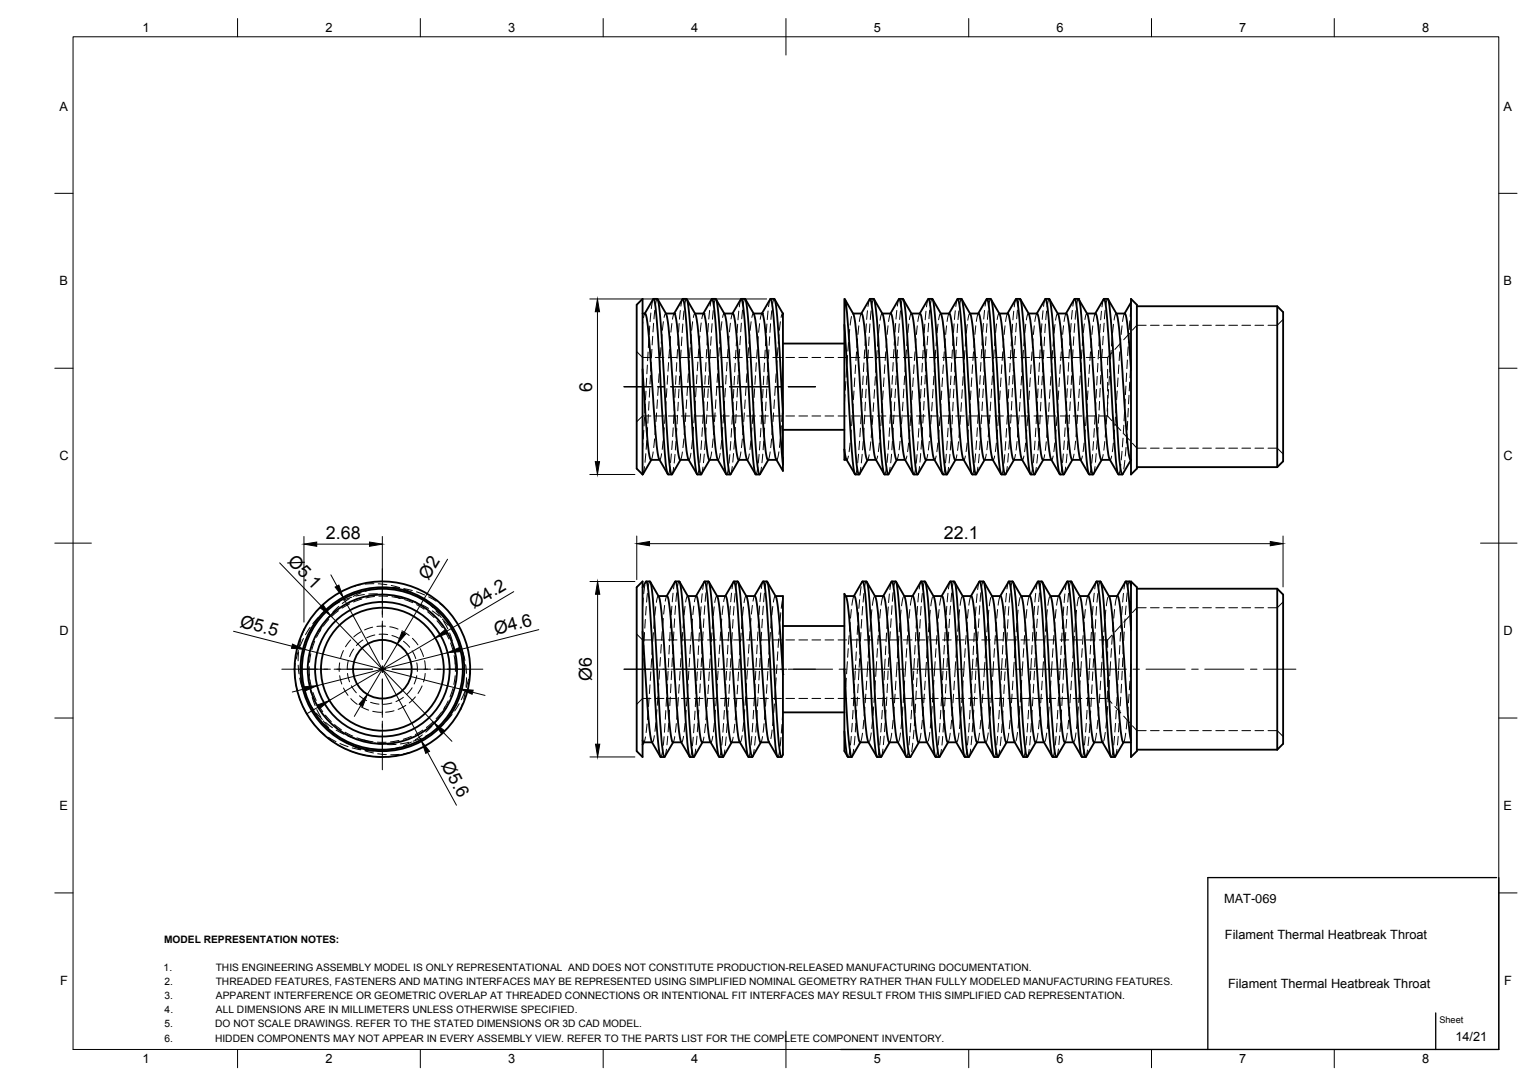
ISO-10303-21;
HEADER;
/* Generated by software containing ST-Developer
 * from STEP Tools, Inc. (www.steptools.com) 
 */

FILE_DESCRIPTION(
/* description */ ('CAx-IF Rec.Pracs.---Representation and Presentation of Product Manufa
cturing Information (PMI)---4.0---2014-10-13'),
/* implementation_level */ '2;1');

FILE_NAME(
/* name */ 'Filament Thermal Heatbreak Throat.step',
/* time_stamp */ '2026-10-24T15:08:39-07:00',
/* author */ (''),
/* organization */ (''),
/* preprocessor_version */ 'ST-DEVELOPER v20.2',
/* originating_system */ 'Autodesk Translation Framework v15.17.0.0',
/* authorisation */ '');

FILE_SCHEMA (('AP242_MANAGED_MODEL_BASED_3D_ENGINEERING_MIM_LF { 1 0 10303 442 2 1 4 }'));
ENDSEC;

DATA;
#10=MECHANICAL_DESIGN_GEOMETRIC_PRESENTATION_REPRESENTATION('',(#831),#50081);
#106=B_SPLINE_SURFACE_WITH_KNOTS('',3,3,((#39360,#39361,#39362,#39363,#39364,
#39365,#39366,#39367,#39368,#39369,#39370,#39371,#39372,#39373,#39374,#39375,
#39376,#39377,#39378,#39379,#39380,#39381,#39382,#39383,#39384,#39385,#39386,
#39387,#39388,#39389,#39390,#39391,#39392,#39393,#39394,#39395,#39396,#39397,
#39398,#39399,#39400,#39401,#39402,#39403,#39404,#39405,#39406,#39407,#39408,
#39409,#39410,#39411,#39412,#39413,#39414,#39415,#39416,#39417,#39418,#39419,
#39420,#39421,#39422,#39423,#39424,#39425,#39426),(#39427,#39428,#39429,
#39430,#39431,#39432,#39433,#39434,#39435,#39436,#39437,#39438,#39439,#39440,
#39441,#39442,#39443,#39444,#39445,#39446,#39447,#39448,#39449,#39450,#39451,
#39452,#39453,#39454,#39455,#39456,#39457,#39458,#39459,#39460,#39461,#39462,
#39463,#39464,#39465,#39466,#39467,#39468,#39469,#39470,#39471,#39472,#39473,
#39474,#39475,#39476,#39477,#39478,#39479,#39480,#39481,#39482,#39483,#39484,
#39485,#39486,#39487,#39488,#39489,#39490,#39491,#39492,#39493),(#39494,
#39495,#39496,#39497,#39498,#39499,#39500,#39501,#39502,#39503,#39504,#39505,
#39506,#39507,#39508,#39509,#39510,#39511,#39512,#39513,#39514,#39515,#39516,
#39517,#39518,#39519,#39520,#39521,#39522,#39523,#39524,#39525,#39526,#39527,
#39528,#39529,#39530,#39531,#39532,#39533,#39534,#39535,#39536,#39537,#39538,
#39539,#39540,#39541,#39542,#39543,#39544,#39545,#39546,#39547,#39548,#39549,
#39550,#39551,#39552,#39553,#39554,#39555,#39556,#39557,#39558,#39559,#39560),
(#39561,#39562,#39563,#39564,#39565,#39566,#39567,#39568,#39569,#39570,
#39571,#39572,#39573,#39574,#39575,#39576,#39577,#39578,#39579,#39580,#39581,
#39582,#39583,#39584,#39585,#39586,#39587,#39588,#39589,#39590,#39591,#39592,
#39593,#39594,#39595,#39596,#39597,#39598,#39599,#39600,#39601,#39602,#39603,
#39604,#39605,#39606,#39607,#39608,#39609,#39610,#39611,#39612,#39613,#39614,
#39615,#39616,#39617,#39618,#39619,#39620,#39621,#39622,#39623,#39624,#39625,
#39626,#39627)),.UNSPECIFIED.,.F.,.F.,.F.,(4,4),(4,1,1,1,1,1,1,1,1,1,1,
1,1,1,1,1,1,1,1,1,1,1,1,1,1,1,1,1,1,1,1,1,1,1,1,1,1,1,1,1,1,1,1,1,1,1,1,
1,1,1,1,1,1,1,1,1,1,1,1,1,1,1,1,1,4),(-0.000386239467008404,0.0586069165862638),
(7.06837814145609,8.05903683580502,9.04949020103305,10.0399435662611,11.0303969314891,
12.0208502967171,13.0113036619452,14.0017570271732,14.9922103924013,15.9826637576293,
16.9731171228573,17.9635704880854,18.9540238533134,19.9444772185414,20.9349305837695,
21.9253839489975,22.9158373142255,23.9062906794536,24.8967440446816,25.8871974099096,
26.8776507751377,27.8681041403657,28.8585575055937,29.8490108708218,30.8394642360498,
31.8299176012778,32.8203709665059,33.8108243317339,34.8012776969619,35.79173106219,
36.782184427418,37.772637792646,38.7630911578741,39.7535445231021,40.7439978883301,
41.7344512535582,42.7249046187862,43.7153579840142,44.7058113492423,45.6962647144703,
46.6867180796983,47.6771714449264,48.6676248101544,49.6580781753824,50.6485315406105,
51.6389849058385,52.6294382710665,53.6198916362946,54.6103450015226,55.6007983667506,
56.5912517319787,57.5817050972067,58.5721584624347,59.5626118276628,60.5530651928908,
61.5435185581188,62.5339719233469,63.5244252885749,64.5148786538029,65.505332019031,
66.495785384259,67.486238749487,68.4766921147151,69.4671454799431,70.4577594577278),
 .UNSPECIFIED.);
#107=B_SPLINE_SURFACE_WITH_KNOTS('',3,3,((#39674,#39675,#39676,#39677,#39678,
#39679,#39680,#39681,#39682,#39683,#39684,#39685,#39686,#39687,#39688,#39689,
#39690,#39691,#39692,#39693,#39694,#39695,#39696,#39697,#39698,#39699,#39700,
#39701,#39702,#39703,#39704,#39705,#39706,#39707,#39708,#39709,#39710,#39711,
#39712,#39713,#39714,#39715,#39716,#39717,#39718,#39719,#39720,#39721,#39722,
#39723,#39724,#39725,#39726,#39727,#39728,#39729,#39730,#39731,#39732,#39733,
#39734,#39735,#39736,#39737,#39738,#39739,#39740),(#39741,#39742,#39743,
#39744,#39745,#39746,#39747,#39748,#39749,#39750,#39751,#39752,#39753,#39754,
#39755,#39756,#39757,#39758,#39759,#39760,#39761,#39762,#39763,#39764,#39765,
#39766,#39767,#39768,#39769,#39770,#39771,#39772,#39773,#39774,#39775,#39776,
#39777,#39778,#39779,#39780,#39781,#39782,#39783,#39784,#39785,#39786,#39787,
#39788,#39789,#39790,#39791,#39792,#39793,#39794,#39795,#39796,#39797,#39798,
#39799,#39800,#39801,#39802,#39803,#39804,#39805,#39806,#39807),(#39808,
#39809,#39810,#39811,#39812,#39813,#39814,#39815,#39816,#39817,#39818,#39819,
#39820,#39821,#39822,#39823,#39824,#39825,#39826,#39827,#39828,#39829,#39830,
#39831,#39832,#39833,#39834,#39835,#39836,#39837,#39838,#39839,#39840,#39841,
#39842,#39843,#39844,#39845,#39846,#39847,#39848,#39849,#39850,#39851,#39852,
#39853,#39854,#39855,#39856,#39857,#39858,#39859,#39860,#39861,#39862,#39863,
#39864,#39865,#39866,#39867,#39868,#39869,#39870,#39871,#39872,#39873,#39874),
(#39875,#39876,#39877,#39878,#39879,#39880,#39881,#39882,#39883,#39884,
#39885,#39886,#39887,#39888,#39889,#39890,#39891,#39892,#39893,#39894,#39895,
#39896,#39897,#39898,#39899,#39900,#39901,#39902,#39903,#39904,#39905,#39906,
#39907,#39908,#39909,#39910,#39911,#39912,#39913,#39914,#39915,#39916,#39917,
#39918,#39919,#39920,#39921,#39922,#39923,#39924,#39925,#39926,#39927,#39928,
#39929,#39930,#39931,#39932,#39933,#39934,#39935,#39936,#39937,#39938,#39939,
#39940,#39941)),.UNSPECIFIED.,.F.,.F.,.F.,(4,4),(4,1,1,1,1,1,1,1,1,1,1,
1,1,1,1,1,1,1,1,1,1,1,1,1,1,1,1,1,1,1,1,1,1,1,1,1,1,1,1,1,1,1,1,1,1,1,1,
1,1,1,1,1,1,1,1,1,1,1,1,1,1,1,1,1,4),(-0.00577350269189626,0.0581188424251775),
(10.7523816656495,11.7430246153529,12.733477980581,13.723931345809,14.714384711037,
15.7048380762651,16.6952914414931,17.6857448067211,18.6761981719492,19.6666515371772,
20.6571049024052,21.6475582676333,22.6380116328613,23.6284649980893,24.6189183633174,
25.6093717285454,26.5998250937734,27.5902784590015,28.5807318242295,29.5711851894575,
30.5616385546856,31.5520919199136,32.5425452851416,33.5329986503697,34.5234520155977,
35.5139053808257,36.5043587460538,37.4948121112818,38.4852654765099,39.4757188417379,
40.4661722069659,41.4566255721939,42.447078937422,43.43753230265,44.4279856678781,
45.4184390331061,46.4088923983341,47.3993457635622,48.3897991287902,49.3802524940182,
50.3707058592463,51.3611592244743,52.3516125897023,53.3420659549304,54.3325193201584,
55.3229726853864,56.3134260506145,57.3038794158425,58.2943327810705,59.2847861462986,
60.2752395115266,61.2656928767546,62.2561462419827,63.2465996072107,64.2370529724387,
65.2275063376668,66.2179597028948,67.2084130681228,68.1988664333509,69.1893197985789,
70.1797731638069,71.170226529035,72.160679894263,73.151133259491,74.1417901888294),
 .UNSPECIFIED.);
#108=B_SPLINE_SURFACE_WITH_KNOTS('',3,3,((#40005,#40006,#40007,#40008,#40009,
#40010,#40011,#40012,#40013,#40014,#40015,#40016,#40017,#40018,#40019,#40020,
#40021,#40022,#40023,#40024,#40025,#40026,#40027,#40028,#40029,#40030,#40031,
#40032,#40033,#40034,#40035,#40036,#40037,#40038,#40039),(#40040,#40041,
#40042,#40043,#40044,#40045,#40046,#40047,#40048,#40049,#40050,#40051,#40052,
#40053,#40054,#40055,#40056,#40057,#40058,#40059,#40060,#40061,#40062,#40063,
#40064,#40065,#40066,#40067,#40068,#40069,#40070,#40071,#40072,#40073,#40074),
(#40075,#40076,#40077,#40078,#40079,#40080,#40081,#40082,#40083,#40084,
#40085,#40086,#40087,#40088,#40089,#40090,#40091,#40092,#40093,#40094,#40095,
#40096,#40097,#40098,#40099,#40100,#40101,#40102,#40103,#40104,#40105,#40106,
#40107,#40108,#40109),(#40110,#40111,#40112,#40113,#40114,#40115,#40116,
#40117,#40118,#40119,#40120,#40121,#40122,#40123,#40124,#40125,#40126,#40127,
#40128,#40129,#40130,#40131,#40132,#40133,#40134,#40135,#40136,#40137,#40138,
#40139,#40140,#40141,#40142,#40143,#40144)),.UNSPECIFIED.,.F.,.F.,.F.,(4,
4),(4,1,1,1,1,1,1,1,1,1,1,1,1,1,1,1,1,1,1,1,1,1,1,1,1,1,1,1,1,1,1,1,4),
(-0.000393287427394601,0.0585773552985969),(7.06836282084679,8.0677424967863,
9.06690152299556,10.0660605492048,11.0652195754141,12.0643786016233,13.0635376278326,
14.0626966540418,15.0618556802511,16.0610147064604,17.0601737326696,18.0593327588789,
19.0584917850881,20.0576508112974,21.0568098375066,22.0559688637159,23.0551278899252,
24.0542869161344,25.0534459423437,26.0526049685529,27.0517639947622,28.0509230209714,
29.0500820471807,30.04924107339,31.0484000995992,32.0475591258085,33.0467181520177,
34.045877178227,35.0450362044363,36.0441952306455,37.0433542568548,38.042513283064,
39.0418309313306),.UNSPECIFIED.);
#109=B_SPLINE_SURFACE_WITH_KNOTS('',3,3,((#40284,#40285,#40286,#40287,#40288,
#40289,#40290,#40291,#40292,#40293,#40294,#40295,#40296,#40297,#40298,#40299,
#40300,#40301,#40302,#40303,#40304,#40305,#40306,#40307,#40308,#40309,#40310,
#40311,#40312,#40313,#40314,#40315,#40316,#40317,#40318),(#40319,#40320,
#40321,#40322,#40323,#40324,#40325,#40326,#40327,#40328,#40329,#40330,#40331,
#40332,#40333,#40334,#40335,#40336,#40337,#40338,#40339,#40340,#40341,#40342,
#40343,#40344,#40345,#40346,#40347,#40348,#40349,#40350,#40351,#40352,#40353),
(#40354,#40355,#40356,#40357,#40358,#40359,#40360,#40361,#40362,#40363,
#40364,#40365,#40366,#40367,#40368,#40369,#40370,#40371,#40372,#40373,#40374,
#40375,#40376,#40377,#40378,#40379,#40380,#40381,#40382,#40383,#40384,#40385,
#40386,#40387,#40388),(#40389,#40390,#40391,#40392,#40393,#40394,#40395,
#40396,#40397,#40398,#40399,#40400,#40401,#40402,#40403,#40404,#40405,#40406,
#40407,#40408,#40409,#40410,#40411,#40412,#40413,#40414,#40415,#40416,#40417,
#40418,#40419,#40420,#40421,#40422,#40423)),.UNSPECIFIED.,.F.,.F.,.F.,(4,
4),(4,1,1,1,1,1,1,1,1,1,1,1,1,1,1,1,1,1,1,1,1,1,1,1,1,1,1,1,1,1,1,1,4),
(-0.000893816201826896,0.0581534486591829),(10.7523808111136,11.7517302763342,
12.7508893025435,13.7500483287527,14.749207354962,15.7483663811713,16.7475254073805,
17.7466844335898,18.745843459799,19.7450024860083,20.7441615122175,21.7433205384268,
22.742479564636,23.7416385908453,24.7407976170546,25.7399566432638,26.7391156694731,
27.7382746956823,28.7374337218916,29.7365927481009,30.7357517743101,31.7349108005194,
32.7340698267286,33.7332288529379,34.7323878791471,35.7315469053564,36.7307059315657,
37.7298649577749,38.7290239839842,39.7281830101934,40.7273420364027,41.7265010626119,
42.7258669660187),.UNSPECIFIED.);
#386=B_SPLINE_CURVE_WITH_KNOTS('',3,(#34790,#34791,#34792,#34793,#34794,
#34795,#34796,#34797,#34798,#34799,#34800,#34801,#34802,#34803,#34804,#34805,
#34806,#34807,#34808,#34809,#34810,#34811,#34812,#34813,#34814,#34815,#34816,
#34817,#34818,#34819,#34820,#34821,#34822,#34823,#34824,#34825,#34826,#34827,
#34828,#34829,#34830,#34831,#34832,#34833,#34834,#34835,#34836,#34837,#34838),
 .UNSPECIFIED.,.F.,.F.,(4,3,3,3,3,3,3,3,3,3,3,3,3,3,3,3,4),(0.,0.0927605595561279,
0.125,0.216051601199591,0.25,0.341388358155206,0.375,0.46637118185636,0.5,
0.591371181856193,0.625,0.716388358155103,0.75,0.841051601199441,0.875,
0.967760559556323,1.),.UNSPECIFIED.);
#387=B_SPLINE_CURVE_WITH_KNOTS('',3,(#34840,#34841,#34842,#34843,#34844,
#34845,#34846,#34847,#34848,#34849,#34850,#34851,#34852,#34853,#34854,#34855,
#34856,#34857,#34858,#34859,#34860,#34861,#34862,#34863,#34864,#34865,#34866,
#34867,#34868,#34869,#34870,#34871,#34872,#34873,#34874,#34875,#34876,#34877,
#34878,#34879,#34880,#34881,#34882,#34883,#34884,#34885,#34886,#34887,#34888,
#34889,#34890,#34891,#34892,#34893,#34894),.UNSPECIFIED.,.F.,.F.,(4,3,3,
3,3,3,3,3,3,3,3,3,3,3,3,3,3,3,4),(1.15710129956961E-6,0.0927580101727587,
0.125,0.215560207328814,0.25,0.343554436628594,0.375,0.4375,0.46875,0.5,
0.53125,0.5625,0.625,0.6875,0.75,0.835314126539692,0.875,0.952649745898871,
0.999999206802969),.UNSPECIFIED.);
#388=B_SPLINE_CURVE_WITH_KNOTS('',3,(#34896,#34897,#34898,#34899,#34900,
#34901,#34902,#34903,#34904,#34905,#34906,#34907,#34908,#34909,#34910,#34911,
#34912,#34913,#34914,#34915,#34916,#34917,#34918,#34919,#34920,#34921,#34922,
#34923,#34924,#34925,#34926,#34927,#34928,#34929,#34930,#34931,#34932,#34933,
#34934,#34935,#34936,#34937,#34938,#34939,#34940,#34941,#34942,#34943,#34944),
 .UNSPECIFIED.,.F.,.F.,(4,3,3,3,3,3,3,3,3,3,3,3,3,3,3,3,4),(0.,0.0927652271086669,
0.125,0.216056340442133,0.25,0.341393095875492,0.375,0.466375911195523,
0.5,0.59137591119598,0.625,0.716393095875431,0.75,0.841056340442169,0.875,
0.967765227108083,1.),.UNSPECIFIED.);
#389=B_SPLINE_CURVE_WITH_KNOTS('',3,(#34946,#34947,#34948,#34949,#34950,
#34951,#34952,#34953,#34954,#34955,#34956,#34957,#34958,#34959,#34960,#34961,
#34962,#34963,#34964,#34965,#34966,#34967,#34968,#34969,#34970,#34971,#34972,
#34973,#34974,#34975,#34976,#34977,#34978,#34979,#34980,#34981,#34982,#34983,
#34984,#34985,#34986,#34987,#34988,#34989,#34990,#34991,#34992,#34993,#34994),
 .UNSPECIFIED.,.F.,.F.,(4,3,3,3,3,3,3,3,3,3,3,3,3,3,3,3,4),(0.,0.0927588912582948,
0.125,0.216049907277145,0.25,0.34138666477614,0.375,0.466369491473306,0.5,
0.591369491472985,0.625,0.716386664776259,0.75,0.841049907277114,0.875,
0.967758891258586,1.),.UNSPECIFIED.);
#390=B_SPLINE_CURVE_WITH_KNOTS('',3,(#34996,#34997,#34998,#34999,#35000,
#35001,#35002,#35003,#35004,#35005,#35006,#35007,#35008,#35009,#35010,#35011,
#35012,#35013,#35014,#35015,#35016,#35017,#35018,#35019,#35020,#35021,#35022,
#35023,#35024,#35025,#35026,#35027,#35028,#35029,#35030,#35031,#35032,#35033,
#35034,#35035,#35036,#35037,#35038,#35039,#35040,#35041,#35042,#35043,#35044,
#35045,#35046,#35047,#35048,#35049,#35050,#35051,#35052,#35053,#35054,#35055,
#35056,#35057,#35058,#35059,#35060,#35061,#35062,#35063,#35064,#35065,#35066,
#35067,#35068,#35069,#35070,#35071),.UNSPECIFIED.,.F.,.F.,(4,3,3,3,3,3,
3,3,3,3,3,3,3,3,3,3,3,3,3,3,3,3,3,3,3,4),(1.15508471750028E-6,0.092144029884165,
0.125,0.216529255746127,0.25,0.3125,0.375,0.40625,0.4375,0.46875,0.484375,
0.4921875,0.5,0.5078125,0.515625,0.53125,0.5625,0.59375,0.625,0.6875,0.75,
0.8125,0.875,0.9375,0.995454104613646,0.999999596646375),.UNSPECIFIED.);
#391=B_SPLINE_CURVE_WITH_KNOTS('',3,(#35073,#35074,#35075,#35076,#35077,
#35078,#35079,#35080,#35081,#35082,#35083,#35084,#35085,#35086,#35087,#35088,
#35089,#35090,#35091,#35092,#35093,#35094,#35095,#35096,#35097,#35098,#35099,
#35100,#35101,#35102,#35103,#35104,#35105,#35106,#35107,#35108,#35109,#35110,
#35111,#35112,#35113,#35114,#35115,#35116,#35117,#35118,#35119,#35120,#35121),
 .UNSPECIFIED.,.F.,.F.,(4,3,3,3,3,3,3,3,3,3,3,3,3,3,3,3,4),(0.,0.0927687029302607,
0.125,0.216059869646637,0.25,0.341396623944995,0.375,0.466379433025891,
0.5,0.59137943302596,0.625,0.71639662394496,0.75,0.841059869646648,0.875,
0.967768702930745,1.),.UNSPECIFIED.);
#392=B_SPLINE_CURVE_WITH_KNOTS('',3,(#35123,#35124,#35125,#35126,#35127,
#35128,#35129,#35130,#35131,#35132,#35133,#35134,#35135,#35136,#35137,#35138,
#35139,#35140,#35141,#35142,#35143,#35144,#35145,#35146,#35147,#35148,#35149,
#35150,#35151,#35152,#35153,#35154,#35155,#35156,#35157,#35158,#35159,#35160,
#35161,#35162,#35163,#35164,#35165,#35166,#35167,#35168,#35169,#35170,#35171),
 .UNSPECIFIED.,.F.,.F.,(4,3,3,3,3,3,3,3,3,3,3,3,3,3,3,3,4),(0.,0.0927568833925016,
0.125,0.216047868569561,0.25,0.34138462672263,0.375,0.46636745702548,0.5,
0.59136745702557,0.625,0.716384626722753,0.75,0.841047868569713,0.875,0.967756883392973,
1.),.UNSPECIFIED.);
#393=B_SPLINE_CURVE_WITH_KNOTS('',3,(#35173,#35174,#35175,#35176,#35177,
#35178,#35179,#35180,#35181,#35182,#35183,#35184,#35185,#35186,#35187,#35188,
#35189,#35190,#35191,#35192,#35193,#35194,#35195,#35196,#35197,#35198,#35199,
#35200,#35201,#35202,#35203,#35204,#35205,#35206,#35207,#35208,#35209,#35210,
#35211,#35212,#35213,#35214,#35215,#35216,#35217,#35218,#35219,#35220,#35221),
 .UNSPECIFIED.,.F.,.F.,(4,3,3,3,3,3,3,3,3,3,3,3,3,3,3,3,4),(1.00511200959296E-6,
0.0927437682042961,0.125,0.216035219771111,0.25,0.341376986124011,0.375,
0.466313829040159,0.5,0.591406458509517,0.625,0.716377484365712,0.75,0.841045743313971,
0.875,0.967756443545387,0.99999978647056),.UNSPECIFIED.);
#394=B_SPLINE_CURVE_WITH_KNOTS('',3,(#35223,#35224,#35225,#35226,#35227,
#35228,#35229,#35230,#35231,#35232,#35233,#35234,#35235,#35236,#35237,#35238,
#35239,#35240,#35241,#35242,#35243,#35244,#35245,#35246,#35247,#35248,#35249,
#35250,#35251,#35252,#35253,#35254,#35255,#35256,#35257,#35258,#35259,#35260,
#35261,#35262,#35263,#35264,#35265,#35266,#35267,#35268,#35269,#35270,#35271),
 .UNSPECIFIED.,.F.,.F.,(4,3,3,3,3,3,3,3,3,3,3,3,3,3,3,3,4),(0.,0.0927720508247614,
0.125,0.216063268956037,0.25,0.341400022160318,0.375,0.466382825231913,
0.5,0.591382825232266,0.625,0.716400022160194,0.75,0.841063268956108,0.875,
0.967772050824302,1.),.UNSPECIFIED.);
#395=B_SPLINE_CURVE_WITH_KNOTS('',3,(#35277,#35278,#35279,#35280,#35281,
#35282,#35283,#35284,#35285,#35286,#35287,#35288,#35289,#35290,#35291,#35292,
#35293,#35294,#35295,#35296,#35297,#35298,#35299,#35300,#35301),
 .UNSPECIFIED.,.F.,.F.,(4,3,3,3,3,3,3,3,4),(0.,0.125,0.25,0.375,0.5,0.625,
0.75,0.875,0.999999474719706),.UNSPECIFIED.);
#396=B_SPLINE_CURVE_WITH_KNOTS('',3,(#35303,#35304,#35305,#35306,#35307,
#35308,#35309,#35310,#35311,#35312,#35313,#35314,#35315,#35316,#35317,#35318,
#35319,#35320,#35321,#35322,#35323,#35324,#35325,#35326,#35327,#35328,#35329,
#35330,#35331,#35332,#35333,#35334,#35335,#35336,#35337,#35338,#35339,#35340,
#35341,#35342,#35343,#35344,#35345,#35346,#35347,#35348,#35349,#35350,#35351),
 .UNSPECIFIED.,.F.,.F.,(4,3,3,3,3,3,3,3,3,3,3,3,3,3,3,3,4),(0.,0.092751628903762,
0.125,0.216042533365587,0.25,0.341379293228406,0.375,0.466362132969287,
0.5,0.591362132969264,0.625,0.716379293228501,0.75,0.841042533365549,0.875,
0.967751628903877,1.),.UNSPECIFIED.);
#397=B_SPLINE_CURVE_WITH_KNOTS('',3,(#35353,#35354,#35355,#35356,#35357,
#35358,#35359,#35360,#35361,#35362,#35363,#35364,#35365,#35366,#35367,#35368,
#35369,#35370,#35371,#35372,#35373,#35374,#35375,#35376,#35377,#35378,#35379,
#35380,#35381,#35382,#35383,#35384,#35385,#35386,#35387,#35388,#35389,#35390,
#35391,#35392,#35393,#35394,#35395,#35396,#35397,#35398,#35399,#35400,#35401),
 .UNSPECIFIED.,.F.,.F.,(4,3,3,3,3,3,3,3,3,3,3,3,3,3,3,3,4),(0.,0.0927733010189759,
0.125,0.216064538349619,0.25,0.341401291145062,0.375,0.4663840919732,0.5,
0.591384091973165,0.625,0.716401291144964,0.75,0.841064538349631,0.875,
0.967773301019603,1.),.UNSPECIFIED.);
#398=B_SPLINE_CURVE_WITH_KNOTS('',3,(#35403,#35404,#35405,#35406,#35407,
#35408,#35409,#35410,#35411,#35412,#35413,#35414,#35415,#35416,#35417,#35418,
#35419,#35420,#35421,#35422,#35423,#35424,#35425,#35426,#35427,#35428,#35429,
#35430,#35431,#35432,#35433,#35434,#35435,#35436,#35437,#35438,#35439,#35440,
#35441,#35442,#35443,#35444,#35445,#35446,#35447,#35448,#35449,#35450,#35451,
#35452,#35453,#35454),.UNSPECIFIED.,.F.,.F.,(4,2,2,2,2,2,2,2,2,2,2,2,2,
2,2,2,2,2,2,2,2,2,2,2,2,4),(0.,0.0553130156040213,0.0625,0.125,0.1875,0.25,
0.3125,0.375,0.40625,0.4375,0.46875,0.484375,0.4921875,0.5,0.5078125,0.515625,
0.53125,0.5625,0.59375,0.625,0.6875,0.75,0.841517211022419,0.875,0.967130863494855,
0.999999278904145),.UNSPECIFIED.);
#399=B_SPLINE_CURVE_WITH_KNOTS('',3,(#35456,#35457,#35458,#35459,#35460,
#35461,#35462,#35463,#35464,#35465,#35466,#35467,#35468,#35469,#35470,#35471,
#35472,#35473,#35474,#35475,#35476,#35477,#35478,#35479,#35480,#35481,#35482,
#35483,#35484,#35485,#35486,#35487,#35488,#35489,#35490,#35491,#35492,#35493,
#35494,#35495,#35496,#35497,#35498,#35499,#35500,#35501,#35502,#35503,#35504),
 .UNSPECIFIED.,.F.,.F.,(4,3,3,3,3,3,3,3,3,3,3,3,3,3,3,3,4),(0.,0.092754553141066,
0.125,0.21604550252371,0.25,0.341382261435592,0.375,0.466365095923449,0.5,
0.591365095923193,0.625,0.716382261435363,0.75,0.841045502523726,0.875,
0.96775455314112,1.),.UNSPECIFIED.);
#400=B_SPLINE_CURVE_WITH_KNOTS('',3,(#35506,#35507,#35508,#35509,#35510,
#35511,#35512,#35513,#35514,#35515,#35516,#35517,#35518,#35519,#35520,#35521,
#35522,#35523,#35524,#35525,#35526,#35527,#35528,#35529,#35530,#35531,#35532,
#35533,#35534,#35535,#35536,#35537,#35538,#35539,#35540,#35541,#35542,#35543,
#35544,#35545,#35546,#35547,#35548,#35549,#35550,#35551,#35552,#35553,#35554),
 .UNSPECIFIED.,.F.,.F.,(4,3,3,3,3,3,3,3,3,3,3,3,3,3,3,3,4),(0.,0.0927714769858617,
0.125,0.216062686304942,0.25,0.341399439696681,0.375,0.466382243798817,
0.5,0.591382243798365,0.625,0.716399439696732,0.75,0.841062686305149,0.875,
0.967771476985755,1.),.UNSPECIFIED.);
#401=B_SPLINE_CURVE_WITH_KNOTS('',3,(#35556,#35557,#35558,#35559,#35560,
#35561,#35562,#35563,#35564,#35565,#35566,#35567,#35568,#35569,#35570,#35571,
#35572,#35573,#35574,#35575,#35576,#35577,#35578,#35579,#35580,#35581,#35582,
#35583,#35584,#35585,#35586,#35587,#35588,#35589,#35590,#35591,#35592,#35593,
#35594,#35595,#35596,#35597,#35598,#35599,#35600,#35601,#35602,#35603,#35604,
#35605,#35606,#35607,#35608,#35609,#35610,#35611,#35612,#35613,#35614,#35615,
#35616,#35617,#35618,#35619,#35620,#35621,#35622,#35623,#35624,#35625,#35626,
#35627,#35628,#35629,#35630,#35631,#35632,#35633,#35634,#35635,#35636,#35637,
#35638,#35639,#35640,#35641,#35642,#35643),.UNSPECIFIED.,.F.,.F.,(4,3,3,
3,3,3,3,3,3,3,3,3,3,3,3,3,3,3,3,3,3,3,3,3,3,3,3,3,3,4),(1.05714741198223E-7,
0.0471016803099375,0.0625,0.114776485281687,0.125,0.183175405287037,0.1875,
0.25,0.3125,0.375,0.40625,0.4375,0.453125,0.46875,0.484375,0.4921875,0.5,
0.5078125,0.515625,0.53125,0.546875,0.5625,0.59375,0.625,0.6875,0.75,0.8125,
0.875,0.968959747574043,0.999999002444466),.UNSPECIFIED.);
#402=B_SPLINE_CURVE_WITH_KNOTS('',3,(#35645,#35646,#35647,#35648,#35649,
#35650,#35651,#35652,#35653,#35654,#35655,#35656,#35657,#35658,#35659,#35660,
#35661,#35662,#35663,#35664,#35665,#35666,#35667,#35668,#35669,#35670,#35671,
#35672,#35673,#35674,#35675,#35676,#35677,#35678,#35679,#35680,#35681,#35682,
#35683,#35684,#35685,#35686,#35687,#35688,#35689,#35690,#35691,#35692,#35693),
 .UNSPECIFIED.,.F.,.F.,(4,3,3,3,3,3,3,3,3,3,3,3,3,3,3,3,4),(0.,0.0927568305050716,
0.125,0.216047814869766,0.25,0.341384573040307,0.375,0.466367403437729,
0.5,0.591367403437667,0.625,0.716384573040161,0.75,0.841047814869804,0.875,
0.967756830505404,1.),.UNSPECIFIED.);
#403=B_SPLINE_CURVE_WITH_KNOTS('',3,(#35695,#35696,#35697,#35698,#35699,
#35700,#35701,#35702,#35703,#35704,#35705,#35706,#35707,#35708,#35709,#35710,
#35711,#35712,#35713,#35714,#35715,#35716,#35717,#35718,#35719,#35720,#35721,
#35722,#35723,#35724,#35725,#35726,#35727,#35728,#35729,#35730,#35731,#35732,
#35733,#35734,#35735,#35736,#35737,#35738,#35739,#35740,#35741,#35742,#35743),
 .UNSPECIFIED.,.F.,.F.,(4,3,3,3,3,3,3,3,3,3,3,3,3,3,3,3,4),(0.,0.0927687785918848,
0.125,0.21605994647008,0.25,0.341396700743647,0.375,0.466379509688856,0.5,
0.591379509688596,0.625,0.716396700743673,0.75,0.841059946470065,0.875,
0.967768778592018,1.),.UNSPECIFIED.);
#404=B_SPLINE_CURVE_WITH_KNOTS('',3,(#35745,#35746,#35747,#35748,#35749,
#35750,#35751,#35752,#35753,#35754,#35755,#35756,#35757,#35758,#35759,#35760,
#35761,#35762,#35763,#35764,#35765,#35766,#35767,#35768,#35769,#35770,#35771,
#35772,#35773,#35774,#35775,#35776,#35777,#35778),.UNSPECIFIED.,.F.,.F.,
(4,2,2,2,2,2,2,2,2,2,2,2,2,2,2,2,4),(6.2904793357381E-7,0.092754167897614,
0.125,0.216044766897767,0.25,0.341379705506234,0.375,0.466367644770845,
0.5,0.591380776467673,0.625,0.716346028360352,0.75,0.841038184239321,0.875,
0.967744550610455,0.999998988396429),.UNSPECIFIED.);
#405=B_SPLINE_CURVE_WITH_KNOTS('',3,(#35780,#35781,#35782,#35783),
 .UNSPECIFIED.,.F.,.F.,(4,4),(0.,0.999999235891784),.UNSPECIFIED.);
#406=B_SPLINE_CURVE_WITH_KNOTS('',3,(#35786,#35787,#35788,#35789,#35790,
#35791,#35792,#35793,#35794,#35795,#35796,#35797,#35798,#35799,#35800,#35801,
#35802,#35803,#35804,#35805,#35806,#35807,#35808,#35809,#35810,#35811,#35812,
#35813,#35814,#35815,#35816,#35817,#35818,#35819,#35820,#35821,#35822,#35823,
#35824,#35825,#35826,#35827,#35828,#35829,#35830,#35831,#35832,#35833,#35834),
 .UNSPECIFIED.,.F.,.F.,(4,3,3,3,3,3,3,3,3,3,3,3,3,3,3,3,4),(5.35367963709457E-13,
0.11846007821872,0.125,0.242079186084241,0.25,0.367390321915038,0.375,0.492346917375386,
0.5,0.617346917375406,0.625,0.742390321915024,0.75,0.86707918608421,0.875,
0.993460078218313,1.),.UNSPECIFIED.);
#407=B_SPLINE_CURVE_WITH_KNOTS('',3,(#35838,#35839,#35840,#35841,#35842,
#35843,#35844,#35845,#35846,#35847,#35848,#35849,#35850,#35851,#35852,#35853,
#35854,#35855,#35856,#35857,#35858,#35859,#35860,#35861,#35862,#35863,#35864,
#35865,#35866,#35867,#35868,#35869,#35870,#35871,#35872,#35873,#35874,#35875,
#35876,#35877,#35878,#35879,#35880,#35881,#35882,#35883,#35884,#35885,#35886),
 .UNSPECIFIED.,.F.,.F.,(4,3,3,3,3,3,3,3,3,3,3,3,3,3,3,3,4),(0.500496609805673,
0.50390625,0.5078125,0.515625,0.53125,0.546875,0.5625,0.591671105840508,
0.59375,0.625,0.6875,0.749287235495431,0.75,0.8125,0.875,0.907000590990823,
0.999998995230263),.UNSPECIFIED.);
#408=B_SPLINE_CURVE_WITH_KNOTS('',3,(#35888,#35889,#35890,#35891,#35892,
#35893,#35894,#35895,#35896,#35897,#35898,#35899,#35900,#35901,#35902,#35903,
#35904,#35905,#35906,#35907,#35908,#35909,#35910,#35911,#35912,#35913,#35914,
#35915,#35916,#35917,#35918,#35919,#35920,#35921,#35922,#35923,#35924,#35925,
#35926,#35927,#35928,#35929,#35930,#35931,#35932,#35933,#35934,#35935,#35936,
#35937,#35938,#35939,#35940,#35941,#35942,#35943,#35944,#35945,#35946,#35947,
#35948,#35949,#35950,#35951,#35952,#35953,#35954,#35955,#35956,#35957,#35958,
#35959,#35960,#35961,#35962,#35963,#35964,#35965,#35966,#35967,#35968,#35969,
#35970,#35971,#35972,#35973,#35974,#35975,#35976,#35977,#35978,#35979,#35980,
#35981,#35982,#35983,#35984,#35985,#35986,#35987,#35988,#35989,#35990,#35991,
#35992,#35993,#35994,#35995,#35996,#35997,#35998,#35999,#36000,#36001,#36002,
#36003,#36004,#36005,#36006,#36007,#36008,#36009,#36010,#36011,#36012,#36013,
#36014,#36015,#36016,#36017,#36018,#36019,#36020,#36021,#36022,#36023,#36024,
#36025,#36026,#36027,#36028,#36029,#36030,#36031,#36032,#36033,#36034,#36035,
#36036,#36037,#36038,#36039,#36040,#36041,#36042,#36043,#36044,#36045,#36046,
#36047,#36048,#36049,#36050,#36051,#36052,#36053,#36054,#36055,#36056,#36057,
#36058,#36059,#36060,#36061,#36062,#36063,#36064,#36065,#36066,#36067,#36068,
#36069,#36070,#36071,#36072,#36073,#36074,#36075,#36076,#36077,#36078,#36079,
#36080,#36081,#36082,#36083,#36084,#36085,#36086,#36087,#36088,#36089,#36090,
#36091,#36092,#36093,#36094,#36095,#36096,#36097,#36098,#36099,#36100,#36101,
#36102,#36103,#36104,#36105,#36106,#36107,#36108,#36109,#36110,#36111,#36112,
#36113,#36114,#36115,#36116,#36117,#36118,#36119,#36120,#36121,#36122,#36123,
#36124,#36125,#36126,#36127,#36128,#36129,#36130,#36131,#36132,#36133,#36134,
#36135,#36136,#36137,#36138,#36139,#36140,#36141,#36142,#36143,#36144,#36145,
#36146,#36147,#36148,#36149,#36150,#36151,#36152,#36153,#36154,#36155,#36156,
#36157,#36158,#36159,#36160,#36161,#36162,#36163,#36164,#36165,#36166,#36167,
#36168,#36169,#36170,#36171,#36172,#36173,#36174,#36175,#36176,#36177,#36178,
#36179,#36180,#36181,#36182,#36183,#36184,#36185,#36186,#36187,#36188,#36189,
#36190,#36191,#36192,#36193,#36194,#36195,#36196,#36197,#36198,#36199,#36200,
#36201,#36202,#36203,#36204,#36205,#36206,#36207,#36208,#36209,#36210,#36211,
#36212,#36213,#36214,#36215,#36216,#36217,#36218,#36219,#36220,#36221,#36222,
#36223,#36224,#36225,#36226,#36227,#36228,#36229,#36230,#36231,#36232,#36233,
#36234,#36235,#36236,#36237,#36238,#36239,#36240,#36241,#36242,#36243,#36244,
#36245,#36246,#36247,#36248,#36249,#36250,#36251,#36252,#36253,#36254,#36255,
#36256,#36257,#36258,#36259,#36260,#36261,#36262,#36263,#36264,#36265,#36266,
#36267,#36268,#36269,#36270,#36271,#36272,#36273,#36274,#36275,#36276,#36277,
#36278,#36279,#36280,#36281,#36282,#36283,#36284,#36285,#36286,#36287,#36288,
#36289,#36290,#36291,#36292,#36293,#36294,#36295,#36296,#36297,#36298,#36299,
#36300,#36301,#36302,#36303,#36304,#36305,#36306,#36307,#36308,#36309,#36310,
#36311,#36312,#36313,#36314,#36315,#36316,#36317,#36318,#36319,#36320,#36321,
#36322,#36323,#36324,#36325,#36326,#36327,#36328,#36329,#36330,#36331,#36332,
#36333,#36334,#36335,#36336,#36337,#36338,#36339,#36340,#36341,#36342,#36343,
#36344,#36345,#36346,#36347,#36348,#36349,#36350,#36351,#36352,#36353,#36354,
#36355,#36356,#36357,#36358,#36359,#36360,#36361,#36362,#36363,#36364,#36365,
#36366,#36367,#36368,#36369,#36370,#36371,#36372,#36373,#36374,#36375,#36376,
#36377,#36378,#36379,#36380,#36381,#36382,#36383,#36384,#36385,#36386,#36387,
#36388,#36389,#36390,#36391,#36392,#36393,#36394,#36395,#36396,#36397,#36398,
#36399,#36400,#36401,#36402,#36403,#36404,#36405,#36406,#36407,#36408,#36409,
#36410,#36411,#36412,#36413,#36414,#36415,#36416,#36417,#36418,#36419,#36420,
#36421,#36422,#36423,#36424,#36425,#36426,#36427,#36428,#36429,#36430,#36431,
#36432,#36433,#36434,#36435,#36436,#36437,#36438,#36439,#36440,#36441,#36442,
#36443,#36444,#36445,#36446,#36447,#36448,#36449,#36450,#36451,#36452,#36453,
#36454,#36455,#36456,#36457,#36458,#36459,#36460,#36461,#36462,#36463,#36464,
#36465,#36466,#36467,#36468,#36469,#36470,#36471,#36472,#36473,#36474,#36475,
#36476,#36477,#36478,#36479,#36480,#36481,#36482,#36483,#36484,#36485,#36486,
#36487,#36488,#36489,#36490,#36491,#36492,#36493,#36494,#36495,#36496,#36497,
#36498,#36499,#36500,#36501,#36502,#36503,#36504,#36505,#36506,#36507,#36508,
#36509,#36510,#36511,#36512,#36513,#36514,#36515,#36516,#36517,#36518,#36519,
#36520,#36521,#36522,#36523,#36524,#36525,#36526,#36527,#36528,#36529,#36530,
#36531,#36532,#36533,#36534,#36535,#36536,#36537,#36538,#36539,#36540,#36541,
#36542,#36543,#36544,#36545,#36546,#36547,#36548,#36549,#36550,#36551,#36552,
#36553,#36554,#36555,#36556,#36557,#36558,#36559,#36560,#36561,#36562,#36563,
#36564,#36565,#36566,#36567,#36568,#36569,#36570,#36571,#36572,#36573,#36574,
#36575,#36576,#36577,#36578,#36579,#36580,#36581,#36582,#36583,#36584,#36585,
#36586,#36587,#36588,#36589,#36590,#36591,#36592,#36593,#36594,#36595,#36596,
#36597,#36598,#36599,#36600,#36601,#36602,#36603,#36604,#36605,#36606,#36607,
#36608,#36609,#36610,#36611,#36612,#36613,#36614,#36615,#36616,#36617,#36618,
#36619,#36620,#36621,#36622,#36623,#36624,#36625,#36626,#36627,#36628,#36629,
#36630,#36631,#36632,#36633,#36634,#36635,#36636,#36637,#36638,#36639,#36640,
#36641,#36642,#36643,#36644,#36645,#36646,#36647,#36648,#36649,#36650,#36651,
#36652,#36653,#36654,#36655,#36656,#36657,#36658,#36659,#36660,#36661,#36662,
#36663,#36664,#36665,#36666,#36667,#36668,#36669,#36670,#36671,#36672,#36673,
#36674,#36675,#36676,#36677,#36678,#36679,#36680,#36681,#36682,#36683,#36684,
#36685,#36686,#36687,#36688,#36689,#36690,#36691,#36692,#36693,#36694,#36695,
#36696,#36697,#36698,#36699,#36700,#36701,#36702,#36703,#36704,#36705,#36706,
#36707,#36708,#36709,#36710,#36711,#36712,#36713,#36714,#36715,#36716,#36717,
#36718,#36719,#36720,#36721,#36722,#36723,#36724,#36725,#36726,#36727,#36728,
#36729,#36730,#36731,#36732,#36733,#36734,#36735,#36736,#36737,#36738,#36739,
#36740,#36741,#36742,#36743,#36744,#36745,#36746,#36747,#36748,#36749,#36750,
#36751,#36752,#36753,#36754,#36755,#36756,#36757,#36758,#36759,#36760,#36761,
#36762,#36763,#36764,#36765,#36766,#36767,#36768,#36769,#36770,#36771,#36772,
#36773,#36774,#36775,#36776,#36777,#36778,#36779,#36780,#36781,#36782,#36783,
#36784,#36785,#36786,#36787,#36788,#36789,#36790,#36791,#36792,#36793,#36794,
#36795,#36796,#36797,#36798,#36799,#36800,#36801,#36802,#36803,#36804,#36805,
#36806,#36807,#36808,#36809,#36810,#36811,#36812,#36813,#36814,#36815,#36816,
#36817,#36818,#36819,#36820,#36821,#36822,#36823,#36824,#36825,#36826,#36827,
#36828,#36829,#36830,#36831,#36832,#36833),.UNSPECIFIED.,.F.,.F.,(4,2,2,
2,2,2,2,2,2,2,2,2,2,2,2,2,2,2,2,2,2,2,2,2,2,2,2,2,2,2,2,2,2,2,2,2,2,2,2,
2,2,2,2,2,2,2,2,2,2,2,2,2,2,2,2,2,2,2,2,2,2,2,2,2,2,2,2,2,2,2,2,2,2,2,2,
2,2,2,2,2,2,2,2,2,2,2,2,2,2,2,2,2,2,2,2,2,2,2,2,2,2,2,2,2,2,2,2,2,2,2,2,
2,2,2,2,2,2,2,2,2,2,2,2,2,2,2,2,2,2,2,2,2,2,2,2,2,2,2,2,2,2,2,2,2,2,2,2,
2,2,2,2,2,2,2,2,2,2,2,2,2,2,2,2,2,2,2,2,2,2,2,2,2,2,2,2,2,2,2,2,2,2,2,2,
2,2,2,2,2,2,2,2,2,2,2,2,2,2,2,2,2,2,2,2,2,2,2,2,2,2,2,2,2,2,2,2,2,2,2,2,
2,2,2,2,2,2,2,2,2,2,2,2,2,2,2,2,2,2,2,2,2,2,2,2,2,2,2,2,2,2,2,2,2,2,2,2,
2,2,2,2,2,2,2,2,2,2,2,2,2,2,2,2,2,2,2,2,2,2,2,2,2,2,2,2,2,2,2,2,2,2,2,2,
2,2,2,2,2,2,2,2,2,2,2,2,2,2,2,2,2,2,2,2,2,2,2,2,2,2,2,2,2,2,2,2,2,2,2,2,
2,2,2,2,2,2,2,2,2,2,2,2,2,2,2,2,2,2,2,2,2,2,2,2,2,2,2,2,2,2,2,2,2,2,2,2,
2,2,2,2,2,2,2,2,2,2,2,2,2,2,2,2,2,2,2,2,2,2,2,2,2,2,2,2,2,2,2,2,2,2,2,2,
2,2,2,2,2,2,2,2,2,2,2,2,2,2,2,2,2,2,2,2,2,2,2,2,2,2,2,2,2,2,2,2,2,2,2,2,
2,2,2,2,2,2,2,2,2,2,2,2,2,2,2,2,2,2,2,2,2,2,2,2,2,2,2,2,2,2,2,2,2,2,2,2,
2,4),(0.000313237606796583,0.0732396125606311,0.107388601669689,0.116229997177897,
0.120739200951735,0.12448068829046,0.12932232799047,0.140221656971463,0.197481902428677,
0.242183482957304,0.258897773384315,0.267128547630496,0.273754482371197,
0.281405825657101,0.294762578788611,0.359832446620594,0.392697716411196,
0.410524918994634,0.416397219067249,0.420282279646255,0.423842780221686,
0.43003701160593,0.449122813102218,0.499312016373005,0.532450329898909,
0.554251024099348,0.563329965988381,0.570055283822999,0.577253748747926,
0.588794905730077,0.63783386640416,0.68555064429509,0.700318391868383,0.71074492774884,
0.715554302770943,0.719289105967843,0.723890692170196,0.733204015963814,
0.775297264573541,0.813397616482522,0.836829411115005,0.854004311242021,
0.862319189947006,0.868890720456341,0.876460021720684,0.889436588905798,
0.958064649980759,0.988901173792772,1.00605964200919,1.01185486548237,1.01572483607133,
1.01981038743091,1.02662506481103,1.05294308186016,1.11603960015384,1.13681639290964,
1.15255038391308,1.16059722623153,1.16657003890367,1.17412248481406,1.18702187013861,
1.26634207907997,1.29860430761864,1.30722407958094,1.31168903283532,1.31543564929409,
1.32033674769295,1.3315838632717,1.38851310549199,1.43301151510683,1.44974680322203,
1.45798167437105,1.46460815319793,1.47225708342722,1.48560161688953,1.5508096408345,
1.58359577756807,1.60139783967576,1.60726747808697,1.61115213976924,1.61471343822002,
1.62091124413417,1.64002901256489,1.69019703923327,1.72332762695399,1.74512535184184,
1.75420411351427,1.76092964789903,1.76812867093258,1.77967145331808,1.82873709616104,
1.87643479990973,1.89120007939844,1.90162546861717,1.906434770132,1.9101697274484,
1.91477176451421,1.92408679796526,1.96636127139429,2.00482306070261,2.02795782992859,
2.0449757045374,2.05326230394008,2.05989243997341,2.06750403665759,2.08067525344837,
2.14761187164537,2.17939332316874,2.19686781230856,2.20270002240954,2.20657731262491,
2.21014682013202,2.21638708153345,2.23591442338624,2.28577745846129,2.33125256327586,
2.3448634669727,2.35249097721753,2.35911945320565,2.36738364623431,2.38048505743541,
2.45126394470639,2.491824698676,2.4990749260843,2.50325459238726,2.50703244418594,
2.51165892580978,2.5230138751059,2.57957652125262,2.62385667981512,2.640608277974,
2.64884637960265,2.65547334481351,2.66312050416494,2.67645581165643,2.74177291493049,
2.77449742393239,2.7922799505251,2.79814754898393,2.80203192776873,2.80559387940277,
2.81179453066218,2.83093749953759,2.88108952277184,2.91421444333614,2.93601008099111,
2.94508878799329,2.95181455092315,2.95901406896798,2.97055820458558,3.01964431923071,
3.06732837603487,3.08209198747141,3.09251664138888,3.09732594073853,3.10106105597637,
3.1056634855733,3.11497990222459,3.15743985639091,3.21906433038732,3.23596923937728,
3.24423525632709,3.25080307478489,3.25840680359813,3.2715414761115,3.33881303289814,
3.37040526765403,3.38781716509415,3.39364215558881,3.39751804612596,3.40108919541907,
3.40733786232631,3.426948013979,3.48278666763428,3.51842522126189,3.53429071536459,
3.54236291286626,3.5483383589686,3.55587295299742,3.56868876036549,3.64839732381433,
3.68047143337749,3.68906884053197,3.6935294641211,3.69727691731241,3.70218474989,
3.71347069177186,3.77036733262433,3.81484680103362,3.83158489220578,3.83982060803806,
3.84644753088318,3.85409671343685,3.86744100221539,3.93266508916591,3.96544623029879,
3.98324714544429,3.98911689971542,3.99300175767898,3.99656333766215,4.0027618249125,
4.02188353105887,4.07205271143324,4.10518460928008,4.12698337883407,4.13606266588215,
4.14278861918699,4.14998811824146,4.16153172542411,4.21060248968077,4.25830151837033,
4.2730674850971,4.28349340724766,4.28830299066872,4.29203818429792,4.29664053409124,
4.30595626291475,4.34934748303688,4.39619782041856,4.41434929080584,4.42857812647288,
4.43633085160234,4.4429505060573,4.45105416420926,4.46359846997177,4.52012220950349,
4.55871685980115,4.57197906541737,4.58161223716024,4.58627531352348,4.5896388918647,
4.59418922081277,4.6032378874983,4.65583263761798,4.69656653463468,4.72135568666745,
4.730856601774,4.73758480567342,4.74462888557875,4.75541960666407,4.79288568239407,
4.82885445160377,4.87344626915557,4.88080474789728,4.88500753632564,4.88881892169032,
4.89429083248362,4.90891007740531,4.93287264334698,5.01162740766663,5.02465998817305,
5.03224150521685,5.03881164645255,5.04710891455437,5.06418654928975,5.08743200694948,
5.12585309495423,5.16790924677788,5.17722081086339,5.18182206712108,5.18555689260041,
5.19036670092958,5.20079548702653,5.21556888747791,5.26331057623244,5.31236987823311,
5.32391216753674,5.33111087790344,5.33783609047363,5.34691438697375,5.36871160436141,
5.40183944885928,5.45201633410622,5.47107788044713,5.47726931209096,5.48082925358337,
5.48471473812841,5.49058942437643,5.50843711943276,5.54136693322142,5.60638140494845,
5.6197470670641,5.62740026155646,5.63402591022171,5.64225388314361,5.65895372302928,
5.70370953468402,5.76105341546906,5.77079415343036,5.77555639304346,5.7793664111699,
5.78347665201096,5.79040604229506,5.82198915488222,5.8857049079595,5.91128857237193,
5.9211610784852,5.92733794405061,5.93417624848413,5.94391888997028,5.97061846915713,
6.01703809091761,6.06096967345059,6.0702767349235,6.07487690866175,6.07861148482227,
6.08342177761782,6.09385448693531,6.10863590921031,6.15643602560443,6.20541939886094,
6.21695774531404,6.22415527180339,6.23088023313038,6.23995951770358,6.261766258068,
6.29491770242867,6.34515755983286,6.36412883642266,6.37031032870974,6.3738681807214,
6.37775507522321,6.38363788156199,6.40156027295113,6.43472527589361,6.49934039243712,
6.51273957205739,6.52039961020333,6.52702412278388,6.53524154289608,6.55188625378585,
6.5967321111915,6.65408992772509,6.66381299538236,6.66857090801069,6.67237964758556,
6.67649143080277,6.68342886648739,6.71518648574016,6.77978011830595,6.80455227971896,
6.81430962319356,6.82108212878374,6.82805754263332,6.83851346682056,6.87195972478911,
6.95215361079866,6.96269806089745,6.96752838705944,6.97126383418314,6.97584690258443,
6.98506573626334,7.02263603588288,7.09433868882286,7.10799292718832,7.11570737876551,
7.12232755374372,7.13047392861467,7.14673772581042,7.20925409112281,7.25175036210626,
7.26106350359465,7.26566474748929,7.26939912698676,7.27420780311051,7.28463214639486,
7.29939754904456,7.34709095519899,7.39619443290078,7.40773763475398,7.4149359919494,
7.42166025661953,7.43073631439035,7.4525229928785,7.48562823741736,7.53575129037795,
7.55487486475011,7.56107238851728,7.56463323392608,7.56851706622811,7.57438498142335,
7.59217665456648,7.62493481732375,7.69022330462129,7.70356180776332,7.71120861885677,
7.71783400362131,7.72606848306152,7.74280685165591,7.78714839928332,7.84382330403291,
7.85529557183305,7.86023376188207,7.8639833645544,7.86842058678017,7.87690577738169,
7.88810374115488,7.91676560401724,7.98957914746058,8.00215087631491,8.00956315584407,
8.01622251652062,8.02482648592442,8.04365816094504,8.07033861727407,8.10460906787267,
8.14806363667771,8.15537705237786,8.15956945765984,8.16338350099015,8.16887609108397,
8.18365337250209,8.20801392577201,8.28573096649293,8.29897840424588,8.30660499365386,
8.31323133193775,8.32149111057444,8.33837102002009,8.38106655106261,8.4352194528517,
8.44928421307062,8.45482389939674,8.45860817415939,8.46276801406585,8.46993053964016,
8.50739522920647,8.56970187884935,8.59163513100119,8.60096217952688,8.60772586212575,
8.61483428769196,8.62594833814482,8.66832213642274,8.68365072489435,8.74111159240067,
8.7496274961707,8.75412329755277,8.75786472642003,8.76280357698595,8.77397110823675,
8.79020879126153,8.84939545791893,8.88566667308928,8.89658894894715,8.90365793660862,
8.91044347639736,8.91989866627855,8.94436484759657,8.98422036065577,9.03835238060195,
9.04708268240285,9.05162363084941,9.05532514558369,9.06018348337513,9.07088942244905,
9.08620626270874,9.13783286586151,9.18237623172095,9.19373048934184,9.20088857749546,
9.20762799411705,9.21680752646988,9.23930234293591,9.27409640251205,9.32864526177467,
9.34224801874259,9.34771243020849,9.35152134447465,9.35572449427036,9.36308997113074,
9.41097147200668,9.44274043488676),.UNSPECIFIED.);
#409=B_SPLINE_CURVE_WITH_KNOTS('',3,(#36835,#36836,#36837,#36838,#36839,
#36840,#36841,#36842,#36843,#36844,#36845,#36846,#36847,#36848,#36849,#36850,
#36851,#36852,#36853,#36854,#36855,#36856,#36857,#36858,#36859,#36860,#36861,
#36862,#36863,#36864,#36865,#36866,#36867,#36868,#36869,#36870,#36871,#36872,
#36873,#36874,#36875,#36876,#36877,#36878,#36879,#36880,#36881,#36882,#36883,
#36884,#36885,#36886,#36887,#36888,#36889,#36890,#36891,#36892,#36893,#36894,
#36895,#36896,#36897,#36898,#36899,#36900,#36901,#36902,#36903,#36904,#36905,
#36906,#36907,#36908,#36909,#36910,#36911,#36912,#36913,#36914,#36915,#36916,
#36917,#36918,#36919,#36920,#36921,#36922,#36923,#36924,#36925,#36926,#36927,
#36928,#36929,#36930,#36931,#36932,#36933,#36934,#36935,#36936,#36937,#36938,
#36939,#36940,#36941,#36942,#36943,#36944,#36945,#36946,#36947,#36948,#36949,
#36950,#36951,#36952,#36953,#36954,#36955,#36956,#36957,#36958,#36959,#36960,
#36961,#36962,#36963,#36964,#36965,#36966,#36967,#36968,#36969,#36970,#36971,
#36972,#36973,#36974,#36975,#36976,#36977,#36978,#36979,#36980,#36981,#36982,
#36983,#36984,#36985,#36986,#36987,#36988,#36989,#36990,#36991,#36992,#36993,
#36994,#36995,#36996,#36997,#36998,#36999,#37000,#37001,#37002,#37003,#37004,
#37005,#37006,#37007,#37008,#37009,#37010,#37011,#37012,#37013,#37014,#37015,
#37016,#37017,#37018,#37019,#37020,#37021,#37022,#37023,#37024,#37025,#37026,
#37027,#37028,#37029,#37030,#37031,#37032,#37033,#37034,#37035,#37036,#37037,
#37038,#37039,#37040,#37041,#37042,#37043,#37044,#37045,#37046,#37047,#37048,
#37049,#37050,#37051,#37052,#37053,#37054,#37055,#37056,#37057,#37058,#37059,
#37060,#37061,#37062,#37063,#37064,#37065,#37066,#37067,#37068,#37069,#37070,
#37071,#37072,#37073,#37074,#37075,#37076,#37077,#37078,#37079,#37080,#37081,
#37082,#37083,#37084,#37085,#37086,#37087,#37088,#37089,#37090,#37091,#37092,
#37093,#37094,#37095,#37096,#37097,#37098,#37099,#37100,#37101,#37102,#37103,
#37104,#37105,#37106,#37107,#37108,#37109,#37110,#37111,#37112,#37113,#37114,
#37115,#37116,#37117,#37118,#37119,#37120,#37121,#37122,#37123,#37124,#37125,
#37126,#37127,#37128,#37129,#37130,#37131,#37132,#37133,#37134,#37135,#37136,
#37137,#37138,#37139,#37140,#37141,#37142,#37143,#37144,#37145,#37146,#37147,
#37148,#37149,#37150,#37151,#37152,#37153,#37154,#37155,#37156,#37157,#37158,
#37159,#37160,#37161,#37162,#37163,#37164,#37165,#37166,#37167,#37168,#37169,
#37170,#37171,#37172,#37173,#37174,#37175,#37176,#37177,#37178,#37179,#37180,
#37181,#37182,#37183,#37184,#37185,#37186,#37187,#37188,#37189,#37190,#37191,
#37192,#37193,#37194,#37195,#37196,#37197,#37198,#37199,#37200,#37201,#37202,
#37203,#37204,#37205,#37206,#37207,#37208,#37209,#37210,#37211,#37212,#37213,
#37214,#37215,#37216,#37217,#37218,#37219,#37220,#37221,#37222,#37223,#37224),
 .UNSPECIFIED.,.F.,.F.,(4,2,2,2,2,2,2,2,2,2,2,2,2,2,2,2,2,2,2,2,2,2,2,2,
2,2,2,2,2,2,2,2,2,2,2,2,2,2,2,2,2,2,2,2,2,2,2,2,2,2,2,2,2,2,2,2,2,2,2,2,
2,2,2,2,2,2,2,2,2,2,2,2,2,2,2,2,2,2,2,2,2,2,2,2,2,2,2,2,2,2,2,2,2,2,2,2,
2,2,2,2,2,2,2,2,2,2,2,2,2,2,2,2,2,2,2,2,2,2,2,2,2,2,2,2,2,2,2,2,2,2,2,2,
2,2,2,2,2,2,2,2,2,2,2,2,2,2,2,2,2,2,2,2,2,2,2,2,2,2,2,2,2,2,2,2,2,2,2,2,
2,2,2,2,2,2,2,2,2,2,2,2,2,2,2,2,2,2,2,2,2,2,2,2,2,2,4),(9.99999999526152E-7,
0.02541508705979,0.0403509785521346,0.0478988957842898,0.0541473169418411,
0.0607715627350446,0.0689794030361682,0.0850231306095784,0.140555435079713,
0.173585934480102,0.188350097916006,0.198774669984789,0.203583572743684,
0.20731820680062,0.211919827642413,0.221233979609255,0.264646346264958,
0.311470042953097,0.329614886335042,0.343839280917871,0.35159037156107,
0.35820904340011,0.366312017366255,0.378856297343035,0.435269542521666,
0.473931972186144,0.49349270960845,0.499550744538113,0.503473421030138,
0.506997351234623,0.512999204789748,0.53040898313939,0.581879644126399,
0.623712128187474,0.640123710024594,0.648298060722711,0.654920127170653,
0.662613387749988,0.67616713643093,0.738608872800642,0.773101424473421,
0.791440449153294,0.797369422545081,0.80126564039814,0.804814062124252,
0.810945956436549,0.829461537871561,0.886330892904588,0.921781420161633,
0.937943429823994,0.946071029843745,0.952690622809616,0.960421006174729,
0.97414880871105,1.03185979384175,1.06958924070581,1.08268946443784,1.09223470828921,
1.09688056522918,1.10024265388201,1.1048070309001,1.11393025772448,1.1799559966417,
1.21189033405176,1.2331676438347,1.24216632496867,1.24887863916426,1.25610686702012,
1.26779453972329,1.31837403481817,1.35636457635536,1.38506419660503,1.39183807772474,
1.39591435594572,1.39974303726536,1.40552566248542,1.42124676978749,1.47406019861245,
1.50820862862716,1.53043596827541,1.5395775531375,1.54631192021341,1.55348559060862,
1.56491065125921,1.60926620515102,1.66090596941392,1.67622375644931,1.68693143540261,
1.69179065888691,1.69549305560627,1.70003539947624,1.70876887097193,1.76293424303464,
1.80280979026846,1.82728429692332,1.83674210724431,1.84352928172483,1.84976015883669,
1.8599462518553,1.88823141575172,1.94179659623945,1.97943655892693,1.98669149214734,
1.99087159173205,1.99469084996073,2.00021440726323,2.01522176968697,2.04016382138305,
2.1164765391538,2.13002112034464,2.13771127091191,2.14433177541148,2.15250559103361,
2.16892119780121,2.21093710449602,2.26274000132455,2.27967966095738,2.28562176463385,
2.28913403699085,2.29306869599499,2.29918716107689,2.31935976452665,2.36028657690867,
2.41367472917936,2.42626028226952,2.43437464521228,2.44099296215536,2.44873263999628,
2.46290364477065,2.48095745045831,2.52734101885416,2.57129836700053,2.58060409495587,
2.58520405916938,2.58893983523734,2.59375359411506,2.6041978076728,2.6190006463112,
2.66695430111742,2.71567951130462,2.72720795203295,2.73440477612739,2.7411329213571,
2.75022265791473,2.77208905832678,2.80537678018994,2.85596265538789,2.87447221987865,
2.88060315926801,2.88415128178029,2.88804330123993,2.89396506363409,2.91227355281239,
2.94667645633749,3.00935373112116,3.02289418062897,3.03057962783057,3.03719446225264,
3.04535893359252,3.06174596062229,3.10327548774194,3.15420939777526,3.17226518965298,
3.17834083402444,3.18187622467,3.18577996015993,3.19175249373992,3.21050493335888,
3.24635311542894,3.30691938175137,3.32057951640045,3.3282967358863,3.33491892847784,
3.34306739813751,3.35933488529976,3.42197603469795,3.46418131911456,3.47353803357934,
3.47815099013026,3.48189654725739,3.48672299886183,3.49718158689922,3.51200355480281,
3.56010114755446,3.60825547711487,3.6197700369559,3.62697430206707,3.63372116635705,
3.64285552699046,3.66494112643857,3.69871103664215,3.76234943713865,3.77115339485521,
3.77402045671866,3.77647229296193),.UNSPECIFIED.);
#410=B_SPLINE_CURVE_WITH_KNOTS('',3,(#37226,#37227,#37228,#37229,#37230,
#37231,#37232,#37233,#37234,#37235,#37236,#37237,#37238,#37239,#37240,#37241,
#37242,#37243,#37244,#37245,#37246,#37247,#37248,#37249,#37250,#37251,#37252,
#37253,#37254,#37255,#37256,#37257,#37258,#37259,#37260,#37261,#37262,#37263,
#37264,#37265,#37266,#37267,#37268,#37269,#37270,#37271,#37272,#37273,#37274,
#37275,#37276,#37277,#37278,#37279,#37280,#37281,#37282,#37283,#37284,#37285,
#37286,#37287,#37288,#37289,#37290,#37291,#37292,#37293,#37294,#37295,#37296,
#37297,#37298,#37299,#37300,#37301,#37302,#37303,#37304,#37305,#37306,#37307,
#37308,#37309,#37310,#37311,#37312,#37313,#37314,#37315,#37316,#37317,#37318,
#37319,#37320,#37321,#37322,#37323,#37324,#37325,#37326,#37327),
 .UNSPECIFIED.,.F.,.F.,(4,2,2,2,2,2,2,2,2,2,2,2,2,2,2,2,2,2,2,2,2,2,2,2,
2,2,2,2,2,2,2,2,2,2,2,2,2,2,2,2,2,2,2,2,2,2,2,2,2,2,4),(0.000274590634593237,
0.0025082762786118,0.00535069727310344,0.0116844857126863,0.0342991856608529,
0.0843016193333742,0.115297757508164,0.136139369508367,0.145022650646858,
0.151667283405926,0.158837468056138,0.170458820756428,0.221014938736121,
0.267413615605875,0.281958972332198,0.292254398082525,0.297016468905675,
0.300730962418017,0.305324808844561,0.314619905230995,0.357647295962238,
0.419422814912621,0.436370390294811,0.444655812784192,0.451299173082329,
0.458941834237123,0.472211170200764,0.516280100710487,0.546464638149321,
0.58483144266112,0.59212456635804,0.596333234407501,0.600256784222936,0.605985302348148,
0.621931521037642,0.649320403068425,0.720955334511645,0.733274317749864,
0.740699761065403,0.747479592700835,0.756403816803348,0.776727475649347,
0.804043104311228,0.856916121248536,0.88117922472343,0.887847382211191,
0.891895834338558,0.895605417154939,0.899318875233909,0.904616105327427,
0.944316620293279),.UNSPECIFIED.);
#411=B_SPLINE_CURVE_WITH_KNOTS('',3,(#37331,#37332,#37333,#37334,#37335,
#37336,#37337),.UNSPECIFIED.,.F.,.F.,(4,1,1,1,4),(0.,0.25,0.5,0.75,1.),
 .UNSPECIFIED.);
#412=B_SPLINE_CURVE_WITH_KNOTS('',3,(#37339,#37340,#37341,#37342,#37343,
#37344,#37345,#37346,#37347,#37348,#37349,#37350,#37351,#37352,#37353,#37354,
#37355,#37356,#37357,#37358,#37359,#37360,#37361,#37362,#37363,#37364,#37365,
#37366,#37367,#37368,#37369,#37370,#37371,#37372,#37373,#37374,#37375,#37376,
#37377,#37378,#37379,#37380,#37381,#37382,#37383,#37384,#37385,#37386,#37387,
#37388,#37389,#37390,#37391,#37392,#37393,#37394,#37395,#37396,#37397,#37398,
#37399,#37400,#37401,#37402,#37403,#37404,#37405,#37406,#37407,#37408,#37409,
#37410,#37411,#37412,#37413,#37414,#37415,#37416,#37417,#37418,#37419,#37420,
#37421,#37422,#37423,#37424,#37425,#37426,#37427,#37428,#37429),
 .UNSPECIFIED.,.F.,.F.,(4,3,3,3,3,3,3,3,3,3,3,3,3,3,3,3,3,3,3,3,3,3,3,3,
3,3,3,3,3,3,4),(1.01781475985858E-6,0.0978279187980743,0.125,0.1875,0.25,
0.255532112875372,0.3125,0.375,0.40625,0.413169433494558,0.4375,0.46875,
0.484375,0.4921875,0.5,0.5078125,0.515625,0.53125,0.5625,0.59375,0.625,
0.627666778982696,0.6875,0.75,0.800182159962401,0.8125,0.875,0.924421520907667,
0.9375,0.992828832419945,0.999999605898017),.UNSPECIFIED.);
#413=B_SPLINE_CURVE_WITH_KNOTS('',3,(#37431,#37432,#37433,#37434,#37435,
#37436,#37437,#37438,#37439,#37440,#37441,#37442,#37443,#37444,#37445,#37446,
#37447,#37448,#37449,#37450,#37451,#37452,#37453,#37454,#37455,#37456,#37457,
#37458,#37459,#37460,#37461,#37462,#37463,#37464,#37465,#37466,#37467,#37468,
#37469,#37470,#37471,#37472,#37473,#37474,#37475,#37476,#37477,#37478,#37479),
 .UNSPECIFIED.,.F.,.F.,(4,3,3,3,3,3,3,3,3,3,3,3,3,3,3,3,4),(0.,0.0886352608471135,
0.125,0.212002569513292,0.25,0.33732431895677,0.375,0.462307893887243,0.5,
0.587307893887231,0.625,0.712324318956778,0.75,0.837002569513291,0.875,
0.963635260847104,1.),.UNSPECIFIED.);
#414=B_SPLINE_CURVE_WITH_KNOTS('',3,(#37481,#37482,#37483,#37484,#37485,
#37486,#37487,#37488,#37489,#37490,#37491,#37492,#37493,#37494,#37495,#37496,
#37497,#37498,#37499,#37500,#37501,#37502,#37503,#37504,#37505,#37506,#37507,
#37508,#37509,#37510,#37511,#37512,#37513,#37514,#37515,#37516,#37517,#37518,
#37519,#37520,#37521,#37522,#37523,#37524,#37525,#37526,#37527,#37528,#37529),
 .UNSPECIFIED.,.F.,.F.,(4,3,3,3,3,3,3,3,3,3,3,3,3,3,3,3,4),(0.,0.0886238521664878,
0.125,0.211990985604023,0.25,0.337312738768364,0.375,0.462296334182994,
0.5,0.587296334182989,0.625,0.71231273876836,0.75,0.836990985604029,0.875,
0.96362385216648,1.),.UNSPECIFIED.);
#415=B_SPLINE_CURVE_WITH_KNOTS('',3,(#37531,#37532,#37533,#37534,#37535,
#37536,#37537,#37538,#37539,#37540,#37541,#37542,#37543,#37544,#37545,#37546,
#37547,#37548,#37549,#37550,#37551,#37552,#37553,#37554,#37555,#37556,#37557,
#37558,#37559,#37560,#37561,#37562,#37563,#37564,#37565,#37566,#37567,#37568,
#37569,#37570,#37571,#37572,#37573,#37574,#37575,#37576,#37577,#37578,#37579),
 .UNSPECIFIED.,.F.,.F.,(4,3,3,3,3,3,3,3,3,3,3,3,3,3,3,3,4),(1.00099247898549E-6,
0.0886113417660512,0.125,0.211978963112827,0.25,0.337305507603416,0.375,
0.462245106775286,0.5,0.587333725456046,0.625,0.712305984259491,0.75,0.836989030990787,
0.875,0.963623492160247,0.999999791341556),.UNSPECIFIED.);
#416=B_SPLINE_CURVE_WITH_KNOTS('',3,(#37581,#37582,#37583,#37584,#37585,
#37586,#37587,#37588,#37589,#37590,#37591,#37592,#37593,#37594,#37595,#37596,
#37597,#37598,#37599,#37600,#37601,#37602,#37603,#37604,#37605,#37606,#37607,
#37608,#37609,#37610,#37611,#37612,#37613,#37614,#37615,#37616,#37617,#37618,
#37619,#37620,#37621,#37622,#37623,#37624,#37625,#37626,#37627,#37628,#37629),
 .UNSPECIFIED.,.F.,.F.,(4,3,3,3,3,3,3,3,3,3,3,3,3,3,3,3,4),(0.,0.0886378390083851,
0.125,0.212005187268809,0.25,0.337326935869751,0.375,0.462310506172766,
0.5,0.587310506172741,0.625,0.712326935869763,0.75,0.837005187268801,0.875,
0.963637839008402,1.),.UNSPECIFIED.);
#417=B_SPLINE_CURVE_WITH_KNOTS('',3,(#37631,#37632,#37633,#37634,#37635,
#37636,#37637,#37638,#37639,#37640,#37641,#37642,#37643,#37644,#37645,#37646,
#37647,#37648,#37649,#37650,#37651,#37652,#37653,#37654,#37655,#37656,#37657,
#37658,#37659,#37660,#37661,#37662,#37663,#37664,#37665,#37666,#37667,#37668,
#37669,#37670,#37671,#37672,#37673,#37674,#37675,#37676,#37677,#37678,#37679),
 .UNSPECIFIED.,.F.,.F.,(4,3,3,3,3,3,3,3,3,3,3,3,3,3,3,3,4),(0.,0.0886216790948839,
0.125,0.211988779152122,0.25,0.337310533023806,0.375,0.462294132341469,
0.5,0.58729413234147,0.625,0.712310533023803,0.75,0.836988779152123,0.875,
0.963621679094858,1.),.UNSPECIFIED.);
#418=B_SPLINE_CURVE_WITH_KNOTS('',3,(#37681,#37682,#37683,#37684,#37685,
#37686,#37687,#37688,#37689,#37690,#37691,#37692,#37693,#37694,#37695,#37696,
#37697,#37698,#37699,#37700,#37701,#37702,#37703,#37704,#37705,#37706,#37707,
#37708,#37709,#37710,#37711,#37712,#37713,#37714,#37715,#37716,#37717,#37718,
#37719,#37720,#37721,#37722,#37723,#37724,#37725,#37726,#37727,#37728,#37729),
 .UNSPECIFIED.,.F.,.F.,(4,3,3,3,3,3,3,3,3,3,3,3,3,3,3,3,4),(7.23012916031714E-7,
0.0886177045235499,0.125,0.211984073096313,0.25,0.337305828475216,0.375,
0.462289436118893,0.5,0.5872894361189,0.625,0.712305828475213,0.75,0.836984073096328,
0.875,0.963617044238319,1.),.UNSPECIFIED.);
#419=B_SPLINE_CURVE_WITH_KNOTS('',3,(#37731,#37732,#37733,#37734,#37735,
#37736,#37737,#37738,#37739,#37740,#37741,#37742,#37743,#37744,#37745,#37746,
#37747,#37748,#37749,#37750,#37751,#37752,#37753,#37754,#37755,#37756,#37757,
#37758,#37759,#37760,#37761,#37762,#37763,#37764,#37765,#37766,#37767,#37768,
#37769,#37770,#37771,#37772,#37773,#37774,#37775,#37776,#37777,#37778,#37779),
 .UNSPECIFIED.,.F.,.F.,(4,3,3,3,3,3,3,3,3,3,3,3,3,3,3,3,4),(0.,0.0886395817675682,
0.125,0.212006956791507,0.25,0.337328704822608,0.375,0.462312271997881,
0.5,0.587312271997905,0.625,0.712328704822597,0.75,0.837006956791513,0.875,
0.963639581767539,1.),.UNSPECIFIED.);
#420=B_SPLINE_CURVE_WITH_KNOTS('',3,(#37781,#37782,#37783,#37784,#37785,
#37786,#37787,#37788,#37789,#37790,#37791,#37792,#37793,#37794,#37795,#37796,
#37797,#37798,#37799,#37800,#37801,#37802,#37803,#37804,#37805,#37806,#37807,
#37808,#37809,#37810,#37811,#37812,#37813,#37814,#37815,#37816,#37817,#37818,
#37819,#37820,#37821,#37822,#37823,#37824,#37825,#37826,#37827,#37828,#37829),
 .UNSPECIFIED.,.F.,.F.,(4,3,3,3,3,3,3,3,3,3,3,3,3,3,3,3,4),(0.,0.0886188875000415,
0.125,0.211985944674266,0.25,0.337307699454002,0.375,0.462291303786219,
0.5,0.587291303786234,0.625,0.712307699453993,0.75,0.836985944674267,0.875,
0.963618887500054,1.),.UNSPECIFIED.);
#421=B_SPLINE_CURVE_WITH_KNOTS('',3,(#37831,#37832,#37833,#37834,#37835,
#37836,#37837,#37838,#37839,#37840,#37841,#37842,#37843,#37844,#37845,#37846,
#37847,#37848,#37849,#37850,#37851,#37852),.UNSPECIFIED.,.F.,.F.,(4,3,3,
3,3,3,3,4),(8.83577889380245E-7,0.195536634947496,0.25,0.5,0.566780896033298,
0.75,0.937584669068563,1.),.UNSPECIFIED.);
#422=B_SPLINE_CURVE_WITH_KNOTS('',3,(#37856,#37857,#37858,#37859,#37860,
#37861,#37862,#37863,#37864,#37865,#37866,#37867,#37868,#37869,#37870,#37871,
#37872,#37873,#37874,#37875,#37876,#37877,#37878,#37879,#37880,#37881,#37882,
#37883,#37884,#37885,#37886,#37887,#37888,#37889,#37890,#37891,#37892,#37893,
#37894,#37895,#37896,#37897,#37898,#37899,#37900,#37901,#37902,#37903,#37904,
#37905,#37906,#37907,#37908,#37909,#37910,#37911,#37912,#37913,#37914,#37915,
#37916,#37917,#37918,#37919,#37920,#37921,#37922,#37923,#37924,#37925,#37926,
#37927,#37928,#37929,#37930,#37931,#37932,#37933,#37934,#37935,#37936,#37937,
#37938,#37939,#37940,#37941,#37942,#37943,#37944,#37945,#37946,#37947,#37948,
#37949,#37950,#37951,#37952,#37953,#37954,#37955,#37956,#37957,#37958,#37959,
#37960,#37961,#37962,#37963,#37964,#37965,#37966,#37967,#37968,#37969,#37970,
#37971,#37972,#37973,#37974,#37975,#37976,#37977,#37978,#37979,#37980,#37981,
#37982,#37983,#37984,#37985,#37986,#37987,#37988,#37989,#37990,#37991,#37992,
#37993,#37994,#37995,#37996,#37997,#37998,#37999,#38000,#38001,#38002,#38003,
#38004,#38005,#38006,#38007,#38008,#38009,#38010,#38011,#38012,#38013,#38014,
#38015,#38016,#38017,#38018,#38019,#38020,#38021,#38022,#38023,#38024,#38025,
#38026,#38027,#38028,#38029,#38030,#38031,#38032,#38033,#38034,#38035,#38036,
#38037,#38038,#38039,#38040,#38041,#38042,#38043,#38044,#38045,#38046,#38047,
#38048,#38049,#38050,#38051,#38052,#38053,#38054,#38055,#38056,#38057,#38058,
#38059,#38060,#38061,#38062,#38063,#38064,#38065,#38066,#38067,#38068,#38069,
#38070,#38071,#38072,#38073,#38074,#38075,#38076,#38077,#38078,#38079,#38080,
#38081,#38082,#38083,#38084,#38085,#38086,#38087,#38088,#38089,#38090,#38091,
#38092,#38093,#38094,#38095,#38096,#38097,#38098,#38099,#38100,#38101,#38102,
#38103,#38104,#38105,#38106,#38107,#38108,#38109,#38110,#38111,#38112,#38113,
#38114,#38115,#38116,#38117,#38118,#38119,#38120,#38121,#38122,#38123,#38124,
#38125,#38126,#38127,#38128,#38129,#38130,#38131,#38132,#38133,#38134,#38135,
#38136,#38137,#38138,#38139,#38140,#38141,#38142,#38143,#38144,#38145,#38146,
#38147,#38148,#38149,#38150,#38151,#38152,#38153,#38154,#38155,#38156,#38157,
#38158,#38159,#38160,#38161,#38162,#38163,#38164,#38165,#38166,#38167,#38168,
#38169,#38170,#38171,#38172,#38173,#38174,#38175,#38176,#38177,#38178,#38179,
#38180,#38181,#38182,#38183,#38184,#38185,#38186,#38187,#38188,#38189,#38190,
#38191,#38192,#38193,#38194,#38195,#38196,#38197),.UNSPECIFIED.,.F.,.F.,
(4,2,2,2,2,2,2,2,2,2,2,2,2,2,2,2,2,2,2,2,2,2,2,2,2,2,2,2,2,2,2,2,2,2,2,
2,2,2,2,2,2,2,2,2,2,2,2,2,2,2,2,2,2,2,2,2,2,2,2,2,2,2,2,2,2,2,2,2,2,2,2,
2,2,2,2,2,2,2,2,2,2,2,2,2,2,2,2,2,2,2,2,2,2,2,2,2,2,2,2,2,2,2,2,2,2,2,2,
2,2,2,2,2,2,2,2,2,2,2,2,2,2,2,2,2,2,2,2,2,2,2,2,2,2,2,2,2,2,2,2,2,2,2,2,
2,2,2,2,2,2,2,2,2,2,2,2,2,2,2,2,2,2,2,2,2,2,2,2,2,2,2,4),(1.00000000230168E-6,
0.00270686683477302,0.00578013839413656,0.0146631673706884,0.0546195079158328,
0.0956849417342354,0.118927518992973,0.128775936846263,0.136252617995142,
0.144478190542676,0.15828221299073,0.235046296377132,0.268196766064285,
0.286394477892574,0.292358443255677,0.296284179023899,0.300167040939504,
0.306427742313422,0.327922114008251,0.382123323164708,0.422311158381288,
0.434910252745757,0.44208371144609,0.448366899237495,0.456249172852546,
0.468792601527292,0.518955441473817,0.565719787146273,0.587278799532253,
0.593306598296846,0.597114659355356,0.600569798001007,0.606200418528769,
0.620832369761187,0.681981858298264,0.727563855778881,0.738978699544188,
0.74623072370966,0.753102243049817,0.762541754626802,0.784632816535728,
0.854402797787406,0.872707911890411,0.884903098454377,0.890096691313338,
0.893939824049587,0.898434112826663,0.906811756910079,0.965737406041129,
1.01356858983867,1.02932012397361,1.03739325442462,1.04339391787124,1.05099379254819,
1.06400661622428,1.14359015573781,1.16749357497808,1.18210231392832,1.18757632047122,
1.19138593847589,1.19556216209836,1.20286773363048,1.2466503732369,1.28143691110029,
1.30769572225958,1.32629495305924,1.3348254503737,1.34143774786581,1.34880564804806,
1.36131579902078,1.43480064613803,1.46340841333038,1.47457962120612,1.48303969140981,
1.4874513914218,1.49119059442889,1.49611282537706,1.50747844961977,1.56433476114742,
1.5999989598884,1.6228690473338,1.63211938844692,1.63888586197319,1.64605080500312,
1.65737090731572,1.69875233824027,1.71627196787867,1.77144690675703,1.78010852447289,
1.78464710306606,1.78836201207362,1.79326289410475,1.80418399198311,1.81992038509624,
1.87477223330872,1.91547880593922,1.92675713612992,1.93390293673173,1.9406553847883,
1.94989187936498,1.97274951265969,2.00840714107598,2.06528199524312,2.07552357683295,
2.08093377673006,2.08473347450726,2.08895721789922,2.09642566664508,2.10589791876019,
2.1277654222735,2.19494631184431,2.21746004485472,2.2268522049097,2.23355637160797,
2.24062130216056,2.25153928621326,2.29086867062449,2.32564080626157,2.36938832195415,
2.37670926188997,2.38090107982992,2.3847139624554,2.3901998970205,2.40492153443202,
2.42913968770142,2.50724404223848,2.52041822514432,2.52803163635923,2.53466351050005,
2.54295266287335,2.55997873443911,2.58312787154005,2.6215354819646,2.66369352930304,
2.67300467983656,2.67760717712282,2.68134300104556,2.68615471963433,2.69659405653731,
2.7113881985145,2.75927686564514,2.80813803034489,2.81967068926964,2.82686675018931,
2.83359174147683,2.84267322490722,2.86449650877761,2.89768572387087,2.94801408370866,
2.9668763350307,2.97304553205218,2.97660063326439,2.98048876321959,2.98638034958086,
3.00438735807661,3.03782125689201,3.10198182120185,3.11542156423178,3.1230894359458,
3.12971193330523,3.13791546624242,3.15449005265703,3.19892062263756,3.25528526333678,
3.26680140627161,3.27145400415412,3.27523692698049,3.2794004830943,3.28657865243074,
3.32452173193262,3.39737921865892),.UNSPECIFIED.);
#423=B_SPLINE_CURVE_WITH_KNOTS('',3,(#38198,#38199,#38200,#38201),
 .UNSPECIFIED.,.F.,.F.,(4,4),(0.5,0.500496609805673),.UNSPECIFIED.);
#424=B_SPLINE_CURVE_WITH_KNOTS('',3,(#38203,#38204,#38205,#38206,#38207,
#38208),.UNSPECIFIED.,.F.,.F.,(4,2,4),(-0.00141044735461021,-0.000756989983528312,
-0.000100211350264882),.UNSPECIFIED.);
#425=B_SPLINE_CURVE_WITH_KNOTS('',3,(#38212,#38213,#38214,#38215,#38216,
#38217,#38218,#38219,#38220,#38221,#38222,#38223,#38224,#38225,#38226,#38227,
#38228,#38229,#38230,#38231,#38232,#38233,#38234,#38235,#38236,#38237,#38238,
#38239,#38240,#38241,#38242,#38243,#38244,#38245,#38246,#38247,#38248,#38249,
#38250,#38251,#38252,#38253,#38254,#38255,#38256,#38257,#38258,#38259,#38260),
 .UNSPECIFIED.,.F.,.F.,(4,3,3,3,3,3,3,3,3,3,3,3,3,3,3,3,4),(0.,0.0927679075208042,
0.125,0.216059062020963,0.25,0.341395816579201,0.375,0.466378627087965,
0.5,0.591378627088015,0.625,0.716395816579185,0.75,0.841059062020798,0.875,
0.967767907520689,1.),.UNSPECIFIED.);
#426=B_SPLINE_CURVE_WITH_KNOTS('',3,(#38262,#38263,#38264,#38265,#38266,
#38267,#38268,#38269,#38270,#38271,#38272,#38273,#38274,#38275,#38276,#38277,
#38278,#38279,#38280,#38281,#38282,#38283,#38284,#38285,#38286,#38287,#38288,
#38289,#38290,#38291,#38292,#38293,#38294,#38295,#38296,#38297,#38298,#38299,
#38300,#38301,#38302,#38303,#38304,#38305,#38306,#38307,#38308,#38309,#38310,
#38311,#38312,#38313,#38314,#38315,#38316,#38317,#38318,#38319,#38320,#38321,
#38322,#38323,#38324,#38325,#38326,#38327,#38328,#38329,#38330,#38331,#38332,
#38333,#38334,#38335,#38336,#38337,#38338,#38339,#38340,#38341,#38342,#38343,
#38344,#38345,#38346,#38347,#38348,#38349,#38350,#38351,#38352,#38353,#38354,
#38355,#38356,#38357,#38358,#38359,#38360,#38361,#38362,#38363,#38364,#38365,
#38366,#38367,#38368,#38369,#38370),.UNSPECIFIED.,.F.,.F.,(4,3,3,3,3,3,
3,3,3,3,3,3,3,3,3,3,3,3,3,3,3,3,3,3,3,3,3,3,3,3,3,3,3,3,3,3,4),(1.46787644835882E-7,
0.0459840424349436,0.0625,0.0640257524258921,0.117713071409535,0.125,0.167674721829891,
0.1875,0.25,0.3125,0.324179685500434,0.375,0.40625,0.4375,0.46875,0.484375,
0.5,0.515625,0.53125,0.5625,0.625,0.634598942174335,0.65625,0.6875,0.71875,
0.734375,0.742632729388345,0.750148009590237,0.757120179138782,0.769674509629174,
0.78125,0.8125,0.84375,0.875,0.926573451013963,0.9375,0.999999590615941),
 .UNSPECIFIED.);
#427=B_SPLINE_CURVE_WITH_KNOTS('',3,(#38372,#38373,#38374,#38375,#38376,
#38377,#38378,#38379,#38380,#38381,#38382,#38383,#38384,#38385,#38386,#38387,
#38388,#38389,#38390,#38391,#38392,#38393,#38394,#38395,#38396,#38397,#38398,
#38399,#38400,#38401,#38402,#38403,#38404,#38405,#38406,#38407,#38408,#38409,
#38410,#38411,#38412,#38413,#38414,#38415,#38416,#38417,#38418,#38419,#38420),
 .UNSPECIFIED.,.F.,.F.,(4,3,3,3,3,3,3,3,3,3,3,3,3,3,3,3,4),(0.,0.0927529117207158,
0.125,0.216043835888795,0.25,0.341380595334184,0.375,0.466363432770545,
0.5,0.591363432771095,0.625,0.716380595334513,0.75,0.841043835888631,0.875,
0.967752911720961,1.),.UNSPECIFIED.);
#428=B_SPLINE_CURVE_WITH_KNOTS('',3,(#38422,#38423,#38424,#38425,#38426,
#38427,#38428,#38429,#38430,#38431,#38432,#38433,#38434,#38435,#38436,#38437,
#38438,#38439,#38440,#38441,#38442,#38443,#38444,#38445,#38446,#38447,#38448,
#38449,#38450,#38451,#38452,#38453,#38454,#38455),.UNSPECIFIED.,.F.,.F.,
(4,2,2,2,2,2,2,2,2,2,2,2,2,2,2,2,4),(0.,0.0927729654601161,0.125,0.216064197637713,
0.25,0.341400950542809,0.375,0.466383751973243,0.5,0.591383751973228,0.625,
0.716400950542821,0.75,0.841064197637697,0.875,0.967772965460199,1.),
 .UNSPECIFIED.);
#429=B_SPLINE_CURVE_WITH_KNOTS('',3,(#38461,#38462,#38463,#38464,#38465,
#38466,#38467,#38468,#38469,#38470,#38471,#38472,#38473,#38474,#38475,#38476,
#38477,#38478,#38479,#38480,#38481,#38482,#38483,#38484,#38485),
 .UNSPECIFIED.,.F.,.F.,(4,3,3,3,3,3,3,3,4),(0.,0.125,0.25,0.375,0.5,0.625,
0.75,0.875,1.),.UNSPECIFIED.);
#430=B_SPLINE_CURVE_WITH_KNOTS('',3,(#38487,#38488,#38489,#38490,#38491,
#38492,#38493,#38494,#38495,#38496,#38497,#38498,#38499,#38500,#38501,#38502,
#38503,#38504,#38505,#38506,#38507,#38508,#38509,#38510,#38511,#38512,#38513,
#38514,#38515,#38516,#38517,#38518,#38519,#38520,#38521,#38522,#38523,#38524,
#38525,#38526,#38527,#38528,#38529,#38530,#38531,#38532,#38533,#38534,#38535),
 .UNSPECIFIED.,.F.,.F.,(4,3,3,3,3,3,3,3,3,3,3,3,3,3,3,3,4),(1.61418366015071E-7,
0.0927499019073366,0.125,0.216040617119944,0.25,0.341377377596209,0.375,
0.466360220727834,0.5,0.591360220727629,0.625,0.716377377596198,0.75,0.841040617119855,
0.875,0.967749741650065,1.),.UNSPECIFIED.);
#431=B_SPLINE_CURVE_WITH_KNOTS('',3,(#38537,#38538,#38539,#38540,#38541,
#38542,#38543,#38544,#38545,#38546,#38547,#38548,#38549,#38550,#38551,#38552,
#38553,#38554,#38555,#38556,#38557,#38558,#38559,#38560,#38561,#38562,#38563,
#38564,#38565,#38566,#38567,#38568,#38569,#38570,#38571,#38572,#38573,#38574,
#38575,#38576,#38577,#38578,#38579,#38580,#38581,#38582,#38583,#38584,#38585),
 .UNSPECIFIED.,.F.,.F.,(4,3,3,3,3,3,3,3,3,3,3,3,3,3,3,3,4),(0.,0.092769801779297,
0.125,0.216060985371345,0.25,0.341397739310444,0.375,0.466380546419268,
0.5,0.591380546419013,0.625,0.716397739310629,0.75,0.841060985371185,0.875,
0.967769801779509,1.),.UNSPECIFIED.);
#432=B_SPLINE_CURVE_WITH_KNOTS('',3,(#38587,#38588,#38589,#38590,#38591,
#38592,#38593,#38594,#38595,#38596,#38597,#38598,#38599,#38600,#38601,#38602,
#38603,#38604,#38605,#38606,#38607,#38608,#38609,#38610,#38611,#38612,#38613,
#38614,#38615,#38616,#38617,#38618,#38619,#38620,#38621,#38622,#38623,#38624,
#38625,#38626,#38627,#38628,#38629,#38630,#38631,#38632,#38633,#38634,#38635),
 .UNSPECIFIED.,.F.,.F.,(4,3,3,3,3,3,3,3,3,3,3,3,3,3,3,3,4),(0.,0.092760818757206,
0.125,0.216051864381934,0.25,0.341388621253046,0.375,0.466371444488478,
0.5,0.59137144448888,0.625,0.716388621253012,0.75,0.841051864382076,0.875,
0.967760818757123,1.),.UNSPECIFIED.);
#433=B_SPLINE_CURVE_WITH_KNOTS('',3,(#38637,#38638,#38639,#38640,#38641,
#38642,#38643,#38644,#38645,#38646,#38647,#38648,#38649,#38650,#38651,#38652,
#38653,#38654,#38655,#38656,#38657,#38658,#38659,#38660,#38661,#38662,#38663,
#38664,#38665,#38666,#38667,#38668,#38669,#38670,#38671,#38672,#38673,#38674,
#38675,#38676,#38677,#38678,#38679,#38680,#38681,#38682,#38683,#38684,#38685),
 .UNSPECIFIED.,.F.,.F.,(4,3,3,3,3,3,3,3,3,3,3,3,3,3,3,3,4),(1.25095121062788E-6,
0.0928811417084261,0.125,0.215904919700791,0.25,0.340703649733594,0.375,
0.472752790800904,0.5,0.58379655566272,0.625,0.717023923539693,0.75,0.841676781252664,
0.875,0.969038482526097,0.999998918721821),.UNSPECIFIED.);
#434=B_SPLINE_CURVE_WITH_KNOTS('',3,(#38687,#38688,#38689,#38690),
 .UNSPECIFIED.,.F.,.F.,(4,4),(0.,0.999999406830264),.UNSPECIFIED.);
#435=B_SPLINE_CURVE_WITH_KNOTS('',3,(#38693,#38694,#38695,#38696,#38697,
#38698,#38699,#38700,#38701,#38702,#38703,#38704,#38705,#38706,#38707,#38708,
#38709,#38710,#38711,#38712,#38713,#38714,#38715,#38716,#38717,#38718,#38719,
#38720,#38721,#38722,#38723,#38724,#38725,#38726,#38727,#38728,#38729,#38730,
#38731,#38732,#38733,#38734,#38735,#38736,#38737,#38738,#38739,#38740,#38741),
 .UNSPECIFIED.,.F.,.F.,(4,3,3,3,3,3,3,3,3,3,3,3,3,3,3,3,4),(5.35569051418317E-13,
0.118460071640814,0.125,0.24207917943708,0.25,0.367390315276668,0.375,0.492346910740242,
0.5,0.617346910740273,0.625,0.742390315276672,0.75,0.867079179437042,0.875,
0.993460071640304,1.),.UNSPECIFIED.);
#436=B_SPLINE_CURVE_WITH_KNOTS('',3,(#38745,#38746,#38747,#38748,#38749,
#38750,#38751,#38752,#38753,#38754,#38755,#38756,#38757,#38758,#38759,#38760,
#38761,#38762,#38763,#38764,#38765,#38766,#38767,#38768,#38769,#38770,#38771,
#38772,#38773,#38774,#38775,#38776,#38777,#38778,#38779,#38780,#38781,#38782,
#38783,#38784,#38785,#38786,#38787,#38788,#38789,#38790,#38791,#38792,#38793),
 .UNSPECIFIED.,.F.,.F.,(4,3,3,3,3,3,3,3,3,3,3,3,3,3,3,3,4),(0.,0.0886362384441663,
0.125,0.212003562124013,0.25,0.337325311248101,0.375,0.462308884423835,
0.5,0.587308884423828,0.625,0.712325311248107,0.75,0.837003562124003,0.875,
0.963636238444181,1.),.UNSPECIFIED.);
#437=B_SPLINE_CURVE_WITH_KNOTS('',3,(#38795,#38796,#38797,#38798,#38799,
#38800,#38801,#38802,#38803,#38804,#38805,#38806,#38807,#38808,#38809,#38810,
#38811,#38812,#38813,#38814,#38815,#38816,#38817,#38818,#38819,#38820,#38821,
#38822,#38823,#38824,#38825,#38826,#38827,#38828,#38829,#38830,#38831,#38832,
#38833,#38834,#38835,#38836,#38837,#38838,#38839,#38840,#38841,#38842,#38843),
 .UNSPECIFIED.,.F.,.F.,(4,3,3,3,3,3,3,3,3,3,3,3,3,3,3,3,4),(0.,0.0886170904948371,
0.125,0.211984120063404,0.25,0.337305875427266,0.375,0.462289482987845,
0.5,0.58728948298785,0.625,0.712305875427259,0.75,0.836984120063407,0.875,
0.963617076466439,0.999999838308052),.UNSPECIFIED.);
#438=B_SPLINE_CURVE_WITH_KNOTS('',3,(#38845,#38846,#38847,#38848,#38849,
#38850,#38851,#38852,#38853,#38854,#38855,#38856,#38857,#38858,#38859,#38860,
#38861,#38862,#38863,#38864,#38865,#38866,#38867,#38868,#38869),
 .UNSPECIFIED.,.F.,.F.,(4,3,3,3,3,3,3,3,4),(0.,0.209718158421766,0.25,0.456937946730344,
0.5,0.70693794673032,0.75,0.959718158421781,1.),.UNSPECIFIED.);
#439=B_SPLINE_CURVE_WITH_KNOTS('',3,(#38873,#38874,#38875,#38876,#38877,
#38878,#38879,#38880,#38881,#38882),.UNSPECIFIED.,.F.,.F.,(4,2,2,2,4),(1.2249654638409E-12,
0.291982900699211,0.5,0.791982900697973,1.),.UNSPECIFIED.);
#440=B_SPLINE_CURVE_WITH_KNOTS('',3,(#38884,#38885,#38886,#38887,#38888,
#38889,#38890,#38891,#38892,#38893,#38894,#38895,#38896,#38897,#38898,#38899,
#38900,#38901,#38902,#38903,#38904,#38905,#38906,#38907,#38908,#38909,#38910,
#38911,#38912,#38913,#38914,#38915,#38916,#38917,#38918,#38919,#38920,#38921,
#38922,#38923,#38924,#38925,#38926,#38927,#38928,#38929,#38930,#38931,#38932),
 .UNSPECIFIED.,.F.,.F.,(4,3,3,3,3,3,3,3,3,3,3,3,3,3,3,3,4),(0.,0.0886392611603209,
0.125,0.212006631260798,0.25,0.337328379396744,0.375,0.462311947147395,
0.5,0.587311947147404,0.625,0.712328379396739,0.75,0.837006631260799,0.875,
0.963639261160282,1.),.UNSPECIFIED.);
#441=B_SPLINE_CURVE_WITH_KNOTS('',3,(#38934,#38935,#38936,#38937,#38938,
#38939,#38940,#38941,#38942,#38943,#38944,#38945,#38946,#38947,#38948,#38949,
#38950,#38951,#38952,#38953,#38954,#38955,#38956,#38957,#38958,#38959,#38960,
#38961,#38962,#38963,#38964,#38965,#38966,#38967,#38968,#38969,#38970,#38971,
#38972,#38973,#38974,#38975,#38976,#38977,#38978,#38979,#38980,#38981,#38982),
 .UNSPECIFIED.,.F.,.F.,(4,3,3,3,3,3,3,3,3,3,3,3,3,3,3,3,4),(0.,0.0886201162472742,
0.125,0.211987192297148,0.25,0.337308946677277,0.375,0.462292548802212,
0.5,0.587292548802218,0.625,0.712308946677277,0.75,0.836987192297145,0.875,
0.963620116247306,1.),.UNSPECIFIED.);
#442=B_SPLINE_CURVE_WITH_KNOTS('',3,(#38984,#38985,#38986,#38987,#38988,
#38989,#38990,#38991,#38992,#38993,#38994,#38995,#38996,#38997,#38998,#38999,
#39000,#39001,#39002,#39003,#39004,#39005,#39006,#39007,#39008,#39009,#39010,
#39011,#39012,#39013,#39014,#39015,#39016,#39017,#39018,#39019,#39020,#39021,
#39022,#39023,#39024,#39025,#39026,#39027,#39028,#39029,#39030,#39031,#39032),
 .UNSPECIFIED.,.F.,.F.,(4,3,3,3,3,3,3,3,3,3,3,3,3,3,3,3,4),(5.05515188767001E-7,
0.0886110104715978,0.125,0.211979068662331,0.25,0.337305561024299,0.375,
0.462245638602086,0.5,0.587333292602463,0.625,0.712306032467428,0.75,0.836989026938191,
0.875,0.963623466963222,0.99999974561912),.UNSPECIFIED.);
#443=B_SPLINE_CURVE_WITH_KNOTS('',3,(#39034,#39035,#39036,#39037,#39038,
#39039,#39040,#39041,#39042,#39043,#39044,#39045,#39046,#39047,#39048,#39049,
#39050,#39051,#39052,#39053,#39054,#39055,#39056,#39057,#39058,#39059,#39060,
#39061,#39062,#39063,#39064,#39065,#39066,#39067,#39068,#39069,#39070,#39071,
#39072,#39073,#39074,#39075,#39076,#39077,#39078,#39079,#39080,#39081,#39082),
 .UNSPECIFIED.,.F.,.F.,(4,3,3,3,3,3,3,3,3,3,3,3,3,3,3,3,4),(0.,0.0886344285884905,
0.125,0.212001724472824,0.25,0.337323474188171,0.375,0.462307050612556,
0.5,0.587307050612541,0.625,0.712323474188171,0.75,0.837001724472838,0.875,
0.963634428588436,1.),.UNSPECIFIED.);
#444=B_SPLINE_CURVE_WITH_KNOTS('',3,(#39084,#39085,#39086,#39087,#39088,
#39089,#39090,#39091,#39092,#39093,#39094,#39095,#39096,#39097,#39098,#39099,
#39100,#39101,#39102,#39103,#39104,#39105,#39106,#39107,#39108),
 .UNSPECIFIED.,.F.,.F.,(4,3,3,3,3,3,3,3,4),(0.,0.177329485747707,0.25,0.424060419200447,
0.5,0.674060419200489,0.75,0.927329485747577,1.),.UNSPECIFIED.);
#445=B_SPLINE_CURVE_WITH_KNOTS('',3,(#39112,#39113,#39114,#39115,#39116,
#39117,#39118),.UNSPECIFIED.,.F.,.F.,(4,1,1,1,4),(0.,0.25,0.5,0.75,1.),
 .UNSPECIFIED.);
#446=B_SPLINE_CURVE_WITH_KNOTS('',3,(#39120,#39121,#39122,#39123,#39124,
#39125,#39126,#39127,#39128,#39129,#39130,#39131,#39132,#39133,#39134,#39135,
#39136,#39137,#39138,#39139,#39140,#39141,#39142,#39143,#39144,#39145,#39146,
#39147,#39148,#39149,#39150,#39151,#39152,#39153,#39154,#39155,#39156,#39157,
#39158,#39159,#39160,#39161,#39162,#39163,#39164,#39165,#39166,#39167,#39168,
#39169,#39170,#39171,#39172,#39173,#39174,#39175,#39176,#39177,#39178,#39179,
#39180,#39181,#39182,#39183,#39184,#39185,#39186),.UNSPECIFIED.,.F.,.F.,
(4,3,3,3,3,3,3,3,3,3,3,3,3,3,3,3,3,3,3,3,3,3,4),(1.06075131901111E-6,0.0884946396841923,
0.102026634743488,0.125,0.212110420183879,0.25,0.261096997261559,0.337989428361259,
0.375,0.420019583798184,0.457713536375547,0.5,0.580296494461757,0.599118987891557,
0.625,0.711607136294009,0.740646741453979,0.75,0.836347955298163,0.875,
0.898862893862905,0.962328567718677,0.999998772366922),.UNSPECIFIED.);
#447=B_SPLINE_CURVE_WITH_KNOTS('',3,(#39187,#39188,#39189,#39190,#39191,
#39192,#39193,#39194,#39195,#39196,#39197,#39198,#39199,#39200,#39201,#39202,
#39203,#39204,#39205,#39206,#39207,#39208,#39209,#39210,#39211,#39212,#39213,
#39214,#39215,#39216,#39217,#39218,#39219,#39220,#39221,#39222,#39223,#39224,
#39225,#39226,#39227,#39228,#39229,#39230,#39231,#39232,#39233,#39234,#39235),
 .UNSPECIFIED.,.F.,.F.,(4,3,3,3,3,3,3,3,3,3,3,3,3,3,3,3,4),(0.,0.0886276628941314,
0.125,0.211994854865046,0.25,0.337316606787889,0.375,0.462300195359125,
0.5,0.587300195359111,0.625,0.712316606787894,0.75,0.836994854865049,0.875,
0.963627662894127,1.),.UNSPECIFIED.);
#448=B_SPLINE_CURVE_WITH_KNOTS('',3,(#39276,#39277,#39278,#39279,#39280,
#39281,#39282,#39283,#39284,#39285,#39286,#39287,#39288,#39289,#39290,#39291,
#39292,#39293,#39294,#39295,#39296,#39297,#39298,#39299,#39300,#39301,#39302,
#39303,#39304,#39305,#39306,#39307,#39308,#39309,#39310,#39311,#39312,#39313,
#39314,#39315),.UNSPECIFIED.,.F.,.F.,(4,3,3,3,3,3,3,3,3,3,3,3,3,4),(-0.499777858153212,
-0.47181324986483,-0.404411035114472,-0.399568579211665,-0.370348404118398,
-0.312287096243119,-0.306423970531928,-0.263103928856152,-0.205372645614112,
-0.199340068239674,-0.11676936673232,-0.101385295104661,-0.096217945588105,
0.),.UNSPECIFIED.);
#449=B_SPLINE_CURVE_WITH_KNOTS('',3,(#39316,#39317,#39318,#39319,#39320,
#39321,#39322,#39323,#39324,#39325,#39326,#39327,#39328,#39329,#39330,#39331,
#39332,#39333,#39334,#39335,#39336,#39337,#39338,#39339,#39340,#39341,#39342,
#39343,#39344,#39345,#39346,#39347,#39348,#39349,#39350,#39351,#39352,#39353,
#39354,#39355,#39356,#39357,#39358),.UNSPECIFIED.,.F.,.F.,(4,3,3,3,3,3,
3,3,3,3,3,3,3,3,4),(-0.503648702838967,-0.430770877953045,-0.423912464156221,
-0.414886975050139,-0.331929750071717,-0.32764763640537,-0.286137866472306,
-0.230749364089863,-0.225605706863336,-0.22120879272055,-0.117677069982424,
-0.111686767538004,-0.0817616813229237,-0.0223522743546254,0.),
 .UNSPECIFIED.);
#450=B_SPLINE_CURVE_WITH_KNOTS('',3,(#39628,#39629,#39630,#39631,#39632,
#39633),.UNSPECIFIED.,.F.,.F.,(4,2,4),(7.69181997283135E-5,0.00104275533486278,
0.00201241795641651),.UNSPECIFIED.);
#451=B_SPLINE_CURVE_WITH_KNOTS('',3,(#39634,#39635,#39636,#39637,#39638,
#39639,#39640,#39641,#39642,#39643,#39644,#39645,#39646,#39647,#39648,#39649,
#39650,#39651,#39652,#39653,#39654,#39655,#39656,#39657,#39658,#39659,#39660,
#39661,#39662,#39663,#39664,#39665,#39666,#39667,#39668,#39669,#39670,#39671,
#39672,#39673),.UNSPECIFIED.,.F.,.F.,(4,3,3,3,3,3,3,3,3,3,3,3,3,4),(0.,
0.0959833697741033,0.101972206699614,0.195587298215562,0.206341771970019,
0.216827129531729,0.271561541990413,0.3003318498953,0.306853038549853,0.312555564896745,
0.399722509461884,0.404649475313381,0.493811083623272,0.501724005229504),
 .UNSPECIFIED.);
#452=B_SPLINE_CURVE_WITH_KNOTS('',3,(#39942,#39943,#39944,#39945,#39946,
#39947,#39948,#39949,#39950,#39951,#39952,#39953,#39954,#39955,#39956,#39957,
#39958,#39959,#39960,#39961,#39962,#39963,#39964,#39965,#39966,#39967,#39968,
#39969,#39970,#39971,#39972,#39973,#39974,#39975,#39976,#39977,#39978,#39979,
#39980,#39981,#39982,#39983,#39984,#39985,#39986,#39987,#39988,#39989,#39990,
#39991,#39992,#39993,#39994,#39995,#39996,#39997,#39998,#39999),
 .UNSPECIFIED.,.F.,.F.,(4,3,3,3,3,3,3,3,3,3,3,3,3,3,3,3,3,3,3,4),(0.000189315453215585,
0.0299594922632419,0.108460134023621,0.114084312282721,0.118341445248336,
0.223026221099152,0.228346490943163,0.239675938105935,0.322886901748949,
0.329558994731095,0.33493041280197,0.389982815414618,0.404828322990172,
0.413165778692639,0.418170476314411,0.422544813989412,0.449072712381233,
0.476360707610091,0.50168871402095,0.503648702838949),.UNSPECIFIED.);
#453=B_SPLINE_CURVE_WITH_KNOTS('',3,(#40145,#40146,#40147,#40148,#40149,
#40150,#40151,#40152,#40153,#40154,#40155,#40156,#40157,#40158,#40159,#40160,
#40161,#40162,#40163,#40164,#40165,#40166,#40167,#40168,#40169,#40170,#40171,
#40172,#40173,#40174,#40175,#40176,#40177,#40178,#40179,#40180,#40181,#40182,
#40183,#40184,#40185,#40186,#40187,#40188,#40189,#40190),.UNSPECIFIED.,
 .F.,.F.,(4,3,3,3,3,3,3,3,3,3,3,3,3,3,3,4),(9.88255891804216E-5,0.0299029135328962,
0.117771907894534,0.147638843125062,0.220655384964364,0.224985986036839,
0.229406390499783,0.237239648816644,0.328742913474894,0.334897242635998,
0.404790741220614,0.413084719440826,0.418385494722407,0.42240987867637,
0.501611305817306,0.503648702838969),.UNSPECIFIED.);
#454=B_SPLINE_CURVE_WITH_KNOTS('',3,(#40191,#40192,#40193,#40194,#40195,
#40196,#40197,#40198,#40199,#40200,#40201,#40202,#40203,#40204,#40205,#40206,
#40207,#40208,#40209,#40210,#40211,#40212,#40213,#40214,#40215,#40216,#40217,
#40218,#40219,#40220,#40221,#40222,#40223,#40224,#40225,#40226,#40227,#40228,
#40229,#40230,#40231,#40232,#40233),.UNSPECIFIED.,.F.,.F.,(4,3,3,3,3,3,
3,3,3,3,3,3,3,3,4),(-0.503648702838958,-0.429930161153392,-0.422397062002223,
-0.416091587548294,-0.333112845076983,-0.328793934021496,-0.300414695296256,
-0.288538996878268,-0.233218025246608,-0.227649042762086,-0.222314267218344,
-0.11882824439468,-0.11430518334793,-0.0249444678531058,0.),
 .UNSPECIFIED.);
#455=B_SPLINE_CURVE_WITH_KNOTS('',3,(#40237,#40238,#40239,#40240,#40241,
#40242,#40243,#40244,#40245,#40246,#40247,#40248,#40249,#40250,#40251,#40252,
#40253,#40254,#40255,#40256,#40257,#40258,#40259,#40260,#40261,#40262,#40263,
#40264,#40265,#40266,#40267,#40268,#40269,#40270,#40271,#40272,#40273,#40274,
#40275,#40276,#40277,#40278,#40279,#40280,#40281,#40282),.UNSPECIFIED.,
 .F.,.F.,(4,3,3,3,3,3,3,3,3,3,3,3,3,3,3,4),(-0.500212455550078,-0.471794247742062,
-0.409627241063031,-0.404584739756394,-0.39961108596175,-0.322820829274765,
-0.311856171421863,-0.26553693014911,-0.207517702253279,-0.202680435589951,
-0.198239983473561,-0.107350009536642,-0.100409420181077,-0.0696937723003933,
-0.0181002222704456,0.),.UNSPECIFIED.);
#456=B_SPLINE_CURVE_WITH_KNOTS('',3,(#40424,#40425,#40426,#40427,#40428,
#40429,#40430,#40431,#40432,#40433,#40434,#40435,#40436,#40437,#40438,#40439,
#40440,#40441,#40442,#40443,#40444,#40445,#40446,#40447,#40448,#40449,#40450,
#40451,#40452,#40453,#40454,#40455,#40456,#40457,#40458,#40459,#40460,#40461,
#40462,#40463),.UNSPECIFIED.,.F.,.F.,(4,3,3,3,3,3,3,3,3,3,3,3,3,4),(0.,
0.0979252393519714,0.101981016086327,0.186131114719788,0.194303776652966,
0.201330780004315,0.205068643612296,0.214441627415338,0.396886032890214,
0.402513654010981,0.407314608904017,0.437254927315218,0.49643612517153,
0.501724005229503),.UNSPECIFIED.);
#639=CONICAL_SURFACE('',#10635,0.0011,0.785398163397448);
#640=CONICAL_SURFACE('',#10642,0.0022,0.785398163397448);
#641=CONICAL_SURFACE('',#10649,0.00155,0.832981266674431);
#642=CONICAL_SURFACE('',#10650,0.00265,0.785398163397448);
#643=CONICAL_SURFACE('',#10657,0.0029,0.785398163397448);
#644=CONICAL_SURFACE('',#10665,0.0029,0.785398163397449);
#748=FACE_BOUND('',#1977,.T.);
#749=FACE_BOUND('',#1980,.T.);
#750=FACE_BOUND('',#1990,.T.);
#751=FACE_BOUND('',#1995,.T.);
#752=FACE_BOUND('',#1998,.T.);
#791=SHAPE_REPRESENTATION_RELATIONSHIP('SRR','None',#50159,#811);
#811=ADVANCED_BREP_SHAPE_REPRESENTATION('',(#851),#50072);
#831=STYLED_ITEM('',(#50261),#851);
#851=MANIFOLD_SOLID_BREP('Body1',#9876);
#999=PLANE('',#10640);
#1000=PLANE('',#10645);
#1001=PLANE('',#10654);
#1002=PLANE('',#10659);
#1003=PLANE('',#10660);
#1004=PLANE('',#10663);
#1005=PLANE('',#10666);
#1391=FACE_OUTER_BOUND('',#1970,.T.);
#1392=FACE_OUTER_BOUND('',#1971,.T.);
#1393=FACE_OUTER_BOUND('',#1972,.T.);
#1394=FACE_OUTER_BOUND('',#1973,.T.);
#1395=FACE_OUTER_BOUND('',#1974,.T.);
#1396=FACE_OUTER_BOUND('',#1975,.T.);
#1397=FACE_OUTER_BOUND('',#1976,.T.);
#1398=FACE_OUTER_BOUND('',#1978,.T.);
#1399=FACE_OUTER_BOUND('',#1979,.T.);
#1400=FACE_OUTER_BOUND('',#1981,.T.);
#1401=FACE_OUTER_BOUND('',#1982,.T.);
#1402=FACE_OUTER_BOUND('',#1983,.T.);
#1403=FACE_OUTER_BOUND('',#1984,.T.);
#1404=FACE_OUTER_BOUND('',#1985,.T.);
#1405=FACE_OUTER_BOUND('',#1986,.T.);
#1406=FACE_OUTER_BOUND('',#1987,.T.);
#1407=FACE_OUTER_BOUND('',#1988,.T.);
#1408=FACE_OUTER_BOUND('',#1989,.T.);
#1409=FACE_OUTER_BOUND('',#1991,.T.);
#1410=FACE_OUTER_BOUND('',#1992,.T.);
#1411=FACE_OUTER_BOUND('',#1993,.T.);
#1412=FACE_OUTER_BOUND('',#1994,.T.);
#1413=FACE_OUTER_BOUND('',#1996,.T.);
#1414=FACE_OUTER_BOUND('',#1997,.T.);
#1415=FACE_OUTER_BOUND('',#1999,.T.);
#1970=EDGE_LOOP('',(#7758,#7759,#7760,#7761,#7762,#7763,#7764,#7765,#7766,
#7767,#7768,#7769,#7770,#7771,#7772,#7773,#7774,#7775,#7776,#7777,#7778,
#7779,#7780,#7781));
#1971=EDGE_LOOP('',(#7782,#7783,#7784,#7785,#7786,#7787,#7788,#7789,#7790,
#7791,#7792,#7793,#7794,#7795,#7796,#7797,#7798,#7799,#7800,#7801,#7802));
#1972=EDGE_LOOP('',(#7803,#7804,#7805,#7806,#7807,#7808,#7809,#7810,#7811,
#7812,#7813,#7814,#7815,#7816));
#1973=EDGE_LOOP('',(#7817,#7818,#7819,#7820,#7821,#7822,#7823,#7824,#7825,
#7826,#7827,#7828,#7829,#7830));
#1974=EDGE_LOOP('',(#7831,#7832,#7833,#7834));
#1975=EDGE_LOOP('',(#7835,#7836,#7837,#7838));
#1976=EDGE_LOOP('',(#7839));
#1977=EDGE_LOOP('',(#7840));
#1978=EDGE_LOOP('',(#7841,#7842,#7843,#7844));
#1979=EDGE_LOOP('',(#7845));
#1980=EDGE_LOOP('',(#7846));
#1981=EDGE_LOOP('',(#7847,#7848,#7849,#7850));
#1982=EDGE_LOOP('',(#7851,#7852,#7853,#7854));
#1983=EDGE_LOOP('',(#7855,#7856,#7857,#7858));
#1984=EDGE_LOOP('',(#7859,#7860,#7861,#7862));
#1985=EDGE_LOOP('',(#7863,#7864,#7865,#7866,#7867));
#1986=EDGE_LOOP('',(#7868,#7869,#7870,#7871,#7872,#7873,#7874,#7875,#7876,
#7877,#7878,#7879,#7880,#7881,#7882,#7883,#7884,#7885,#7886,#7887,#7888,
#7889,#7890,#7891,#7892));
#1987=EDGE_LOOP('',(#7893,#7894,#7895,#7896,#7897,#7898,#7899,#7900,#7901,
#7902,#7903,#7904,#7905,#7906,#7907,#7908,#7909,#7910,#7911));
#1988=EDGE_LOOP('',(#7912,#7913,#7914,#7915,#7916,#7917,#7918));
#1989=EDGE_LOOP('',(#7919));
#1990=EDGE_LOOP('',(#7920));
#1991=EDGE_LOOP('',(#7921,#7922,#7923,#7924,#7925,#7926,#7927,#7928,#7929,
#7930,#7931,#7932,#7933,#7934));
#1992=EDGE_LOOP('',(#7935,#7936,#7937,#7938,#7939));
#1993=EDGE_LOOP('',(#7940,#7941,#7942,#7943,#7944,#7945,#7946,#7947,#7948,
#7949,#7950,#7951,#7952,#7953));
#1994=EDGE_LOOP('',(#7954,#7955,#7956,#7957));
#1995=EDGE_LOOP('',(#7958));
#1996=EDGE_LOOP('',(#7959,#7960,#7961,#7962,#7963,#7964));
#1997=EDGE_LOOP('',(#7965,#7966,#7967,#7968));
#1998=EDGE_LOOP('',(#7969));
#1999=EDGE_LOOP('',(#7970,#7971,#7972,#7973));
#2523=LINE('',#39240,#3101);
#2524=LINE('',#39245,#3102);
#2525=LINE('',#39253,#3103);
#2526=LINE('',#39260,#3104);
#2527=LINE('',#39263,#3105);
#2528=LINE('',#39267,#3106);
#2529=LINE('',#39270,#3107);
#2530=LINE('',#40002,#3108);
#2531=LINE('',#40468,#3109);
#2532=LINE('',#40473,#3110);
#3101=VECTOR('',#12377,0.0011);
#3102=VECTOR('',#12384,0.001);
#3103=VECTOR('',#12393,0.0022);
#3104=VECTOR('',#12402,0.0021);
#3105=VECTOR('',#12407,0.00155);
#3106=VECTOR('',#12412,0.00265);
#3107=VECTOR('',#12415,0.00275);
#3108=VECTOR('',#12426,0.0029);
#3109=VECTOR('',#12443,0.0029);
#3110=VECTOR('',#12450,0.001475);
#3601=CIRCLE('',#10622,0.00251045773724889);
#3602=CIRCLE('',#10623,0.00250000000001);
#3603=CIRCLE('',#10624,0.00250000000001);
#3604=CIRCLE('',#10626,0.00300000000001);
#3605=CIRCLE('',#10627,0.00300000000001);
#3606=CIRCLE('',#10629,0.00251044841467262);
#3607=CIRCLE('',#10630,0.00250000000001);
#3608=CIRCLE('',#10631,0.00250000000001);
#3609=CIRCLE('',#10633,0.00300000000001);
#3610=CIRCLE('',#10634,0.00300000000001);
#3611=CIRCLE('',#10636,0.00100000000001);
#3612=CIRCLE('',#10637,0.00120000000001);
#3613=CIRCLE('',#10639,0.00100000000001);
#3614=CIRCLE('',#10641,0.00280000000001);
#3615=CIRCLE('',#10643,0.00210000000001);
#3616=CIRCLE('',#10644,0.00230000000001);
#3617=CIRCLE('',#10646,0.00255000000001);
#3618=CIRCLE('',#10648,0.00210000000001);
#3619=CIRCLE('',#10651,0.00275000000001);
#3620=CIRCLE('',#10653,0.00275000000001);
#3621=CIRCLE('',#10655,0.00300000000001);
#3622=CIRCLE('',#10656,0.00300000000001);
#3623=CIRCLE('',#10658,0.00280000000001);
#3624=CIRCLE('',#10661,0.00300000000001);
#3625=CIRCLE('',#10662,0.00300000000001);
#3626=CIRCLE('',#10664,0.00147500000001);
#3627=CIRCLE('',#10667,0.00147500000001);
#4295=VERTEX_POINT('',#34788);
#4296=VERTEX_POINT('',#34789);
#4297=VERTEX_POINT('',#34839);
#4298=VERTEX_POINT('',#34895);
#4299=VERTEX_POINT('',#34945);
#4300=VERTEX_POINT('',#34995);
#4301=VERTEX_POINT('',#35072);
#4302=VERTEX_POINT('',#35122);
#4303=VERTEX_POINT('',#35172);
#4304=VERTEX_POINT('',#35222);
#4305=VERTEX_POINT('',#35272);
#4306=VERTEX_POINT('',#35274);
#4307=VERTEX_POINT('',#35276);
#4308=VERTEX_POINT('',#35302);
#4309=VERTEX_POINT('',#35352);
#4310=VERTEX_POINT('',#35402);
#4311=VERTEX_POINT('',#35455);
#4312=VERTEX_POINT('',#35505);
#4313=VERTEX_POINT('',#35555);
#4314=VERTEX_POINT('',#35644);
#4315=VERTEX_POINT('',#35694);
#4316=VERTEX_POINT('',#35744);
#4317=VERTEX_POINT('',#35779);
#4318=VERTEX_POINT('',#35784);
#4319=VERTEX_POINT('',#35836);
#4320=VERTEX_POINT('',#35837);
#4321=VERTEX_POINT('',#35887);
#4322=VERTEX_POINT('',#36834);
#4323=VERTEX_POINT('',#37225);
#4324=VERTEX_POINT('',#37328);
#4325=VERTEX_POINT('',#37330);
#4326=VERTEX_POINT('',#37338);
#4327=VERTEX_POINT('',#37430);
#4328=VERTEX_POINT('',#37480);
#4329=VERTEX_POINT('',#37530);
#4330=VERTEX_POINT('',#37580);
#4331=VERTEX_POINT('',#37630);
#4332=VERTEX_POINT('',#37680);
#4333=VERTEX_POINT('',#37730);
#4334=VERTEX_POINT('',#37780);
#4335=VERTEX_POINT('',#37830);
#4336=VERTEX_POINT('',#37853);
#4337=VERTEX_POINT('',#37855);
#4338=VERTEX_POINT('',#38202);
#4339=VERTEX_POINT('',#38210);
#4340=VERTEX_POINT('',#38211);
#4341=VERTEX_POINT('',#38261);
#4342=VERTEX_POINT('',#38371);
#4343=VERTEX_POINT('',#38421);
#4344=VERTEX_POINT('',#38456);
#4345=VERTEX_POINT('',#38458);
#4346=VERTEX_POINT('',#38460);
#4347=VERTEX_POINT('',#38486);
#4348=VERTEX_POINT('',#38536);
#4349=VERTEX_POINT('',#38586);
#4350=VERTEX_POINT('',#38636);
#4351=VERTEX_POINT('',#38686);
#4352=VERTEX_POINT('',#38691);
#4353=VERTEX_POINT('',#38743);
#4354=VERTEX_POINT('',#38744);
#4355=VERTEX_POINT('',#38794);
#4356=VERTEX_POINT('',#38844);
#4357=VERTEX_POINT('',#38870);
#4358=VERTEX_POINT('',#38872);
#4359=VERTEX_POINT('',#38883);
#4360=VERTEX_POINT('',#38933);
#4361=VERTEX_POINT('',#38983);
#4362=VERTEX_POINT('',#39033);
#4363=VERTEX_POINT('',#39083);
#4364=VERTEX_POINT('',#39109);
#4365=VERTEX_POINT('',#39111);
#4366=VERTEX_POINT('',#39119);
#4367=VERTEX_POINT('',#39237);
#4368=VERTEX_POINT('',#39239);
#4369=VERTEX_POINT('',#39243);
#4370=VERTEX_POINT('',#39247);
#4371=VERTEX_POINT('',#39250);
#4372=VERTEX_POINT('',#39252);
#4373=VERTEX_POINT('',#39256);
#4374=VERTEX_POINT('',#39259);
#4375=VERTEX_POINT('',#39265);
#4376=VERTEX_POINT('',#39269);
#4377=VERTEX_POINT('',#39273);
#4378=VERTEX_POINT('',#39274);
#4379=VERTEX_POINT('',#40001);
#4380=VERTEX_POINT('',#40235);
#4381=VERTEX_POINT('',#40465);
#4382=VERTEX_POINT('',#40470);
#5532=EDGE_CURVE('',#4295,#4296,#386,.T.);
#5533=EDGE_CURVE('',#4296,#4297,#387,.T.);
#5534=EDGE_CURVE('',#4297,#4298,#388,.T.);
#5535=EDGE_CURVE('',#4298,#4299,#389,.T.);
#5536=EDGE_CURVE('',#4299,#4300,#390,.T.);
#5537=EDGE_CURVE('',#4300,#4301,#391,.T.);
#5538=EDGE_CURVE('',#4301,#4302,#392,.T.);
#5539=EDGE_CURVE('',#4302,#4303,#393,.T.);
#5540=EDGE_CURVE('',#4303,#4304,#394,.T.);
#5541=EDGE_CURVE('',#4304,#4305,#3601,.T.);
#5542=EDGE_CURVE('',#4306,#4305,#3602,.T.);
#5543=EDGE_CURVE('',#4307,#4306,#395,.F.);
#5544=EDGE_CURVE('',#4308,#4307,#396,.F.);
#5545=EDGE_CURVE('',#4309,#4308,#397,.F.);
#5546=EDGE_CURVE('',#4310,#4309,#398,.F.);
#5547=EDGE_CURVE('',#4311,#4310,#399,.F.);
#5548=EDGE_CURVE('',#4312,#4311,#400,.F.);
#5549=EDGE_CURVE('',#4313,#4312,#401,.F.);
#5550=EDGE_CURVE('',#4314,#4313,#402,.F.);
#5551=EDGE_CURVE('',#4315,#4314,#403,.F.);
#5552=EDGE_CURVE('',#4316,#4315,#404,.F.);
#5553=EDGE_CURVE('',#4317,#4316,#405,.F.);
#5554=EDGE_CURVE('',#4318,#4317,#3603,.T.);
#5555=EDGE_CURVE('',#4318,#4295,#406,.T.);
#5556=EDGE_CURVE('',#4319,#4320,#407,.T.);
#5557=EDGE_CURVE('',#4320,#4321,#408,.T.);
#5558=EDGE_CURVE('',#4321,#4322,#409,.T.);
#5559=EDGE_CURVE('',#4322,#4323,#410,.T.);
#5560=EDGE_CURVE('',#4323,#4324,#3604,.T.);
#5561=EDGE_CURVE('',#4324,#4325,#411,.T.);
#5562=EDGE_CURVE('',#4325,#4326,#412,.T.);
#5563=EDGE_CURVE('',#4326,#4327,#413,.T.);
#5564=EDGE_CURVE('',#4327,#4328,#414,.T.);
#5565=EDGE_CURVE('',#4328,#4329,#415,.T.);
#5566=EDGE_CURVE('',#4329,#4330,#416,.T.);
#5567=EDGE_CURVE('',#4330,#4331,#417,.T.);
#5568=EDGE_CURVE('',#4331,#4332,#418,.T.);
#5569=EDGE_CURVE('',#4332,#4333,#419,.T.);
#5570=EDGE_CURVE('',#4333,#4334,#420,.T.);
#5571=EDGE_CURVE('',#4334,#4335,#421,.T.);
#5572=EDGE_CURVE('',#4336,#4335,#3605,.T.);
#5573=EDGE_CURVE('',#4336,#4337,#422,.T.);
#5574=EDGE_CURVE('',#4337,#4319,#423,.T.);
#5575=EDGE_CURVE('',#4319,#4338,#424,.T.);
#5576=EDGE_CURVE('',#4339,#4340,#425,.T.);
#5577=EDGE_CURVE('',#4340,#4341,#426,.T.);
#5578=EDGE_CURVE('',#4341,#4342,#427,.T.);
#5579=EDGE_CURVE('',#4342,#4343,#428,.T.);
#5580=EDGE_CURVE('',#4343,#4344,#3606,.T.);
#5581=EDGE_CURVE('',#4345,#4344,#3607,.T.);
#5582=EDGE_CURVE('',#4346,#4345,#429,.F.);
#5583=EDGE_CURVE('',#4347,#4346,#430,.F.);
#5584=EDGE_CURVE('',#4348,#4347,#431,.F.);
#5585=EDGE_CURVE('',#4349,#4348,#432,.F.);
#5586=EDGE_CURVE('',#4350,#4349,#433,.F.);
#5587=EDGE_CURVE('',#4351,#4350,#434,.F.);
#5588=EDGE_CURVE('',#4352,#4351,#3608,.T.);
#5589=EDGE_CURVE('',#4352,#4339,#435,.T.);
#5590=EDGE_CURVE('',#4353,#4354,#436,.T.);
#5591=EDGE_CURVE('',#4354,#4355,#437,.T.);
#5592=EDGE_CURVE('',#4355,#4356,#438,.T.);
#5593=EDGE_CURVE('',#4357,#4356,#3609,.T.);
#5594=EDGE_CURVE('',#4357,#4358,#439,.T.);
#5595=EDGE_CURVE('',#4358,#4359,#440,.T.);
#5596=EDGE_CURVE('',#4359,#4360,#441,.T.);
#5597=EDGE_CURVE('',#4360,#4361,#442,.T.);
#5598=EDGE_CURVE('',#4361,#4362,#443,.T.);
#5599=EDGE_CURVE('',#4362,#4363,#444,.T.);
#5600=EDGE_CURVE('',#4364,#4363,#3610,.T.);
#5601=EDGE_CURVE('',#4364,#4365,#445,.T.);
#5602=EDGE_CURVE('',#4365,#4366,#446,.T.);
#5603=EDGE_CURVE('',#4366,#4353,#447,.T.);
#5604=EDGE_CURVE('',#4367,#4367,#3611,.T.);
#5605=EDGE_CURVE('',#4367,#4368,#2523,.T.);
#5606=EDGE_CURVE('',#4368,#4368,#3612,.T.);
#5607=EDGE_CURVE('',#4369,#4369,#3613,.T.);
#5608=EDGE_CURVE('',#4369,#4367,#2524,.T.);
#5609=EDGE_CURVE('',#4370,#4370,#3614,.T.);
#5610=EDGE_CURVE('',#4371,#4371,#3615,.T.);
#5611=EDGE_CURVE('',#4371,#4372,#2525,.T.);
#5612=EDGE_CURVE('',#4372,#4372,#3616,.T.);
#5613=EDGE_CURVE('',#4373,#4373,#3617,.T.);
#5614=EDGE_CURVE('',#4371,#4374,#2526,.T.);
#5615=EDGE_CURVE('',#4374,#4374,#3618,.T.);
#5616=EDGE_CURVE('',#4369,#4374,#2527,.T.);
#5617=EDGE_CURVE('',#4375,#4375,#3619,.T.);
#5618=EDGE_CURVE('',#4375,#4373,#2528,.T.);
#5619=EDGE_CURVE('',#4375,#4376,#2529,.T.);
#5620=EDGE_CURVE('',#4376,#4376,#3620,.T.);
#5621=EDGE_CURVE('',#4377,#4378,#3621,.T.);
#5622=EDGE_CURVE('',#4377,#4306,#448,.T.);
#5623=EDGE_CURVE('',#4305,#4336,#449,.T.);
#5624=EDGE_CURVE('',#4378,#4336,#3622,.T.);
#5625=EDGE_CURVE('',#4335,#4377,#450,.T.);
#5626=EDGE_CURVE('',#4317,#4324,#451,.T.);
#5627=EDGE_CURVE('',#4323,#4318,#452,.T.);
#5628=EDGE_CURVE('',#4378,#4379,#2530,.T.);
#5629=EDGE_CURVE('',#4379,#4379,#3623,.T.);
#5630=EDGE_CURVE('',#4356,#4345,#453,.T.);
#5631=EDGE_CURVE('',#4351,#4364,#454,.T.);
#5632=EDGE_CURVE('',#4363,#4380,#3624,.T.);
#5633=EDGE_CURVE('',#4363,#4352,#455,.T.);
#5634=EDGE_CURVE('',#4380,#4364,#3625,.T.);
#5635=EDGE_CURVE('',#4344,#4357,#456,.T.);
#5636=EDGE_CURVE('',#4381,#4381,#3626,.T.);
#5637=EDGE_CURVE('',#4380,#4370,#2531,.T.);
#5638=EDGE_CURVE('',#4382,#4382,#3627,.T.);
#5639=EDGE_CURVE('',#4382,#4381,#2532,.T.);
#7758=ORIENTED_EDGE('',*,*,#5532,.T.);
#7759=ORIENTED_EDGE('',*,*,#5533,.T.);
#7760=ORIENTED_EDGE('',*,*,#5534,.T.);
#7761=ORIENTED_EDGE('',*,*,#5535,.T.);
#7762=ORIENTED_EDGE('',*,*,#5536,.T.);
#7763=ORIENTED_EDGE('',*,*,#5537,.T.);
#7764=ORIENTED_EDGE('',*,*,#5538,.T.);
#7765=ORIENTED_EDGE('',*,*,#5539,.T.);
#7766=ORIENTED_EDGE('',*,*,#5540,.T.);
#7767=ORIENTED_EDGE('',*,*,#5541,.T.);
#7768=ORIENTED_EDGE('',*,*,#5542,.F.);
#7769=ORIENTED_EDGE('',*,*,#5543,.F.);
#7770=ORIENTED_EDGE('',*,*,#5544,.F.);
#7771=ORIENTED_EDGE('',*,*,#5545,.F.);
#7772=ORIENTED_EDGE('',*,*,#5546,.F.);
#7773=ORIENTED_EDGE('',*,*,#5547,.F.);
#7774=ORIENTED_EDGE('',*,*,#5548,.F.);
#7775=ORIENTED_EDGE('',*,*,#5549,.F.);
#7776=ORIENTED_EDGE('',*,*,#5550,.F.);
#7777=ORIENTED_EDGE('',*,*,#5551,.F.);
#7778=ORIENTED_EDGE('',*,*,#5552,.F.);
#7779=ORIENTED_EDGE('',*,*,#5553,.F.);
#7780=ORIENTED_EDGE('',*,*,#5554,.F.);
#7781=ORIENTED_EDGE('',*,*,#5555,.T.);
#7782=ORIENTED_EDGE('',*,*,#5556,.T.);
#7783=ORIENTED_EDGE('',*,*,#5557,.T.);
#7784=ORIENTED_EDGE('',*,*,#5558,.T.);
#7785=ORIENTED_EDGE('',*,*,#5559,.T.);
#7786=ORIENTED_EDGE('',*,*,#5560,.T.);
#7787=ORIENTED_EDGE('',*,*,#5561,.T.);
#7788=ORIENTED_EDGE('',*,*,#5562,.T.);
#7789=ORIENTED_EDGE('',*,*,#5563,.T.);
#7790=ORIENTED_EDGE('',*,*,#5564,.T.);
#7791=ORIENTED_EDGE('',*,*,#5565,.T.);
#7792=ORIENTED_EDGE('',*,*,#5566,.T.);
#7793=ORIENTED_EDGE('',*,*,#5567,.T.);
#7794=ORIENTED_EDGE('',*,*,#5568,.T.);
#7795=ORIENTED_EDGE('',*,*,#5569,.T.);
#7796=ORIENTED_EDGE('',*,*,#5570,.T.);
#7797=ORIENTED_EDGE('',*,*,#5571,.T.);
#7798=ORIENTED_EDGE('',*,*,#5572,.F.);
#7799=ORIENTED_EDGE('',*,*,#5573,.T.);
#7800=ORIENTED_EDGE('',*,*,#5574,.T.);
#7801=ORIENTED_EDGE('',*,*,#5575,.T.);
#7802=ORIENTED_EDGE('',*,*,#5575,.F.);
#7803=ORIENTED_EDGE('',*,*,#5576,.T.);
#7804=ORIENTED_EDGE('',*,*,#5577,.T.);
#7805=ORIENTED_EDGE('',*,*,#5578,.T.);
#7806=ORIENTED_EDGE('',*,*,#5579,.T.);
#7807=ORIENTED_EDGE('',*,*,#5580,.T.);
#7808=ORIENTED_EDGE('',*,*,#5581,.F.);
#7809=ORIENTED_EDGE('',*,*,#5582,.F.);
#7810=ORIENTED_EDGE('',*,*,#5583,.F.);
#7811=ORIENTED_EDGE('',*,*,#5584,.F.);
#7812=ORIENTED_EDGE('',*,*,#5585,.F.);
#7813=ORIENTED_EDGE('',*,*,#5586,.F.);
#7814=ORIENTED_EDGE('',*,*,#5587,.F.);
#7815=ORIENTED_EDGE('',*,*,#5588,.F.);
#7816=ORIENTED_EDGE('',*,*,#5589,.T.);
#7817=ORIENTED_EDGE('',*,*,#5590,.T.);
#7818=ORIENTED_EDGE('',*,*,#5591,.T.);
#7819=ORIENTED_EDGE('',*,*,#5592,.T.);
#7820=ORIENTED_EDGE('',*,*,#5593,.F.);
#7821=ORIENTED_EDGE('',*,*,#5594,.T.);
#7822=ORIENTED_EDGE('',*,*,#5595,.T.);
#7823=ORIENTED_EDGE('',*,*,#5596,.T.);
#7824=ORIENTED_EDGE('',*,*,#5597,.T.);
#7825=ORIENTED_EDGE('',*,*,#5598,.T.);
#7826=ORIENTED_EDGE('',*,*,#5599,.T.);
#7827=ORIENTED_EDGE('',*,*,#5600,.F.);
#7828=ORIENTED_EDGE('',*,*,#5601,.T.);
#7829=ORIENTED_EDGE('',*,*,#5602,.T.);
#7830=ORIENTED_EDGE('',*,*,#5603,.T.);
#7831=ORIENTED_EDGE('',*,*,#5604,.T.);
#7832=ORIENTED_EDGE('',*,*,#5605,.T.);
#7833=ORIENTED_EDGE('',*,*,#5606,.T.);
#7834=ORIENTED_EDGE('',*,*,#5605,.F.);
#7835=ORIENTED_EDGE('',*,*,#5607,.F.);
#7836=ORIENTED_EDGE('',*,*,#5608,.T.);
#7837=ORIENTED_EDGE('',*,*,#5604,.F.);
#7838=ORIENTED_EDGE('',*,*,#5608,.F.);
#7839=ORIENTED_EDGE('',*,*,#5609,.F.);
#7840=ORIENTED_EDGE('',*,*,#5606,.F.);
#7841=ORIENTED_EDGE('',*,*,#5610,.T.);
#7842=ORIENTED_EDGE('',*,*,#5611,.T.);
#7843=ORIENTED_EDGE('',*,*,#5612,.T.);
#7844=ORIENTED_EDGE('',*,*,#5611,.F.);
#7845=ORIENTED_EDGE('',*,*,#5613,.F.);
#7846=ORIENTED_EDGE('',*,*,#5612,.F.);
#7847=ORIENTED_EDGE('',*,*,#5610,.F.);
#7848=ORIENTED_EDGE('',*,*,#5614,.T.);
#7849=ORIENTED_EDGE('',*,*,#5615,.T.);
#7850=ORIENTED_EDGE('',*,*,#5614,.F.);
#7851=ORIENTED_EDGE('',*,*,#5607,.T.);
#7852=ORIENTED_EDGE('',*,*,#5616,.T.);
#7853=ORIENTED_EDGE('',*,*,#5615,.F.);
#7854=ORIENTED_EDGE('',*,*,#5616,.F.);
#7855=ORIENTED_EDGE('',*,*,#5617,.T.);
#7856=ORIENTED_EDGE('',*,*,#5618,.T.);
#7857=ORIENTED_EDGE('',*,*,#5613,.T.);
#7858=ORIENTED_EDGE('',*,*,#5618,.F.);
#7859=ORIENTED_EDGE('',*,*,#5617,.F.);
#7860=ORIENTED_EDGE('',*,*,#5619,.T.);
#7861=ORIENTED_EDGE('',*,*,#5620,.F.);
#7862=ORIENTED_EDGE('',*,*,#5619,.F.);
#7863=ORIENTED_EDGE('',*,*,#5621,.F.);
#7864=ORIENTED_EDGE('',*,*,#5622,.T.);
#7865=ORIENTED_EDGE('',*,*,#5542,.T.);
#7866=ORIENTED_EDGE('',*,*,#5623,.T.);
#7867=ORIENTED_EDGE('',*,*,#5624,.F.);
#7868=ORIENTED_EDGE('',*,*,#5622,.F.);
#7869=ORIENTED_EDGE('',*,*,#5625,.F.);
#7870=ORIENTED_EDGE('',*,*,#5571,.F.);
#7871=ORIENTED_EDGE('',*,*,#5570,.F.);
#7872=ORIENTED_EDGE('',*,*,#5569,.F.);
#7873=ORIENTED_EDGE('',*,*,#5568,.F.);
#7874=ORIENTED_EDGE('',*,*,#5567,.F.);
#7875=ORIENTED_EDGE('',*,*,#5566,.F.);
#7876=ORIENTED_EDGE('',*,*,#5565,.F.);
#7877=ORIENTED_EDGE('',*,*,#5564,.F.);
#7878=ORIENTED_EDGE('',*,*,#5563,.F.);
#7879=ORIENTED_EDGE('',*,*,#5562,.F.);
#7880=ORIENTED_EDGE('',*,*,#5561,.F.);
#7881=ORIENTED_EDGE('',*,*,#5626,.F.);
#7882=ORIENTED_EDGE('',*,*,#5553,.T.);
#7883=ORIENTED_EDGE('',*,*,#5552,.T.);
#7884=ORIENTED_EDGE('',*,*,#5551,.T.);
#7885=ORIENTED_EDGE('',*,*,#5550,.T.);
#7886=ORIENTED_EDGE('',*,*,#5549,.T.);
#7887=ORIENTED_EDGE('',*,*,#5548,.T.);
#7888=ORIENTED_EDGE('',*,*,#5547,.T.);
#7889=ORIENTED_EDGE('',*,*,#5546,.T.);
#7890=ORIENTED_EDGE('',*,*,#5545,.T.);
#7891=ORIENTED_EDGE('',*,*,#5544,.T.);
#7892=ORIENTED_EDGE('',*,*,#5543,.T.);
#7893=ORIENTED_EDGE('',*,*,#5573,.F.);
#7894=ORIENTED_EDGE('',*,*,#5623,.F.);
#7895=ORIENTED_EDGE('',*,*,#5541,.F.);
#7896=ORIENTED_EDGE('',*,*,#5540,.F.);
#7897=ORIENTED_EDGE('',*,*,#5539,.F.);
#7898=ORIENTED_EDGE('',*,*,#5538,.F.);
#7899=ORIENTED_EDGE('',*,*,#5537,.F.);
#7900=ORIENTED_EDGE('',*,*,#5536,.F.);
#7901=ORIENTED_EDGE('',*,*,#5535,.F.);
#7902=ORIENTED_EDGE('',*,*,#5534,.F.);
#7903=ORIENTED_EDGE('',*,*,#5533,.F.);
#7904=ORIENTED_EDGE('',*,*,#5532,.F.);
#7905=ORIENTED_EDGE('',*,*,#5555,.F.);
#7906=ORIENTED_EDGE('',*,*,#5627,.F.);
#7907=ORIENTED_EDGE('',*,*,#5559,.F.);
#7908=ORIENTED_EDGE('',*,*,#5558,.F.);
#7909=ORIENTED_EDGE('',*,*,#5557,.F.);
#7910=ORIENTED_EDGE('',*,*,#5556,.F.);
#7911=ORIENTED_EDGE('',*,*,#5574,.F.);
#7912=ORIENTED_EDGE('',*,*,#5621,.T.);
#7913=ORIENTED_EDGE('',*,*,#5628,.T.);
#7914=ORIENTED_EDGE('',*,*,#5629,.T.);
#7915=ORIENTED_EDGE('',*,*,#5628,.F.);
#7916=ORIENTED_EDGE('',*,*,#5624,.T.);
#7917=ORIENTED_EDGE('',*,*,#5572,.T.);
#7918=ORIENTED_EDGE('',*,*,#5625,.T.);
#7919=ORIENTED_EDGE('',*,*,#5629,.F.);
#7920=ORIENTED_EDGE('',*,*,#5620,.T.);
#7921=ORIENTED_EDGE('',*,*,#5630,.F.);
#7922=ORIENTED_EDGE('',*,*,#5592,.F.);
#7923=ORIENTED_EDGE('',*,*,#5591,.F.);
#7924=ORIENTED_EDGE('',*,*,#5590,.F.);
#7925=ORIENTED_EDGE('',*,*,#5603,.F.);
#7926=ORIENTED_EDGE('',*,*,#5602,.F.);
#7927=ORIENTED_EDGE('',*,*,#5601,.F.);
#7928=ORIENTED_EDGE('',*,*,#5631,.F.);
#7929=ORIENTED_EDGE('',*,*,#5587,.T.);
#7930=ORIENTED_EDGE('',*,*,#5586,.T.);
#7931=ORIENTED_EDGE('',*,*,#5585,.T.);
#7932=ORIENTED_EDGE('',*,*,#5584,.T.);
#7933=ORIENTED_EDGE('',*,*,#5583,.T.);
#7934=ORIENTED_EDGE('',*,*,#5582,.T.);
#7935=ORIENTED_EDGE('',*,*,#5632,.F.);
#7936=ORIENTED_EDGE('',*,*,#5633,.T.);
#7937=ORIENTED_EDGE('',*,*,#5588,.T.);
#7938=ORIENTED_EDGE('',*,*,#5631,.T.);
#7939=ORIENTED_EDGE('',*,*,#5634,.F.);
#7940=ORIENTED_EDGE('',*,*,#5635,.F.);
#7941=ORIENTED_EDGE('',*,*,#5580,.F.);
#7942=ORIENTED_EDGE('',*,*,#5579,.F.);
#7943=ORIENTED_EDGE('',*,*,#5578,.F.);
#7944=ORIENTED_EDGE('',*,*,#5577,.F.);
#7945=ORIENTED_EDGE('',*,*,#5576,.F.);
#7946=ORIENTED_EDGE('',*,*,#5589,.F.);
#7947=ORIENTED_EDGE('',*,*,#5633,.F.);
#7948=ORIENTED_EDGE('',*,*,#5599,.F.);
#7949=ORIENTED_EDGE('',*,*,#5598,.F.);
#7950=ORIENTED_EDGE('',*,*,#5597,.F.);
#7951=ORIENTED_EDGE('',*,*,#5596,.F.);
#7952=ORIENTED_EDGE('',*,*,#5595,.F.);
#7953=ORIENTED_EDGE('',*,*,#5594,.F.);
#7954=ORIENTED_EDGE('',*,*,#5630,.T.);
#7955=ORIENTED_EDGE('',*,*,#5581,.T.);
#7956=ORIENTED_EDGE('',*,*,#5635,.T.);
#7957=ORIENTED_EDGE('',*,*,#5593,.T.);
#7958=ORIENTED_EDGE('',*,*,#5636,.T.);
#7959=ORIENTED_EDGE('',*,*,#5632,.T.);
#7960=ORIENTED_EDGE('',*,*,#5637,.T.);
#7961=ORIENTED_EDGE('',*,*,#5609,.T.);
#7962=ORIENTED_EDGE('',*,*,#5637,.F.);
#7963=ORIENTED_EDGE('',*,*,#5634,.T.);
#7964=ORIENTED_EDGE('',*,*,#5600,.T.);
#7965=ORIENTED_EDGE('',*,*,#5626,.T.);
#7966=ORIENTED_EDGE('',*,*,#5560,.F.);
#7967=ORIENTED_EDGE('',*,*,#5627,.T.);
#7968=ORIENTED_EDGE('',*,*,#5554,.T.);
#7969=ORIENTED_EDGE('',*,*,#5638,.T.);
#7970=ORIENTED_EDGE('',*,*,#5638,.F.);
#7971=ORIENTED_EDGE('',*,*,#5639,.T.);
#7972=ORIENTED_EDGE('',*,*,#5636,.F.);
#7973=ORIENTED_EDGE('',*,*,#5639,.F.);
#9242=CYLINDRICAL_SURFACE('',#10621,0.0025);
#9243=CYLINDRICAL_SURFACE('',#10625,0.003);
#9244=CYLINDRICAL_SURFACE('',#10628,0.0025);
#9245=CYLINDRICAL_SURFACE('',#10632,0.003);
#9246=CYLINDRICAL_SURFACE('',#10638,0.001);
#9247=CYLINDRICAL_SURFACE('',#10647,0.0021);
#9248=CYLINDRICAL_SURFACE('',#10652,0.00275);
#9249=CYLINDRICAL_SURFACE('',#10668,0.001475);
#9613=ADVANCED_FACE('',(#1391),#9242,.T.);
#9614=ADVANCED_FACE('',(#1392),#9243,.T.);
#9615=ADVANCED_FACE('',(#1393),#9244,.T.);
#9616=ADVANCED_FACE('',(#1394),#9245,.T.);
#9617=ADVANCED_FACE('',(#1395),#639,.F.);
#9618=ADVANCED_FACE('',(#1396),#9246,.F.);
#9619=ADVANCED_FACE('',(#1397,#748),#999,.F.);
#9620=ADVANCED_FACE('',(#1398),#640,.F.);
#9621=ADVANCED_FACE('',(#1399,#749),#1000,.T.);
#9622=ADVANCED_FACE('',(#1400),#9247,.F.);
#9623=ADVANCED_FACE('',(#1401),#641,.F.);
#9624=ADVANCED_FACE('',(#1402),#642,.T.);
#9625=ADVANCED_FACE('',(#1403),#9248,.T.);
#9626=ADVANCED_FACE('',(#1404),#1001,.F.);
#9627=ADVANCED_FACE('',(#1405),#106,.F.);
#9628=ADVANCED_FACE('',(#1406),#107,.F.);
#9629=ADVANCED_FACE('',(#1407),#643,.T.);
#9630=ADVANCED_FACE('',(#1408,#750),#1002,.T.);
#9631=ADVANCED_FACE('',(#1409),#108,.F.);
#9632=ADVANCED_FACE('',(#1410),#1003,.T.);
#9633=ADVANCED_FACE('',(#1411),#109,.F.);
#9634=ADVANCED_FACE('',(#1412,#751),#1004,.T.);
#9635=ADVANCED_FACE('',(#1413),#644,.T.);
#9636=ADVANCED_FACE('',(#1414,#752),#1005,.F.);
#9637=ADVANCED_FACE('',(#1415),#9249,.T.);
#9876=CLOSED_SHELL('',(#9613,#9614,#9615,#9616,#9617,#9618,#9619,#9620,
#9621,#9622,#9623,#9624,#9625,#9626,#9627,#9628,#9629,#9630,#9631,#9632,
#9633,#9634,#9635,#9636,#9637));
#10620=AXIS2_PLACEMENT_3D('',#34786,#12343,#12344);
#10621=AXIS2_PLACEMENT_3D('',#34787,#12345,#12346);
#10622=AXIS2_PLACEMENT_3D('',#35273,#12347,#12348);
#10623=AXIS2_PLACEMENT_3D('',#35275,#12349,#12350);
#10624=AXIS2_PLACEMENT_3D('',#35785,#12351,#12352);
#10625=AXIS2_PLACEMENT_3D('',#35835,#12353,#12354);
#10626=AXIS2_PLACEMENT_3D('',#37329,#12355,#12356);
#10627=AXIS2_PLACEMENT_3D('',#37854,#12357,#12358);
#10628=AXIS2_PLACEMENT_3D('',#38209,#12359,#12360);
#10629=AXIS2_PLACEMENT_3D('',#38457,#12361,#12362);
#10630=AXIS2_PLACEMENT_3D('',#38459,#12363,#12364);
#10631=AXIS2_PLACEMENT_3D('',#38692,#12365,#12366);
#10632=AXIS2_PLACEMENT_3D('',#38742,#12367,#12368);
#10633=AXIS2_PLACEMENT_3D('',#38871,#12369,#12370);
#10634=AXIS2_PLACEMENT_3D('',#39110,#12371,#12372);
#10635=AXIS2_PLACEMENT_3D('',#39236,#12373,#12374);
#10636=AXIS2_PLACEMENT_3D('',#39238,#12375,#12376);
#10637=AXIS2_PLACEMENT_3D('',#39241,#12378,#12379);
#10638=AXIS2_PLACEMENT_3D('',#39242,#12380,#12381);
#10639=AXIS2_PLACEMENT_3D('',#39244,#12382,#12383);
#10640=AXIS2_PLACEMENT_3D('',#39246,#12385,#12386);
#10641=AXIS2_PLACEMENT_3D('',#39248,#12387,#12388);
#10642=AXIS2_PLACEMENT_3D('',#39249,#12389,#12390);
#10643=AXIS2_PLACEMENT_3D('',#39251,#12391,#12392);
#10644=AXIS2_PLACEMENT_3D('',#39254,#12394,#12395);
#10645=AXIS2_PLACEMENT_3D('',#39255,#12396,#12397);
#10646=AXIS2_PLACEMENT_3D('',#39257,#12398,#12399);
#10647=AXIS2_PLACEMENT_3D('',#39258,#12400,#12401);
#10648=AXIS2_PLACEMENT_3D('',#39261,#12403,#12404);
#10649=AXIS2_PLACEMENT_3D('',#39262,#12405,#12406);
#10650=AXIS2_PLACEMENT_3D('',#39264,#12408,#12409);
#10651=AXIS2_PLACEMENT_3D('',#39266,#12410,#12411);
#10652=AXIS2_PLACEMENT_3D('',#39268,#12413,#12414);
#10653=AXIS2_PLACEMENT_3D('',#39271,#12416,#12417);
#10654=AXIS2_PLACEMENT_3D('',#39272,#12418,#12419);
#10655=AXIS2_PLACEMENT_3D('',#39275,#12420,#12421);
#10656=AXIS2_PLACEMENT_3D('',#39359,#12422,#12423);
#10657=AXIS2_PLACEMENT_3D('',#40000,#12424,#12425);
#10658=AXIS2_PLACEMENT_3D('',#40003,#12427,#12428);
#10659=AXIS2_PLACEMENT_3D('',#40004,#12429,#12430);
#10660=AXIS2_PLACEMENT_3D('',#40234,#12431,#12432);
#10661=AXIS2_PLACEMENT_3D('',#40236,#12433,#12434);
#10662=AXIS2_PLACEMENT_3D('',#40283,#12435,#12436);
#10663=AXIS2_PLACEMENT_3D('',#40464,#12437,#12438);
#10664=AXIS2_PLACEMENT_3D('',#40466,#12439,#12440);
#10665=AXIS2_PLACEMENT_3D('',#40467,#12441,#12442);
#10666=AXIS2_PLACEMENT_3D('',#40469,#12444,#12445);
#10667=AXIS2_PLACEMENT_3D('',#40471,#12446,#12447);
#10668=AXIS2_PLACEMENT_3D('',#40472,#12448,#12449);
#12343=DIRECTION('axis',(0.,0.,1.));
#12344=DIRECTION('refdir',(1.,0.,0.));
#12345=DIRECTION('center_axis',(0.,1.,0.));
#12346=DIRECTION('ref_axis',(-1.,0.,5.99795050356438E-14));
#12347=DIRECTION('center_axis',(0.00224230328468888,0.997965773468312,0.0637125345734545));
#12348=DIRECTION('ref_axis',(0.997534176097042,0.0022370021927377,-0.0701467272193514));
#12349=DIRECTION('center_axis',(0.,1.,0.));
#12350=DIRECTION('ref_axis',(-1.,0.,4.05997950501941E-12));
#12351=DIRECTION('center_axis',(0.,-1.,0.));
#12352=DIRECTION('ref_axis',(-1.,0.,4.05997950501941E-12));
#12353=DIRECTION('center_axis',(0.,1.,0.));
#12354=DIRECTION('ref_axis',(-1.,0.,0.));
#12355=DIRECTION('center_axis',(0.,1.,0.));
#12356=DIRECTION('ref_axis',(-1.,0.,0.));
#12357=DIRECTION('center_axis',(0.,1.,0.));
#12358=DIRECTION('ref_axis',(-1.,0.,0.));
#12359=DIRECTION('center_axis',(0.,1.,0.));
#12360=DIRECTION('ref_axis',(1.,0.,1.24958540118864E-14));
#12361=DIRECTION('center_axis',(-0.00223920793173383,0.997967529966866,
-0.063685124477159));
#12362=DIRECTION('ref_axis',(-0.997538864914972,0.00223390431455718,0.0700801159792351));
#12363=DIRECTION('center_axis',(0.,1.,0.));
#12364=DIRECTION('ref_axis',(1.,0.,4.01249585399583E-12));
#12365=DIRECTION('center_axis',(0.,-1.,0.));
#12366=DIRECTION('ref_axis',(1.,0.,4.01249585399583E-12));
#12367=DIRECTION('center_axis',(0.,1.,0.));
#12368=DIRECTION('ref_axis',(1.,0.,0.));
#12369=DIRECTION('center_axis',(0.,1.,0.));
#12370=DIRECTION('ref_axis',(1.,0.,0.));
#12371=DIRECTION('center_axis',(0.,-1.,0.));
#12372=DIRECTION('ref_axis',(1.,0.,0.));
#12373=DIRECTION('center_axis',(0.,-1.,0.));
#12374=DIRECTION('ref_axis',(-1.,0.,0.));
#12375=DIRECTION('center_axis',(0.,1.,0.));
#12376=DIRECTION('ref_axis',(-1.,0.,0.));
#12377=DIRECTION('',(0.707106781186547,-0.707106781186548,8.65956056235493E-17));
#12378=DIRECTION('center_axis',(0.,-1.,0.));
#12379=DIRECTION('ref_axis',(-1.,0.,0.));
#12380=DIRECTION('center_axis',(0.,-1.,0.));
#12381=DIRECTION('ref_axis',(-1.,0.,0.));
#12382=DIRECTION('center_axis',(0.,-1.,0.));
#12383=DIRECTION('ref_axis',(-1.,0.,0.));
#12384=DIRECTION('',(0.,-1.,0.));
#12385=DIRECTION('center_axis',(0.,1.,0.));
#12386=DIRECTION('ref_axis',(1.,0.,0.));
#12387=DIRECTION('center_axis',(0.,1.,0.));
#12388=DIRECTION('ref_axis',(1.,0.,0.));
#12389=DIRECTION('center_axis',(0.,1.,0.));
#12390=DIRECTION('ref_axis',(-1.,0.,0.));
#12391=DIRECTION('center_axis',(0.,-1.,0.));
#12392=DIRECTION('ref_axis',(-1.,0.,0.));
#12393=DIRECTION('',(0.707106781186547,0.707106781186548,-8.65956056235493E-17));
#12394=DIRECTION('center_axis',(0.,1.,0.));
#12395=DIRECTION('ref_axis',(-1.,0.,0.));
#12396=DIRECTION('center_axis',(0.,1.,0.));
#12397=DIRECTION('ref_axis',(1.,0.,0.));
#12398=DIRECTION('center_axis',(0.,-1.,0.));
#12399=DIRECTION('ref_axis',(-1.,0.,0.));
#12400=DIRECTION('center_axis',(0.,-1.,0.));
#12401=DIRECTION('ref_axis',(-1.,0.,0.));
#12402=DIRECTION('',(0.,-1.,0.));
#12403=DIRECTION('center_axis',(0.,-1.,0.));
#12404=DIRECTION('ref_axis',(-1.,0.,0.));
#12405=DIRECTION('center_axis',(0.,1.,0.));
#12406=DIRECTION('ref_axis',(-1.,0.,0.));
#12407=DIRECTION('',(0.739940073395943,0.672672793996313,-9.061652424452E-17));
#12408=DIRECTION('center_axis',(0.,-1.,0.));
#12409=DIRECTION('ref_axis',(-1.,0.,0.));
#12410=DIRECTION('center_axis',(0.,1.,0.));
#12411=DIRECTION('ref_axis',(-1.,0.,0.));
#12412=DIRECTION('',(-0.707106781186547,0.707106781186548,-8.65956056235493E-17));
#12413=DIRECTION('center_axis',(0.,1.,0.));
#12414=DIRECTION('ref_axis',(-1.,0.,0.));
#12415=DIRECTION('',(0.,-1.,0.));
#12416=DIRECTION('center_axis',(0.,-1.,0.));
#12417=DIRECTION('ref_axis',(-1.,0.,0.));
#12418=DIRECTION('center_axis',(0.,1.,0.));
#12419=DIRECTION('ref_axis',(1.,0.,0.));
#12420=DIRECTION('center_axis',(0.,1.,0.));
#12421=DIRECTION('ref_axis',(-1.,0.,0.));
#12422=DIRECTION('center_axis',(0.,1.,0.));
#12423=DIRECTION('ref_axis',(-1.,0.,0.));
#12424=DIRECTION('center_axis',(0.,-1.,0.));
#12425=DIRECTION('ref_axis',(-1.,0.,0.));
#12426=DIRECTION('',(-0.707106781186547,0.707106781186548,-8.65956056235493E-17));
#12427=DIRECTION('center_axis',(0.,-1.,0.));
#12428=DIRECTION('ref_axis',(-1.,0.,0.));
#12429=DIRECTION('center_axis',(0.,1.,0.));
#12430=DIRECTION('ref_axis',(1.,0.,0.));
#12431=DIRECTION('center_axis',(0.,1.,0.));
#12432=DIRECTION('ref_axis',(1.,0.,0.));
#12433=DIRECTION('center_axis',(0.,-1.,0.));
#12434=DIRECTION('ref_axis',(1.,0.,0.));
#12435=DIRECTION('center_axis',(0.,-1.,0.));
#12436=DIRECTION('ref_axis',(1.,0.,0.));
#12437=DIRECTION('center_axis',(0.,1.,0.));
#12438=DIRECTION('ref_axis',(1.,0.,0.));
#12439=DIRECTION('center_axis',(0.,-1.,0.));
#12440=DIRECTION('ref_axis',(-1.,0.,0.));
#12441=DIRECTION('center_axis',(0.,1.,0.));
#12442=DIRECTION('ref_axis',(1.,0.,0.));
#12443=DIRECTION('',(0.707106781186548,-0.707106781186547,-8.65956056235494E-17));
#12444=DIRECTION('center_axis',(0.,1.,0.));
#12445=DIRECTION('ref_axis',(1.,0.,0.));
#12446=DIRECTION('center_axis',(0.,1.,0.));
#12447=DIRECTION('ref_axis',(-1.,0.,0.));
#12448=DIRECTION('center_axis',(0.,1.,0.));
#12449=DIRECTION('ref_axis',(-1.,0.,0.));
#12450=DIRECTION('',(0.,-1.,0.));
#34786=CARTESIAN_POINT('',(0.,0.,0.));
#34787=CARTESIAN_POINT('Origin',(0.,-0.0288900992552775,-0.0121758532865581));
#34788=CARTESIAN_POINT('',(0.00249999999996746,-0.0263900992552675,-0.0121758405315141));
#34789=CARTESIAN_POINT('',(0.00249999969210765,-0.0253900438073696,-0.0121749724286797));
#34790=CARTESIAN_POINT('Ctrl Pts',(0.00249999999999986,-0.0263900983848402,
-0.0121758541222231));
#34791=CARTESIAN_POINT('Ctrl Pts',(0.0024999998376673,-0.0263591782252352,
-0.0126614929956707));
#34792=CARTESIAN_POINT('Ctrl Pts',(0.00235420814557946,-0.0263282580656303,
-0.0131471076179502));
#34793=CARTESIAN_POINT('Ctrl Pts',(0.00208694255055651,-0.0262973379060254,
-0.0135523236969472));
#34794=CARTESIAN_POINT('Ctrl Pts',(0.00199405292942151,-0.0262865914352314,
-0.013693158764224));
#34795=CARTESIAN_POINT('Ctrl Pts',(0.00188693836179305,-0.0262758449644375,
-0.0138244280014296));
#34796=CARTESIAN_POINT('Ctrl Pts',(0.00176792152173108,-0.0262650984936436,
-0.0139434656572435));
#34797=CARTESIAN_POINT('Ctrl Pts',(0.00143179056821086,-0.0262347479863283,
-0.0142796553992388));
#34798=CARTESIAN_POINT('Ctrl Pts',(0.000995395947558976,-0.0262043974790131,
-0.0145182192446305));
#34799=CARTESIAN_POINT('Ctrl Pts',(0.000529245665941188,-0.0261740469716978,
-0.0146191909679035));
#34800=CARTESIAN_POINT('Ctrl Pts',(0.00035544250978807,-0.0261627308486142,
-0.0146568380634414));
#34801=CARTESIAN_POINT('Ctrl Pts',(0.000177767476799881,-0.0261514147255306,
-0.0146758221771375));
#34802=CARTESIAN_POINT('Ctrl Pts',(4.38041264954561E-7,-0.026140098602447,
-0.0146758532481821));
#34803=CARTESIAN_POINT('Ctrl Pts',(-0.000476928978646773,-0.0261096358429109,
-0.0146759368907647));
#34804=CARTESIAN_POINT('Ctrl Pts',(-0.000955851385580713,-0.0260791730833748,
-0.0145349752078753));
#34805=CARTESIAN_POINT('Ctrl Pts',(-0.00135775933618906,-0.0260487103238387,
-0.0142750173070652));
#34806=CARTESIAN_POINT('Ctrl Pts',(-0.0015055766989595,-0.026037506452976,
-0.0141794076251195));
#34807=CARTESIAN_POINT('Ctrl Pts',(-0.00164311820444229,-0.0260263025821132,
-0.0140682035642993));
#34808=CARTESIAN_POINT('Ctrl Pts',(-0.00176730198346023,-0.0260150987112504,
-0.0139440850867635));
#34809=CARTESIAN_POINT('Ctrl Pts',(-0.00210488795169868,-0.0259846416771423,
-0.0136066766365892));
#34810=CARTESIAN_POINT('Ctrl Pts',(-0.0023438742147858,-0.0259541846430342,
-0.0131684597223472));
#34811=CARTESIAN_POINT('Ctrl Pts',(-0.00244431536234987,-0.025923727608926,
-0.0127005650258783));
#34812=CARTESIAN_POINT('Ctrl Pts',(-0.00248128234709218,-0.0259125180126353,
-0.0125283581512571));
#34813=CARTESIAN_POINT('Ctrl Pts',(-0.00249993823183487,-0.0259013084163446,
-0.0123523861710988));
#34814=CARTESIAN_POINT('Ctrl Pts',(-0.0024999998462029,-0.0258900988200539,
-0.0121767302047395));
#34815=CARTESIAN_POINT('Ctrl Pts',(-0.00250016725552431,-0.0258596417859458,
-0.0116994641534089));
#34816=CARTESIAN_POINT('Ctrl Pts',(-0.00235934708740709,-0.0258291847518377,
-0.0112206008805832));
#34817=CARTESIAN_POINT('Ctrl Pts',(-0.00209955019121586,-0.0257987277177296,
-0.0108186911759149));
#34818=CARTESIAN_POINT('Ctrl Pts',(-0.00200393292547784,-0.0257875181214388,
-0.0106707698281338));
#34819=CARTESIAN_POINT('Ctrl Pts',(-0.00189270211542129,-0.0257763085251481,
-0.0105331307828027));
#34820=CARTESIAN_POINT('Ctrl Pts',(-0.00176854202418612,-0.0257650989288573,
-0.0104088617447878));
#34821=CARTESIAN_POINT('Ctrl Pts',(-0.00143112942651921,-0.0257346361693212,
-0.0100711530776225));
#34822=CARTESIAN_POINT('Ctrl Pts',(-0.000992860182890661,-0.0257041734097852,
-0.00983206793845762));
#34823=CARTESIAN_POINT('Ctrl Pts',(-0.000524883444357732,-0.0256737106502491,
-0.00973157478977441));
#34824=CARTESIAN_POINT('Ctrl Pts',(-0.000352766701647285,-0.0256625067793863,
-0.00969461450523058));
#34825=CARTESIAN_POINT('Ctrl Pts',(-0.000176886159280237,-0.0256513029085235,
-0.00967594603868218));
#34826=CARTESIAN_POINT('Ctrl Pts',(-1.31579507085305E-6,-0.0256400990376607,
-0.00967585363282146));
#34827=CARTESIAN_POINT('Ctrl Pts',(0.000474292116562906,-0.0256097485303454,
-0.00967560331176847));
#34828=CARTESIAN_POINT('Ctrl Pts',(0.000951652707267703,-0.0255793980230303,
-0.00981539592066256));
#34829=CARTESIAN_POINT('Ctrl Pts',(0.00135268560133641,-0.0255490475157151,
-0.0100734162092744));
#34830=CARTESIAN_POINT('Ctrl Pts',(0.00150220987593061,-0.0255377313926314,
-0.0101696185334625));
#34831=CARTESIAN_POINT('Ctrl Pts',(0.00164126741877263,-0.0255264152695477,
-0.0102817414029005));
#34832=CARTESIAN_POINT('Ctrl Pts',(0.001766681045625,-0.0255150991464641,
-0.0104070010928943));
#34833=CARTESIAN_POINT('Ctrl Pts',(0.00210936107218999,-0.0254841789868592,
-0.0107492605025924));
#34834=CARTESIAN_POINT('Ctrl Pts',(0.00235032903843675,-0.0254532588272541,
-0.0111949342399714));
#34835=CARTESIAN_POINT('Ctrl Pts',(0.00244848861379047,-0.0254223386676491,
-0.0116709735898595));
#34836=CARTESIAN_POINT('Ctrl Pts',(0.0024826045117403,-0.0254115921968552,
-0.0118364236727716));
#34837=CARTESIAN_POINT('Ctrl Pts',(0.00249988091828759,-0.0254008457260614,
-0.0120053122063183));
#34838=CARTESIAN_POINT('Ctrl Pts',(0.00249999938422522,-0.0253900992552675,
-0.0121740986146384));
#34839=CARTESIAN_POINT('',(0.00249999952816097,-0.024390152306814,-0.0121770295369509));
#34840=CARTESIAN_POINT('Ctrl Pts',(0.00249999999999008,-0.0253899883594716,
-0.0121758462427209));
#34841=CARTESIAN_POINT('Ctrl Pts',(0.00250000136839726,-0.0253591394204884,
-0.0126615215734826));
#34842=CARTESIAN_POINT('Ctrl Pts',(0.00235419002331737,-0.0253282841355819,
-0.0131471701041643));
#34843=CARTESIAN_POINT('Ctrl Pts',(0.00208688788741109,-0.0252974109206306,
-0.0135524065711704));
#34844=CARTESIAN_POINT('Ctrl Pts',(0.00199397450730698,-0.0252866794884028,
-0.0136932654900987));
#34845=CARTESIAN_POINT('Ctrl Pts',(0.00188683073616151,-0.025275945889803,
-0.0138245546547794));
#34846=CARTESIAN_POINT('Ctrl Pts',(0.00176778032757569,-0.0252652096383225,
-0.013943606864814));
#34847=CARTESIAN_POINT('Ctrl Pts',(0.00143339557831302,-0.0252350540193544,
-0.0142779966739247));
#34848=CARTESIAN_POINT('Ctrl Pts',(0.000999612545386808,-0.0252048774713678,
-0.0145159046057349));
#34849=CARTESIAN_POINT('Ctrl Pts',(0.000536244085537721,-0.0251747123357439,
-0.014617664557055));
#34850=CARTESIAN_POINT('Ctrl Pts',(0.000360026360796584,-0.0251632406193308,
-0.0146563635809317));
#34851=CARTESIAN_POINT('Ctrl Pts',(0.000179805506686608,-0.0251517705534416,
-0.0146758523796725));
#34852=CARTESIAN_POINT('Ctrl Pts',(1.26097002276545E-8,-0.0251403039168796,
-0.0146758532865263));
#34853=CARTESIAN_POINT('Ctrl Pts',(-0.000488388216285484,-0.0251091552182267,
-0.0146758557499615));
#34854=CARTESIAN_POINT('Ctrl Pts',(-0.000977672425016896,-0.0250780318251737,
-0.0145284407289839));
#34855=CARTESIAN_POINT('Ctrl Pts',(-0.00138584435671831,-0.0250468029969821,
-0.0142565828266358));
#34856=CARTESIAN_POINT('Ctrl Pts',(-0.00152303930767185,-0.0250363063478513,
-0.0141652058144451));
#34857=CARTESIAN_POINT('Ctrl Pts',(-0.00165119095954436,-0.0250257977869763,
-0.0140601956449662));
#34858=CARTESIAN_POINT('Ctrl Pts',(-0.00176776249477623,-0.0250152723496241,
-0.0139436246977034));
#34859=CARTESIAN_POINT('Ctrl Pts',(-0.00199945562318164,-0.024994352392594,
-0.0137119327379227));
#34860=CARTESIAN_POINT('Ctrl Pts',(-0.00218550612955122,-0.0249733657666968,
-0.0134323885029887));
#34861=CARTESIAN_POINT('Ctrl Pts',(-0.00230969762490276,-0.0249527093738166,
-0.0131325647799136));
#34862=CARTESIAN_POINT('Ctrl Pts',(-0.00237179337257852,-0.0249423811773765,
-0.0129826529183761));
#34863=CARTESIAN_POINT('Ctrl Pts',(-0.00241920188088303,-0.0249321355391907,
-0.0128282808273792));
#34864=CARTESIAN_POINT('Ctrl Pts',(-0.00245196289350594,-0.024921416087868,
-0.0126635806375135));
#34865=CARTESIAN_POINT('Ctrl Pts',(-0.00248472390612885,-0.0249106966365453,
-0.0124988804476478));
#34866=CARTESIAN_POINT('Ctrl Pts',(-0.00250000000000001,-0.0248995033720857,
-0.01232309132871));
#34867=CARTESIAN_POINT('Ctrl Pts',(-0.0025,-0.024890114936556,-0.012175853286558));
#34868=CARTESIAN_POINT('Ctrl Pts',(-0.00249999999999999,-0.0248807265010263,
-0.0120286152444059));
#34869=CARTESIAN_POINT('Ctrl Pts',(-0.00248916168542769,-0.0248731428944265,
-0.0119098588003648));
#34870=CARTESIAN_POINT('Ctrl Pts',(-0.00246883231316729,-0.0248649169214783,
-0.0117823218272553));
#34871=CARTESIAN_POINT('Ctrl Pts',(-0.0024485029409069,-0.0248566909485302,
-0.0116547848541457));
#34872=CARTESIAN_POINT('Ctrl Pts',(-0.00241621500340535,-0.0248478226092338,
-0.0115190288997562));
#34873=CARTESIAN_POINT('Ctrl Pts',(-0.00237210836288918,-0.0248389128968786,
-0.0113864852388698));
#34874=CARTESIAN_POINT('Ctrl Pts',(-0.00228389508185683,-0.0248210934721682,
-0.011121397917097));
#34875=CARTESIAN_POINT('Ctrl Pts',(-0.00215053058275203,-0.0248031085552227,
-0.0108678864920868));
#34876=CARTESIAN_POINT('Ctrl Pts',(-0.00197052077585615,-0.024784486819113,
-0.0106373319601153));
#34877=CARTESIAN_POINT('Ctrl Pts',(-0.00179051096896026,-0.0247658650830033,
-0.0104067774281438));
#34878=CARTESIAN_POINT('Ctrl Pts',(-0.00156298563825604,-0.0247466065277293,
-0.0102001638565565));
#34879=CARTESIAN_POINT('Ctrl Pts',(-0.00129778925817226,-0.0247268367032592,
-0.0100390933465151));
#34880=CARTESIAN_POINT('Ctrl Pts',(-0.00103259287808847,-0.0247070668787891,
-0.0098780228364736));
#34881=CARTESIAN_POINT('Ctrl Pts',(-0.000730081343127169,-0.0246867857851227,
-0.00976244661799695));
#34882=CARTESIAN_POINT('Ctrl Pts',(-0.00040649663987185,-0.0246659625493172,
-0.00970912255910265));
#34883=CARTESIAN_POINT('Ctrl Pts',(3.52049012454766E-5,-0.0246375382905256,
-0.00963633383097276));
#34884=CARTESIAN_POINT('Ctrl Pts',(0.000514584471571425,-0.0246081038604287,
-0.00968312478566572));
#34885=CARTESIAN_POINT('Ctrl Pts',(0.000956243946241907,-0.0245776671113977,
-0.00986596205204603));
#34886=CARTESIAN_POINT('Ctrl Pts',(0.00116169224343761,-0.0245635087413882,
-0.00995101310879009));
#34887=CARTESIAN_POINT('Ctrl Pts',(0.00135861700196376,-0.0245491334831793,
-0.0100648674701259));
#34888=CARTESIAN_POINT('Ctrl Pts',(0.00153853044578671,-0.0245345421271688,
-0.010205339630836));
#34889=CARTESIAN_POINT('Ctrl Pts',(0.00189055074869411,-0.0245059925454727,
-0.0104801887555733));
#34890=CARTESIAN_POINT('Ctrl Pts',(0.00218016631731741,-0.0244766156723194,
-0.0108631077290133));
#34891=CARTESIAN_POINT('Ctrl Pts',(0.00234507266630632,-0.02444640953421,
-0.0113094618105249));
#34892=CARTESIAN_POINT('Ctrl Pts',(0.00244562968209433,-0.0244279903579601,
-0.011581640745398));
#34893=CARTESIAN_POINT('Ctrl Pts',(0.0025000009689668,-0.0244092628321647,
-0.01187638284372));
#34894=CARTESIAN_POINT('Ctrl Pts',(0.00249999999998691,-0.024390226509356,
-0.0121758613754508));
#34895=CARTESIAN_POINT('',(0.00249999997439014,-0.023390082751053,-0.0121756050547064));
#34896=CARTESIAN_POINT('Ctrl Pts',(0.00249999919082622,-0.0243900992552675,
-0.0121778647209288));
#34897=CARTESIAN_POINT('Ctrl Pts',(0.00249960845783168,-0.0243591775128979,
-0.0126635043144498));
#34898=CARTESIAN_POINT('Ctrl Pts',(0.00235342576395591,-0.0243282557705284,
-0.0131490022570672));
#34899=CARTESIAN_POINT('Ctrl Pts',(0.00208583353260368,-0.0242973340281588,
-0.0135540036681442));
#34900=CARTESIAN_POINT('Ctrl Pts',(0.00199284853085276,-0.0242865891038617,
-0.0136947366659888));
#34901=CARTESIAN_POINT('Ctrl Pts',(0.0018856518032898,-0.0242758441795646,
-0.0138258961121601));
#34902=CARTESIAN_POINT('Ctrl Pts',(0.00176656675632587,-0.0242650992552675,
-0.0139448196218636));
#34903=CARTESIAN_POINT('Ctrl Pts',(0.00143017696340042,-0.0242347471417868,
-0.0142807531065711));
#34904=CARTESIAN_POINT('Ctrl Pts',(0.00099359785863377,-0.0242043950283061,
-0.0145189828434659));
#34905=CARTESIAN_POINT('Ctrl Pts',(0.000527368666328687,-0.0241740429148254,
-0.0146195967857361));
#34906=CARTESIAN_POINT('Ctrl Pts',(0.000353569402019352,-0.0241627283616394,
-0.0146571032941968));
#34907=CARTESIAN_POINT('Ctrl Pts',(0.000175914055471926,-0.0241514138084535,
-0.0146759509197155));
#34908=CARTESIAN_POINT('Ctrl Pts',(-1.38208273950699E-6,-0.0241400992552675,
-0.0146758529045275));
#34909=CARTESIAN_POINT('Ctrl Pts',(-0.000478750851133147,-0.0241096348899757,
-0.0146755889992331));
#34910=CARTESIAN_POINT('Ctrl Pts',(-0.000957571928518442,-0.0240791705246838,
-0.0145342776525842));
#34911=CARTESIAN_POINT('Ctrl Pts',(-0.00135929122746163,-0.024048706159392,
-0.0142740256719797));
#34912=CARTESIAN_POINT('Ctrl Pts',(-0.00150701072241057,-0.0240375038580171,
-0.0141783262837863));
#34913=CARTESIAN_POINT('Ctrl Pts',(-0.00164444690479554,-0.0240263015566424,
-0.0140670459612177));
#34914=CARTESIAN_POINT('Ctrl Pts',(-0.00176852156248608,-0.0240150992552675,
-0.0139428653077458));
#34915=CARTESIAN_POINT('Ctrl Pts',(-0.00210587590077154,-0.0239846406182023,
-0.0136052227709083));
#34916=CARTESIAN_POINT('Ctrl Pts',(-0.0023445600348803,-0.0239541819811371,
-0.0131668393892154));
#34917=CARTESIAN_POINT('Ctrl Pts',(-0.00244467776727557,-0.023923723344072,
-0.0126988739498101));
#34918=CARTESIAN_POINT('Ctrl Pts',(-0.00248151863136018,-0.0239125153144705,
-0.0125266741732374));
#34919=CARTESIAN_POINT('Ctrl Pts',(-0.00250005276538172,-0.023901307284869,
-0.0123507233831673));
#34920=CARTESIAN_POINT('Ctrl Pts',(-0.0024999998866792,-0.0238900992552675,
-0.0121751005555373));
#34921=CARTESIAN_POINT('Ctrl Pts',(-0.00249985618495232,-0.0238596406182022,
-0.0116978327254759));
#34922=CARTESIAN_POINT('Ctrl Pts',(-0.00235872289837664,-0.0238291819811368,
-0.0112190599612614));
#34923=CARTESIAN_POINT('Ctrl Pts',(-0.00209866256915363,-0.0237987233440715,
-0.0108173189951861));
#34924=CARTESIAN_POINT('Ctrl Pts',(-0.00200296676169467,-0.0237875153144702,
-0.010669488196645));
#34925=CARTESIAN_POINT('Ctrl Pts',(-0.00189167007198695,-0.0237763072848689,
-0.0105319459848342));
#34926=CARTESIAN_POINT('Ctrl Pts',(-0.00176745717406797,-0.0237650992552675,
-0.0104077766089687));
#34927=CARTESIAN_POINT('Ctrl Pts',(-0.00142983609072378,-0.0237346348899757,
-0.0100702738222191));
#34928=CARTESIAN_POINT('Ctrl Pts',(-0.000991418463670934,-0.0237041705246839,
-0.00983145743438289));
#34929=CARTESIAN_POINT('Ctrl Pts',(-0.000523378534922975,-0.023673706159392,
-0.00973125211066419));
#34930=CARTESIAN_POINT('Ctrl Pts',(-0.000351271737782169,-0.0236625038580172,
-0.00969440479003534));
#34931=CARTESIAN_POINT('Ctrl Pts',(-0.000175413828559905,-0.0236513015566424,
-0.00967584462654266));
#34932=CARTESIAN_POINT('Ctrl Pts',(1.23379254317394E-7,-0.0236400992552675,
-0.00967585328960259));
#34933=CARTESIAN_POINT('Ctrl Pts',(0.000475733262739959,-0.0236097471417868,
-0.00967587676175972));
#34934=CARTESIAN_POINT('Ctrl Pts',(0.000953014801081544,-0.0235793950283061,
-0.00981594521882193));
#34935=CARTESIAN_POINT('Ctrl Pts',(0.0013538998578098,-0.0235490429148253,
-0.0100741979449232));
#34936=CARTESIAN_POINT('Ctrl Pts',(0.00150334036707393,-0.0235377283616394,
-0.0101704684799798));
#34937=CARTESIAN_POINT('Ctrl Pts',(0.00164230892020507,-0.0235264138084535,
-0.0102826474887713));
#34938=CARTESIAN_POINT('Ctrl Pts',(0.0017676316806438,-0.0235150992552675,
-0.0104079510716196));
#34939=CARTESIAN_POINT('Ctrl Pts',(0.00211012846753573,-0.0234841775128981,
-0.0107503954477357));
#34940=CARTESIAN_POINT('Ctrl Pts',(0.00235085694096267,-0.0234532557705288,
-0.0111961996941204));
#34941=CARTESIAN_POINT('Ctrl Pts',(0.00244876022617186,-0.0234223340281594,
-0.0116722926102551));
#34942=CARTESIAN_POINT('Ctrl Pts',(0.00248278041091645,-0.0234115891038621,
-0.0118377290297571));
#34943=CARTESIAN_POINT('Ctrl Pts',(0.00249996579487876,-0.0234008441795648,
-0.0120065934906643));
#34944=CARTESIAN_POINT('Ctrl Pts',(0.00249999994879836,-0.0233900992552675,
-0.0121753473140382));
#34945=CARTESIAN_POINT('',(0.00249999978282922,-0.0223900527209141,-0.0121751135025362));
#34946=CARTESIAN_POINT('Ctrl Pts',(0.00249999999998192,-0.0233900662468386,
-0.0121758627953746));
#34947=CARTESIAN_POINT('Ctrl Pts',(0.00249999815284274,-0.0233591476370275,
-0.0126615013552356));
#34948=CARTESIAN_POINT('Ctrl Pts',(0.00235420495401003,-0.0233282290272166,
-0.01314711521106));
#34949=CARTESIAN_POINT('Ctrl Pts',(0.00208693825047046,-0.0232973104174055,
-0.0135523302165222));
#34950=CARTESIAN_POINT('Ctrl Pts',(0.00199404176653275,-0.0232865637359011,
-0.0136931747315616));
#34951=CARTESIAN_POINT('Ctrl Pts',(0.00188691839382461,-0.0232758170543966,
-0.0138244520404621));
#34952=CARTESIAN_POINT('Ctrl Pts',(0.00176789131965712,-0.0232650703728922,
-0.0139434958640836));
#34953=CARTESIAN_POINT('Ctrl Pts',(0.0014317551106563,-0.0232347214056046,
-0.0142796793740706));
#34954=CARTESIAN_POINT('Ctrl Pts',(0.000995357070768357,-0.0232043724383171,
-0.0145182356543401));
#34955=CARTESIAN_POINT('Ctrl Pts',(0.000529205667740109,-0.0231740234710294,
-0.0146191996314777));
#34956=CARTESIAN_POINT('Ctrl Pts',(0.0003553901875384,-0.0231627071470016,
-0.0146568464175974));
#34957=CARTESIAN_POINT('Ctrl Pts',(0.000177702613060415,-0.0231513908229737,
-0.0146758276322675));
#34958=CARTESIAN_POINT('Ctrl Pts',(3.61283311594722E-7,-0.0231400744989458,
-0.014675853260453));
#34959=CARTESIAN_POINT('Ctrl Pts',(-0.000477005090471533,-0.0231096132828639,
-0.0146759222462554));
#34960=CARTESIAN_POINT('Ctrl Pts',(-0.00095592265976367,-0.0230791520667819,
-0.014534946223913));
#34961=CARTESIAN_POINT('Ctrl Pts',(-0.00135782237193734,-0.0230486908507,
-0.0142749765335987));
#34962=CARTESIAN_POINT('Ctrl Pts',(-0.00150564689080733,-0.0230374867754665,
-0.0141793559266975));
#34963=CARTESIAN_POINT('Ctrl Pts',(-0.00164319368247117,-0.023026282700233,
-0.0140681391251308));
#34964=CARTESIAN_POINT('Ctrl Pts',(-0.00176738035000952,-0.0230150786249995,
-0.0139440067579514));
#34965=CARTESIAN_POINT('Ctrl Pts',(-0.00210495091791582,-0.0229846231331628,
-0.0136065837920654));
#34966=CARTESIAN_POINT('Ctrl Pts',(-0.0023439176592855,-0.0229541676413262,
-0.0131683568875582));
#34967=CARTESIAN_POINT('Ctrl Pts',(-0.00244433827125326,-0.0229237121494896,
-0.0127004582957666));
#34968=CARTESIAN_POINT('Ctrl Pts',(-0.00248130023954904,-0.0229125023500108,
-0.0125282381451764));
#34969=CARTESIAN_POINT('Ctrl Pts',(-0.002499948451974,-0.0229012925505319,
-0.0123522531780084));
#34970=CARTESIAN_POINT('Ctrl Pts',(-0.00249999989281311,-0.0228900827510531,
-0.0121765853619898));
#34971=CARTESIAN_POINT('Ctrl Pts',(-0.00250013965053656,-0.0228596272592165,
-0.0116993199348243));
#34972=CARTESIAN_POINT('Ctrl Pts',(-0.00235929209470182,-0.02282917176738,
-0.0112204653179175));
#34973=CARTESIAN_POINT('Ctrl Pts',(-0.00209947244932243,-0.0227987162755435,
-0.0108185709155917));
#34974=CARTESIAN_POINT('Ctrl Pts',(-0.00200384023490871,-0.0227875064760646,
-0.0106706450280063));
#34975=CARTESIAN_POINT('Ctrl Pts',(-0.00189259294181167,-0.0227762966765856,
-0.0105330037373359));
#34976=CARTESIAN_POINT('Ctrl Pts',(-0.0017684155842339,-0.0227650868771067,
-0.0104087352029432));
#34977=CARTESIAN_POINT('Ctrl Pts',(-0.00143097927872439,-0.0227346256610247,
-0.0100710511359404));
#34978=CARTESIAN_POINT('Ctrl Pts',(-0.000992693544891953,-0.0227041644449427,
-0.00983199746057321));
#34979=CARTESIAN_POINT('Ctrl Pts',(-0.000524710188623356,-0.0226737032288607,
-0.00973153759132664));
#34980=CARTESIAN_POINT('Ctrl Pts',(-0.000352579150994395,-0.0226624991536272,
-0.0096945870004523));
#34981=CARTESIAN_POINT('Ctrl Pts',(-0.000176685099276302,-0.0226512950783938,
-0.00967593098740631));
#34982=CARTESIAN_POINT('Ctrl Pts',(-1.10286753579808E-6,-0.0226400910031603,
-0.00967585352982147));
#34983=CARTESIAN_POINT('Ctrl Pts',(0.000474504382178306,-0.0226097420358727,
-0.00967564371708286));
#34984=CARTESIAN_POINT('Ctrl Pts',(0.000951852528106953,-0.0225793930685852,
-0.00981547660079706));
#34985=CARTESIAN_POINT('Ctrl Pts',(0.00135286317164378,-0.0225490441012976,
-0.0100735304667205));
#34986=CARTESIAN_POINT('Ctrl Pts',(0.00150238939235155,-0.0225377277772697,
-0.0101697519010701));
#34987=CARTESIAN_POINT('Ctrl Pts',(0.0016414461183173,-0.0225264114532418,
-0.0102818951503619));
#34988=CARTESIAN_POINT('Ctrl Pts',(0.00176685577834738,-0.0225150951292139,
-0.0104071756283851));
#34989=CARTESIAN_POINT('Ctrl Pts',(0.00210950170607601,-0.0224841765194028,
-0.0107494686033299));
#34990=CARTESIAN_POINT('Ctrl Pts',(0.00235042559911038,-0.0224532579095917,
-0.0111951657732823));
#34991=CARTESIAN_POINT('Ctrl Pts',(0.00244853827886408,-0.0224223392997806,
-0.0116712145078883));
#34992=CARTESIAN_POINT('Ctrl Pts',(0.0024826402558706,-0.0224115926182762,
-0.0118366793901265));
#34993=CARTESIAN_POINT('Ctrl Pts',(0.00249990006528172,-0.0224008459367719,
-0.0120055815453249));
#34994=CARTESIAN_POINT('Ctrl Pts',(0.00249999956566543,-0.0223900992552675,
-0.0121743796269425));
#34995=CARTESIAN_POINT('',(0.00249999946670881,-0.0213901564165093,-0.012177099742631));
#34996=CARTESIAN_POINT('Ctrl Pts',(0.00249999999999302,-0.0223900061865608,
-0.0121758473781298));
#34997=CARTESIAN_POINT('Ctrl Pts',(0.00250000114022626,-0.0223593773858453,
-0.0126583078509963));
#34998=CARTESIAN_POINT('Ctrl Pts',(0.00235604930438737,-0.0223287344743284,
-0.0131410200720147));
#34999=CARTESIAN_POINT('Ctrl Pts',(0.00209205887758274,-0.0222980771500896,
-0.0135445350073125));
#35000=CARTESIAN_POINT('Ctrl Pts',(0.00199792613435286,-0.0222871454732647,
-0.0136884188907304));
#35001=CARTESIAN_POINT('Ctrl Pts',(0.00188900128248741,-0.0222762119639099,
-0.0138223841604978));
#35002=CARTESIAN_POINT('Ctrl Pts',(0.0017677797086252,-0.0222652766083368,
-0.0139436074837736));
#35003=CARTESIAN_POINT('Ctrl Pts',(0.00143008399010385,-0.0222348131962569,
-0.0142813080757631));
#35004=CARTESIAN_POINT('Ctrl Pts',(0.000991179767819557,-0.0222043354565482,
-0.0145205707095847));
#35005=CARTESIAN_POINT('Ctrl Pts',(0.000522028801479781,-0.0221738442769973,
-0.014620743044896));
#35006=CARTESIAN_POINT('Ctrl Pts',(0.000350468005067636,-0.0221626941538544,
-0.0146573744212706));
#35007=CARTESIAN_POINT('Ctrl Pts',(0.000175121182212468,-0.0221515422334758,
-0.0146758524441749));
#35008=CARTESIAN_POINT('Ctrl Pts',(1.20261312456349E-8,-0.0221403885592749,
-0.0146758532865292));
#35009=CARTESIAN_POINT('Ctrl Pts',(-0.000326969715656887,-0.0221195612770291,
-0.0146758548594593));
#35010=CARTESIAN_POINT('Ctrl Pts',(-0.000654265414087993,-0.0220987278795242,
-0.0146108269010241));
#35011=CARTESIAN_POINT('Ctrl Pts',(-0.000956700247905833,-0.0220778855401309,
-0.0144855555694632));
#35012=CARTESIAN_POINT('Ctrl Pts',(-0.00125913508172367,-0.0220570432007376,
-0.0143602842379022));
#35013=CARTESIAN_POINT('Ctrl Pts',(-0.00153644332769053,-0.0220361919194559,
-0.0141749427520477));
#35014=CARTESIAN_POINT('Ctrl Pts',(-0.00176776270110393,-0.0220153431912449,
-0.0139436244913767));
#35015=CARTESIAN_POINT('Ctrl Pts',(-0.00188342238781062,-0.0220049188271394,
-0.0138279653610412));
#35016=CARTESIAN_POINT('Ctrl Pts',(-0.00198770652448018,-0.0219944951013015,
-0.0137009208315779));
#35017=CARTESIAN_POINT('Ctrl Pts',(-0.00207867152525912,-0.0219840572681485,
-0.0135647826188414));
#35018=CARTESIAN_POINT('Ctrl Pts',(-0.00216963652603806,-0.0219736194349956,
-0.0134286444061049));
#35019=CARTESIAN_POINT('Ctrl Pts',(-0.00224723455883184,-0.0219631674945277,
-0.013283363448231));
#35020=CARTESIAN_POINT('Ctrl Pts',(-0.00230969768073528,-0.0219527615126167,
-0.0131325646451225));
#35021=CARTESIAN_POINT('Ctrl Pts',(-0.00237216080263872,-0.0219423555307058,
-0.0129817658420139));
#35022=CARTESIAN_POINT('Ctrl Pts',(-0.00241973422772398,-0.0219319955073519,
-0.0128256045726092));
#35023=CARTESIAN_POINT('Ctrl Pts',(-0.0024519629077376,-0.0219214559246494,
-0.0126635805659663));
#35024=CARTESIAN_POINT('Ctrl Pts',(-0.00246807724774441,-0.0219161861332981,
-0.0125825685626449));
#35025=CARTESIAN_POINT('Ctrl Pts',(-0.00248016729986118,-0.0219108714521097,
-0.0125000349508198));
#35026=CARTESIAN_POINT('Ctrl Pts',(-0.00248796174300818,-0.0219057994435024,
-0.0124208968853884));
#35027=CARTESIAN_POINT('Ctrl Pts',(-0.00249185896458168,-0.0219032634391987,
-0.0123813278526727));
#35028=CARTESIAN_POINT('Ctrl Pts',(-0.00249482184802687,-0.0219007881030403,
-0.0123426284113902));
#35029=CARTESIAN_POINT('Ctrl Pts',(-0.00249698862207265,-0.021897970281138,
-0.0122985228477366));
#35030=CARTESIAN_POINT('Ctrl Pts',(-0.00249915539611843,-0.0218951524592358,
-0.012254417284083));
#35031=CARTESIAN_POINT('Ctrl Pts',(-0.0025,-0.0218919921515896,-0.0122048746012686));
#35032=CARTESIAN_POINT('Ctrl Pts',(-0.0025,-0.0218901405042465,-0.012175853286558));
#35033=CARTESIAN_POINT('Ctrl Pts',(-0.0025,-0.0218882888569033,-0.0121468319718473));
#35034=CARTESIAN_POINT('Ctrl Pts',(-0.00249975948868643,-0.0218877458698631,
-0.0121383237374989));
#35035=CARTESIAN_POINT('Ctrl Pts',(-0.00249946167551239,-0.0218868304812657,
-0.0121239752310355));
#35036=CARTESIAN_POINT('Ctrl Pts',(-0.00249916386233835,-0.0218859150926683,
-0.0121096267245721));
#35037=CARTESIAN_POINT('Ctrl Pts',(-0.00249858311755661,-0.0218846273025136,
-0.0120894460511038));
#35038=CARTESIAN_POINT('Ctrl Pts',(-0.0024977526130494,-0.0218833775691218,
-0.0120698727034076));
#35039=CARTESIAN_POINT('Ctrl Pts',(-0.00249609160403497,-0.0218808781023383,
-0.0120307260080153));
#35040=CARTESIAN_POINT('Ctrl Pts',(-0.0024936817236808,-0.0218785308626062,
-0.0119939903198025));
#35041=CARTESIAN_POINT('Ctrl Pts',(-0.00249023640476994,-0.0218760430773448,
-0.0119551212128613));
#35042=CARTESIAN_POINT('Ctrl Pts',(-0.00248334576694822,-0.0218710675068219,
-0.011877382998979));
#35043=CARTESIAN_POINT('Ctrl Pts',(-0.00247194153334508,-0.0218655297541816,
-0.0117911618818107));
#35044=CARTESIAN_POINT('Ctrl Pts',(-0.00245443835988697,-0.0218596594238335,
-0.0117007403131346));
#35045=CARTESIAN_POINT('Ctrl Pts',(-0.00243693518642886,-0.0218537890934854,
-0.0116103187444584));
#35046=CARTESIAN_POINT('Ctrl Pts',(-0.00241347394517101,-0.0218475861854294,
-0.0115156557012848));
#35047=CARTESIAN_POINT('Ctrl Pts',(-0.00238205060024122,-0.0218409895437126,
-0.0114170154001222));
#35048=CARTESIAN_POINT('Ctrl Pts',(-0.00235062725531143,-0.0218343929019958,
-0.0113183750989597));
#35049=CARTESIAN_POINT('Ctrl Pts',(-0.00231120270368248,-0.0218274025266182,
-0.0112157783033761));
#35050=CARTESIAN_POINT('Ctrl Pts',(-0.00226189465481612,-0.0218200334369823,
-0.0111110375416922));
#35051=CARTESIAN_POINT('Ctrl Pts',(-0.0021632785570834,-0.0218052952577104,
-0.0109015560183245));
#35052=CARTESIAN_POINT('Ctrl Pts',(-0.00202509411853232,-0.0217890422214056,
-0.0106835381773548));
#35053=CARTESIAN_POINT('Ctrl Pts',(-0.001835460791482,-0.0217712625436928,
-0.0104784777585937));
#35054=CARTESIAN_POINT('Ctrl Pts',(-0.00164582746443168,-0.02175348286598,
-0.0102734173398327));
#35055=CARTESIAN_POINT('Ctrl Pts',(-0.00140431280704041,-0.0217341765468593,
-0.0100818042152198));
#35056=CARTESIAN_POINT('Ctrl Pts',(-0.00111110002761456,-0.0217133467439652,
-0.00993633174644402));
#35057=CARTESIAN_POINT('Ctrl Pts',(-0.00081788724818871,-0.021692516941071,
-0.00979085927766821));
#35058=CARTESIAN_POINT('Ctrl Pts',(-0.000472595108618116,-0.0216701636544036,
-0.0096924156088888));
#35059=CARTESIAN_POINT('Ctrl Pts',(-9.76363564151474E-5,-0.0216462860377993,
-0.00967776058573494));
#35060=CARTESIAN_POINT('Ctrl Pts',(0.000277322395787821,-0.0216224084211949,
-0.00966310556258107));
#35061=CARTESIAN_POINT('Ctrl Pts',(0.000681901047087343,-0.0215970064746537,
-0.00973369490722545));
#35062=CARTESIAN_POINT('Ctrl Pts',(0.00106482420138709,-0.0215700804251951,
-0.00991396261277646));
#35063=CARTESIAN_POINT('Ctrl Pts',(0.00144774735568684,-0.0215431543757365,
-0.0100942303183275));
#35064=CARTESIAN_POINT('Ctrl Pts',(0.00180788869735316,-0.0215147042233605,
-0.0103860811844988));
#35065=CARTESIAN_POINT('Ctrl Pts',(0.00207151346256511,-0.0214847299061527,
-0.010776270500721));
#35066=CARTESIAN_POINT('Ctrl Pts',(0.00231596365811457,-0.0214569357507098,
-0.0111380796599445));
#35067=CARTESIAN_POINT('Ctrl Pts',(0.00247586744117682,-0.0214278310853771,
-0.0115853104295833));
#35068=CARTESIAN_POINT('Ctrl Pts',(0.00249745187057231,-0.0213974159266089,
-0.0120630075769592));
#35069=CARTESIAN_POINT('Ctrl Pts',(0.00249914479383464,-0.0213950303861407,
-0.0121004746138832));
#35070=CARTESIAN_POINT('Ctrl Pts',(0.00250000013050565,-0.0213926367839425,
-0.0121381054938293));
#35071=CARTESIAN_POINT('Ctrl Pts',(0.00249999999998506,-0.0213902351200221,
-0.0121758619288322));
#35072=CARTESIAN_POINT('',(0.00249990205332692,-0.0203902475809712,-0.012175258225647));
#35073=CARTESIAN_POINT('Ctrl Pts',(0.00249999907939785,-0.0213900992552675,
-0.0121779987491857));
#35074=CARTESIAN_POINT('Ctrl Pts',(0.00249958231006304,-0.0213591763542908,
-0.0126636389742638));
#35075=CARTESIAN_POINT('Ctrl Pts',(0.00235337321701218,-0.021328253453314,
-0.0131491296217983));
#35076=CARTESIAN_POINT('Ctrl Pts',(0.00208575865386121,-0.0212973305523372,
-0.0135541169905869));
#35077=CARTESIAN_POINT('Ctrl Pts',(0.00199277940318017,-0.0212865867866473,
-0.0136948246622542));
#35078=CARTESIAN_POINT('Ctrl Pts',(0.00188559305150799,-0.0212758430209575,
-0.0138259607867651));
#35079=CARTESIAN_POINT('Ctrl Pts',(0.00176652209780973,-0.0212650992552675,
-0.0139448642186752));
#35080=CARTESIAN_POINT('Ctrl Pts',(0.00143012280556268,-0.0212347459653853,
-0.0142807902283188));
#35081=CARTESIAN_POINT('Ctrl Pts',(0.000993536318349333,-0.0212043926755031,
-0.0145190091690837));
#35082=CARTESIAN_POINT('Ctrl Pts',(0.000527303328876991,-0.0211740393856209,
-0.0146196108848798));
#35083=CARTESIAN_POINT('Ctrl Pts',(0.000353527454837905,-0.0211627260088364,
-0.0146571074831195));
#35084=CARTESIAN_POINT('Ctrl Pts',(0.000175897082413975,-0.021151412632052,
-0.0146759503570788));
#35085=CARTESIAN_POINT('Ctrl Pts',(-1.37428056251401E-6,-0.0211400992552675,
-0.0146758529088287));
#35086=CARTESIAN_POINT('Ctrl Pts',(-0.000478744400520623,-0.0211096337139525,
-0.0146755904925982));
#35087=CARTESIAN_POINT('Ctrl Pts',(-0.000957566979565421,-0.0210791681726375,
-0.0145342798794274));
#35088=CARTESIAN_POINT('Ctrl Pts',(-0.00135928762466615,-0.0210487026313225,
-0.0142740280060296));
#35089=CARTESIAN_POINT('Ctrl Pts',(-0.00150698640525244,-0.0210375015059708,
-0.0141783423975977));
#35090=CARTESIAN_POINT('Ctrl Pts',(-0.00164440482203652,-0.0210263003806192,
-0.0140670802591278));
#35091=CARTESIAN_POINT('Ctrl Pts',(-0.00176846592375923,-0.0210150992552675,
-0.0139429209922509));
#35092=CARTESIAN_POINT('Ctrl Pts',(-0.00210583182168066,-0.0209846394442589,
-0.0136052881486477));
#35093=CARTESIAN_POINT('Ctrl Pts',(-0.00234452996584051,-0.0209541796332503,
-0.0131669110301521));
#35094=CARTESIAN_POINT('Ctrl Pts',(-0.00244466201221942,-0.0209237198222416,
-0.012698947585907));
#35095=CARTESIAN_POINT('Ctrl Pts',(-0.00248150286425866,-0.0209125129665836,
-0.012526773215836));
#35096=CARTESIAN_POINT('Ctrl Pts',(-0.00250004228843935,-0.0209013061109256,
-0.0123508483409523));
#35097=CARTESIAN_POINT('Ctrl Pts',(-0.00249999992725447,-0.0208900992552675,
-0.0121752501881915));
#35098=CARTESIAN_POINT('Ctrl Pts',(-0.00249988479115165,-0.0208596394442589,
-0.0116979810317242));
#35099=CARTESIAN_POINT('Ctrl Pts',(-0.00235877941875351,-0.0208291796332502,
-0.0112191987874848));
#35100=CARTESIAN_POINT('Ctrl Pts',(-0.00209874201892454,-0.0207987198222416,
-0.0108174417369898));
#35101=CARTESIAN_POINT('Ctrl Pts',(-0.00200306835881087,-0.0207875129665835,
-0.0106696262015222));
#35102=CARTESIAN_POINT('Ctrl Pts',(-0.00189179763511228,-0.0207763061109256,
-0.0105320954221778));
#35103=CARTESIAN_POINT('Ctrl Pts',(-0.00176761314542966,-0.0207650992552675,
-0.0104079325394361));
#35104=CARTESIAN_POINT('Ctrl Pts',(-0.001430020887926,-0.0207346337139525,
-0.0100703990198312));
#35105=CARTESIAN_POINT('Ctrl Pts',(-0.000991623047142472,-0.0207041681726375,
-0.00983154374161374));
#35106=CARTESIAN_POINT('Ctrl Pts',(-0.000523590769440504,-0.0206737026313225,
-0.00973129755879146));
#35107=CARTESIAN_POINT('Ctrl Pts',(-0.000351511496107748,-0.0206625015059708,
-0.00969444050615581));
#35108=CARTESIAN_POINT('Ctrl Pts',(-0.00017568058482422,-0.0206513003806192,
-0.00967586509253789));
#35109=CARTESIAN_POINT('Ctrl Pts',(-1.68083886645815E-7,-0.0206400992552675,
-0.00967585329220854));
#35110=CARTESIAN_POINT('Ctrl Pts',(0.000475443218696623,-0.0206097459653853,
-0.00967582131516996));
#35111=CARTESIAN_POINT('Ctrl Pts',(0.000952742201519874,-0.0205793926755031,
-0.0098158349233419));
#35112=CARTESIAN_POINT('Ctrl Pts',(0.00135365793268781,-0.0205490393856208,
-0.0100740421149084));
#35113=CARTESIAN_POINT('Ctrl Pts',(0.00150308854607822,-0.0205377260088364,
-0.0101702819379386));
#35114=CARTESIAN_POINT('Ctrl Pts',(0.00164205199002488,-0.020526412632052,
-0.0102824269558209));
#35115=CARTESIAN_POINT('Ctrl Pts',(0.00176737540225734,-0.0205150992552675,
-0.0104076948695898));
#35116=CARTESIAN_POINT('Ctrl Pts',(0.00210992241897826,-0.0204841763542906,
-0.0107500901921239));
#35117=CARTESIAN_POINT('Ctrl Pts',(0.0023507156029587,-0.0204532534533137,
-0.0111958603106268));
#35118=CARTESIAN_POINT('Ctrl Pts',(0.00244868762262492,-0.0204223305523368,
-0.0116719396761014));
#35119=CARTESIAN_POINT('Ctrl Pts',(0.00248272674541716,-0.020411586786647,
-0.0118373473510217));
#35120=CARTESIAN_POINT('Ctrl Pts',(0.00249993643078121,-0.0204008430209573,
-0.0120061844971346));
#35121=CARTESIAN_POINT('Ctrl Pts',(0.00249999982355582,-0.0203900992552675,
-0.0121749140204342));
#35122=CARTESIAN_POINT('',(0.00249999986986764,-0.0193900632541159,-0.0121752806287112));
#35123=CARTESIAN_POINT('Ctrl Pts',(0.00249999999995715,-0.0203900382015828,
-0.0121758679244561));
#35124=CARTESIAN_POINT('Ctrl Pts',(0.00249999715646827,-0.0203591211281684,
-0.012661506106886));
#35125=CARTESIAN_POINT('Ctrl Pts',(0.00235420317554791,-0.0203282040547541,
-0.0131471193498656));
#35126=CARTESIAN_POINT('Ctrl Pts',(0.00208693599846101,-0.0202972869813398,
-0.0135523336308884));
#35127=CARTESIAN_POINT('Ctrl Pts',(0.00199403155362639,-0.020286539931991,
-0.0136931897144067));
#35128=CARTESIAN_POINT('Ctrl Pts',(0.00188689786182557,-0.0202757928826422,
-0.013824476965648));
#35129=CARTESIAN_POINT('Ctrl Pts',(0.00176785872255326,-0.0202650458332934,
-0.0139435284651733));
#35130=CARTESIAN_POINT('Ctrl Pts',(0.00143171690229952,-0.0202346983967062,
-0.0142797051882159));
#35131=CARTESIAN_POINT('Ctrl Pts',(0.000995315253905716,-0.0202043509601189,
-0.0145182532900219));
#35132=CARTESIAN_POINT('Ctrl Pts',(0.000529162715761184,-0.0201740035235317,
-0.0146192089340741));
#35133=CARTESIAN_POINT('Ctrl Pts',(0.000355332482386485,-0.0201626868373558,
-0.0146568557164684));
#35134=CARTESIAN_POINT('Ctrl Pts',(0.000177629853437843,-0.0201513701511799,
-0.0146758338185694));
#35135=CARTESIAN_POINT('Ctrl Pts',(2.74208224093162E-7,-0.020140053465004,
-0.0146758532715201));
#35136=CARTESIAN_POINT('Ctrl Pts',(-0.000477091387164691,-0.0201095937825525,
-0.0146759056305492));
#35137=CARTESIAN_POINT('Ctrl Pts',(-0.000956003432813248,-0.020079134100101,
-0.0145349133668213));
#35138=CARTESIAN_POINT('Ctrl Pts',(-0.0013578937810368,-0.0200486744176495,
-0.0142749303407468));
#35139=CARTESIAN_POINT('Ctrl Pts',(-0.00150572711533615,-0.0200374699773378,
-0.0141792968980038));
#35140=CARTESIAN_POINT('Ctrl Pts',(-0.00164328050466185,-0.0200262655370262,
-0.0140680650532317));
#35141=CARTESIAN_POINT('Ctrl Pts',(-0.00176747091116223,-0.0200150610967145,
-0.0139439162317598));
#35142=CARTESIAN_POINT('Ctrl Pts',(-0.00210502365928357,-0.019984607137146,
-0.0136064765128253));
#35143=CARTESIAN_POINT('Ctrl Pts',(-0.00234396783479502,-0.0199541531775775,
-0.0131682380928252));
#35144=CARTESIAN_POINT('Ctrl Pts',(-0.00244436472397797,-0.019923699218009,
-0.0127003350271098));
#35145=CARTESIAN_POINT('Ctrl Pts',(-0.00248132101892018,-0.0199124890548144,
-0.0125280989763549));
#35146=CARTESIAN_POINT('Ctrl Pts',(-0.00249996036917035,-0.0199012788916198,
-0.0123520984181568));
#35147=CARTESIAN_POINT('Ctrl Pts',(-0.00249999993659396,-0.0198900687284252,
-0.0121764163409007));
#35148=CARTESIAN_POINT('Ctrl Pts',(-0.00250010742697549,-0.0198596147688566,
-0.0116991516673366));
#35149=CARTESIAN_POINT('Ctrl Pts',(-0.00235922792536984,-0.0198291608092881,
-0.0112203071714482));
#35150=CARTESIAN_POINT('Ctrl Pts',(-0.00209938175411062,-0.0197987068497195,
-0.0108184306366412));
#35151=CARTESIAN_POINT('Ctrl Pts',(-0.00200373186074464,-0.0197874966865249,
-0.0106704990834677));
#35152=CARTESIAN_POINT('Ctrl Pts',(-0.00189246502018833,-0.0197762865233303,
-0.0105328548560365));
#35153=CARTESIAN_POINT('Ctrl Pts',(-0.0017682671442481,-0.0197650763601357,
-0.0104085866664431));
#35154=CARTESIAN_POINT('Ctrl Pts',(-0.00143080302382207,-0.0197346166776842,
-0.0100709314933526));
#35155=CARTESIAN_POINT('Ctrl Pts',(-0.000992497953249737,-0.0197041569952327,
-0.00983191475799308));
#35156=CARTESIAN_POINT('Ctrl Pts',(-0.000524506848390027,-0.0196736973127811,
-0.00973149395004639));
#35157=CARTESIAN_POINT('Ctrl Pts',(-0.000352358684694864,-0.0196624928724695,
-0.00969455466315548));
#35158=CARTESIAN_POINT('Ctrl Pts',(-0.000176448413992738,-0.0196512884321579,
-0.00967591326800827));
#35159=CARTESIAN_POINT('Ctrl Pts',(-8.51900453529701E-7,-0.0196400839918463,
-0.00967585343170498));
#35160=CARTESIAN_POINT('Ctrl Pts',(0.000474754547648577,-0.019609736555259,
-0.00967569136395604));
#35161=CARTESIAN_POINT('Ctrl Pts',(0.000952088007784488,-0.0195793891186717,
-0.00981557170663914));
#35162=CARTESIAN_POINT('Ctrl Pts',(0.00135307241530568,-0.0195490416820845,
-0.0100736651315779));
#35163=CARTESIAN_POINT('Ctrl Pts',(0.00150260117989429,-0.0195377249959086,
-0.0101699092504406));
#35164=CARTESIAN_POINT('Ctrl Pts',(0.00164165715754688,-0.0195264083097328,
-0.010282076734405));
#35165=CARTESIAN_POINT('Ctrl Pts',(0.00176706230547633,-0.0195150916235569,
-0.0104073819668685));
#35166=CARTESIAN_POINT('Ctrl Pts',(0.00210966791500204,-0.0194841745501424,
-0.010749714608341));
#35167=CARTESIAN_POINT('Ctrl Pts',(0.00235053970574287,-0.019453257476728,
-0.0111954394640646));
#35168=CARTESIAN_POINT('Ctrl Pts',(0.00244859695247532,-0.0194223404033135,
-0.011671499279606));
#35169=CARTESIAN_POINT('Ctrl Pts',(0.00248268252246114,-0.0194115933539649,
-0.0118369819002261));
#35170=CARTESIAN_POINT('Ctrl Pts',(0.00249992271098996,-0.0194008463046161,
-0.0120059004115422));
#35171=CARTESIAN_POINT('Ctrl Pts',(0.00249999973973945,-0.0193900992552675,
-0.012174712540005));
#35172=CARTESIAN_POINT('',(0.00249999952946043,-0.0183901705276876,-0.012176929269498));
#35173=CARTESIAN_POINT('Ctrl Pts',(0.00249999999999582,-0.0193900272529644,
-0.0121758487174173));
#35174=CARTESIAN_POINT('Ctrl Pts',(0.00250000088756219,-0.0193592099655948,
-0.012661479609892));
#35175=CARTESIAN_POINT('Ctrl Pts',(0.00235421483873487,-0.0193283761000651,
-0.0131470874883483));
#35176=CARTESIAN_POINT('Ctrl Pts',(0.0020869581343954,-0.0192975252233586,
-0.0135523000691403));
#35177=CARTESIAN_POINT('Ctrl Pts',(0.001994005391597,-0.0192867951890469,
-0.0136932343102256));
#35178=CARTESIAN_POINT('Ctrl Pts',(0.00188680774892241,-0.0192760630969427,
-0.0138245894057865));
#35179=CARTESIAN_POINT('Ctrl Pts',(0.00176769300135974,-0.0192653289288279,
-0.0139436941880376));
#35180=CARTESIAN_POINT('Ctrl Pts',(0.00143152114808729,-0.0192350343997095,
-0.0142798379166879));
#35181=CARTESIAN_POINT('Ctrl Pts',(0.000995098492753798,-0.019204723334944,
-0.0145183453699338));
#35182=CARTESIAN_POINT('Ctrl Pts',(0.000528936678592756,-0.0191743969631418,
-0.0146192578764775));
#35183=CARTESIAN_POINT('Ctrl Pts',(0.000355014062610838,-0.0191630823471504,
-0.0146569078224624));
#35184=CARTESIAN_POINT('Ctrl Pts',(0.000177216695672668,-0.0191517656004221,
-0.0146758695670535));
#35185=CARTESIAN_POINT('Ctrl Pts',(-2.29520690578055E-7,-0.0191404467867643,
-0.0146758532760222));
#35186=CARTESIAN_POINT('Ctrl Pts',(-0.000477621111070754,-0.0191099952698817,
-0.014675809447523));
#35187=CARTESIAN_POINT('Ctrl Pts',(-0.000956528405034772,-0.0190795287926513,
-0.0145347058285624));
#35188=CARTESIAN_POINT('Ctrl Pts',(-0.00135838029685896,-0.0190490427992403,
-0.0142746155334802));
#35189=CARTESIAN_POINT('Ctrl Pts',(-0.00150624544658671,-0.0190378251937692,
-0.0141789128847991));
#35190=CARTESIAN_POINT('Ctrl Pts',(-0.00164381976427042,-0.0190266049459231,
-0.0140676026162161));
#35191=CARTESIAN_POINT('Ctrl Pts',(-0.00176801757635966,-0.0190153818287327,
-0.0139433695805943));
#35192=CARTESIAN_POINT('Ctrl Pts',(-0.00210531564910551,-0.0189849019375425,
-0.0136059758473093));
#35193=CARTESIAN_POINT('Ctrl Pts',(-0.00234407137079544,-0.018954400883096,
-0.0131678879829634));
#35194=CARTESIAN_POINT('Ctrl Pts',(-0.00244439518612312,-0.0189238956125108,
-0.012700193037157));
#35195=CARTESIAN_POINT('Ctrl Pts',(-0.00248140519030315,-0.0189126420513481,
-0.0125276578136636));
#35196=CARTESIAN_POINT('Ctrl Pts',(-0.00250003369489785,-0.0189013879164058,
-0.0123513493333056));
#35197=CARTESIAN_POINT('Ctrl Pts',(-0.00249999995404654,-0.0188901340585108,
-0.0121753739460773));
#35198=CARTESIAN_POINT('Ctrl Pts',(-0.00249990839921447,-0.0188595970379636,
-0.0116978697812211));
#35199=CARTESIAN_POINT('Ctrl Pts',(-0.00235869288269855,-0.0188290620572946,
-0.0112188869879149));
#35200=CARTESIAN_POINT('Ctrl Pts',(-0.00209846725181672,-0.0187985416747736,
-0.0108170173166733));
#35201=CARTESIAN_POINT('Ctrl Pts',(-0.00200282958386128,-0.0187873248772602,
-0.0106693228791603));
#35202=CARTESIAN_POINT('Ctrl Pts',(-0.00189161856248915,-0.0187761100515137,
-0.0105319019889743));
#35203=CARTESIAN_POINT('Ctrl Pts',(-0.00176751057099405,-0.0187648978209337,
-0.0104078299887975));
#35204=CARTESIAN_POINT('Ctrl Pts',(-0.00142992556062184,-0.0187343995352791,
-0.0100703428780802));
#35205=CARTESIAN_POINT('Ctrl Pts',(-0.000991551759118442,-0.0187039204509871,
-0.009831520411939));
#35206=CARTESIAN_POINT('Ctrl Pts',(-0.000523550509890121,-0.0186734572019689,
-0.00973128893608708));
#35207=CARTESIAN_POINT('Ctrl Pts',(-0.00035134857821876,-0.018662248192731,
-0.00969440857778797));
#35208=CARTESIAN_POINT('Ctrl Pts',(-0.000175390128030396,-0.0186510413274082,
-0.00967583603259462));
#35209=CARTESIAN_POINT('Ctrl Pts',(2.45764735002735E-7,-0.0186398364383139,
-0.00967585329863816));
#35210=CARTESIAN_POINT('Ctrl Pts',(0.000475846715698093,-0.0186094949413409,
-0.00967590005301506));
#35211=CARTESIAN_POINT('Ctrl Pts',(0.000953114529689402,-0.01857916793529,
-0.00981598683912423));
#35212=CARTESIAN_POINT('Ctrl Pts',(0.00135398369347432,-0.0185488563282234,
-0.0100742519547624));
#35213=CARTESIAN_POINT('Ctrl Pts',(0.0015034823299754,-0.0185375520316199,
-0.0101705683745117));
#35214=CARTESIAN_POINT('Ctrl Pts',(0.00164249968130742,-0.0185262498767293,
-0.0102828061312865));
#35215=CARTESIAN_POINT('Ctrl Pts',(0.0017678581511007,-0.0185149499106513,
-0.0104081775364312));
#35216=CARTESIAN_POINT('Ctrl Pts',(0.00211031317621986,-0.018484080595052,
-0.0107506678984214));
#35217=CARTESIAN_POINT('Ctrl Pts',(0.00235098525044874,-0.0184532276140454,
-0.0111965061642443));
#35218=CARTESIAN_POINT('Ctrl Pts',(0.00244882647930589,-0.0184223906475597,
-0.0116726148994588));
#35219=CARTESIAN_POINT('Ctrl Pts',(0.00248283735956045,-0.0184116713180213,
-0.0118381164714512));
#35220=CARTESIAN_POINT('Ctrl Pts',(0.00250000059660287,-0.0184009539235939,
-0.0120070464132494));
#35221=CARTESIAN_POINT('Ctrl Pts',(0.00249999999998439,-0.0183902384508335,
-0.0121758621219101));
#35222=CARTESIAN_POINT('',(0.00249999959063015,-0.0173900991833072,-0.0121744179063317));
#35223=CARTESIAN_POINT('Ctrl Pts',(0.00249999903573504,-0.0183900992552675,
-0.0121780490378796));
#35224=CARTESIAN_POINT('Ctrl Pts',(0.00249957249695903,-0.0183591752383259,
-0.0126636898835828));
#35225=CARTESIAN_POINT('Ctrl Pts',(0.00235335328054027,-0.0183282512213843,
-0.0131491781125948));
#35226=CARTESIAN_POINT('Ctrl Pts',(0.00208572997424369,-0.0182973272044428,
-0.0135541603911402));
#35227=CARTESIAN_POINT('Ctrl Pts',(0.00199276069915751,-0.0182865845547177,
-0.0136948466018448));
#35228=CARTESIAN_POINT('Ctrl Pts',(0.00188558847493998,-0.0182758419049926,
-0.0138259636437154));
#35229=CARTESIAN_POINT('Ctrl Pts',(0.0017665348429219,-0.0182650992552675,
-0.0139448514914026));
#35230=CARTESIAN_POINT('Ctrl Pts',(0.00143013698981292,-0.0182347448322822,
-0.0142807809044306));
#35231=CARTESIAN_POINT('Ctrl Pts',(0.000993550900972938,-0.0182043904092969,
-0.0145190032078329));
#35232=CARTESIAN_POINT('Ctrl Pts',(0.00052731742539814,-0.0181740359863115,
-0.0146196078431516));
#35233=CARTESIAN_POINT('Ctrl Pts',(0.00035356526115382,-0.0181627237426302,
-0.0146571003743305));
#35234=CARTESIAN_POINT('Ctrl Pts',(0.000175959535775875,-0.0181514114989488,
-0.0146759442704757));
#35235=CARTESIAN_POINT('Ctrl Pts',(-1.28796846103748E-6,-0.0181400992552675,
-0.0146758529547855));
#35236=CARTESIAN_POINT('Ctrl Pts',(-0.000478659398081885,-0.0181096325812141,
-0.0146756070190147));
#35237=CARTESIAN_POINT('Ctrl Pts',(-0.000957487877102955,-0.0180791659071606,
-0.0145343122044584));
#35238=CARTESIAN_POINT('Ctrl Pts',(-0.00135921802140773,-0.0180486992331071,
-0.0142740730963684));
#35239=CARTESIAN_POINT('Ctrl Pts',(-0.0015068998668508,-0.0180374992404939,
-0.0141784054142588));
#35240=CARTESIAN_POINT('Ctrl Pts',(-0.00164430467893622,-0.0180262992478808,
-0.0140671651195189));
#35241=CARTESIAN_POINT('Ctrl Pts',(-0.0017683566360559,-0.0180150992552675,
-0.0139430303596657));
#35242=CARTESIAN_POINT('Ctrl Pts',(-0.0021057443084893,-0.0179846383135236,
-0.0136054174862585));
#35243=CARTESIAN_POINT('Ctrl Pts',(-0.00234446976288325,-0.0179541773717796,
-0.0131670539246621));
#35244=CARTESIAN_POINT('Ctrl Pts',(-0.00244463034509106,-0.0179237164300356,
-0.0126990955591814));
#35245=CARTESIAN_POINT('Ctrl Pts',(-0.00248147661011304,-0.0179125107051129,
-0.0125269468198901));
#35246=CARTESIAN_POINT('Ctrl Pts',(-0.00250002667142186,-0.0179013049801901,
-0.0123510474891866));
#35247=CARTESIAN_POINT('Ctrl Pts',(-0.00249999997109181,-0.0178900992552675,
-0.0121754731011273));
#35248=CARTESIAN_POINT('Ctrl Pts',(-0.00249992739058463,-0.0178596383135234,
-0.0116982026662986));
#35249=CARTESIAN_POINT('Ctrl Pts',(-0.00235886399483292,-0.0178291773717794,
-0.0112194068467278));
#35250=CARTESIAN_POINT('Ctrl Pts',(-0.0020988613435106,-0.0177987164300353,
-0.0108176261108924));
#35251=CARTESIAN_POINT('Ctrl Pts',(-0.0020032136706863,-0.0177875107051127,
-0.0106698222628437));
#35252=CARTESIAN_POINT('Ctrl Pts',(-0.00189197228786045,-0.01777630498019,
-0.0105322989909189));
#35253=CARTESIAN_POINT('Ctrl Pts',(-0.00176781907028875,-0.0177650992552675,
-0.0104081384524507));
#35254=CARTESIAN_POINT('Ctrl Pts',(-0.00143026521825581,-0.0177346325812141,
-0.0100705646960056));
#35255=CARTESIAN_POINT('Ctrl Pts',(-0.000991893967360312,-0.0177041659071607,
-0.00983165814577795));
#35256=CARTESIAN_POINT('Ctrl Pts',(-0.000523872223124607,-0.0176736992331073,
-0.00973135785930967));
#35257=CARTESIAN_POINT('Ctrl Pts',(-0.0003518206211315,-0.0176624992404941,
-0.00969448601482857));
#35258=CARTESIAN_POINT('Ctrl Pts',(-0.000176016299390968,-0.0176512992478808,
-0.00967589037720141));
#35259=CARTESIAN_POINT('Ctrl Pts',(-5.27597649642248E-7,-0.0176400992552675,
-0.00967585334222996));
#35260=CARTESIAN_POINT('Ctrl Pts',(0.000475085062621117,-0.0176097448322822,
-0.00967575296937904));
#35261=CARTESIAN_POINT('Ctrl Pts',(0.000952405251914807,-0.0175793904092968,
-0.00981569870440331));
#35262=CARTESIAN_POINT('Ctrl Pts',(0.00135335865844833,-0.0175490359863114,
-0.0100738493994059));
#35263=CARTESIAN_POINT('Ctrl Pts',(0.00150278276846154,-0.0175377237426301,
-0.0101700549365618));
#35264=CARTESIAN_POINT('Ctrl Pts',(0.00164174481919509,-0.0175264114989488,
-0.0102821628401217));
#35265=CARTESIAN_POINT('Ctrl Pts',(0.00176707279908354,-0.0175150992552675,
-0.0104073924521772));
#35266=CARTESIAN_POINT('Ctrl Pts',(0.00210967897717657,-0.017484175238326,
-0.0107497297244178));
#35267=CARTESIAN_POINT('Ctrl Pts',(0.00235054853018672,-0.0174532512213847,
-0.0111954593727511));
#35268=CARTESIAN_POINT('Ctrl Pts',(0.0024486017532444,-0.0174223272044432,
-0.0116715225875039));
#35269=CARTESIAN_POINT('Ctrl Pts',(0.00248266432123916,-0.017411584554718,
-0.0118369015023081));
#35270=CARTESIAN_POINT('Ctrl Pts',(0.00249990272492457,-0.0174008419049927,
-0.0120057117944032));
#35271=CARTESIAN_POINT('Ctrl Pts',(0.00249999958793644,-0.0173900992552675,
-0.0121744179058976));
#35272=CARTESIAN_POINT('',(0.00249381958246776,-0.0173787744554382,-0.0123515850776938));
#35273=CARTESIAN_POINT('Origin',(-1.04514259548572E-5,-0.0173843902893253,
-0.0121754854583606));
#35274=CARTESIAN_POINT('',(-0.0005656487160527,-0.0173787743898723,-0.00974068562702664));
#35275=CARTESIAN_POINT('Origin',(0.,-0.0173787743898623,-0.0121758532865581));
#35276=CARTESIAN_POINT('',(0.00249999999193524,-0.0180924405687266,-0.0121757107249461));
#35277=CARTESIAN_POINT('Ctrl Pts',(-0.000565648716059983,-0.0173787743898623,
-0.00974068562702833));
#35278=CARTESIAN_POINT('Ctrl Pts',(-0.00102063502873678,-0.0174085101231125,
-0.00984637133724353));
#35279=CARTESIAN_POINT('Ctrl Pts',(-0.00144474304188495,-0.0174382458563627,
-0.0100828662127555));
#35280=CARTESIAN_POINT('Ctrl Pts',(-0.00177369170692559,-0.0174679815896129,
-0.0104140310115305));
#35281=CARTESIAN_POINT('Ctrl Pts',(-0.00210264037196623,-0.017497717322863,
-0.0107451958103055));
#35282=CARTESIAN_POINT('Ctrl Pts',(-0.00233633893814873,-0.0175274530561132,
-0.0111711335748698));
#35283=CARTESIAN_POINT('Ctrl Pts',(-0.00243891071790016,-0.0175571887893634,
-0.0116265678324346));
#35284=CARTESIAN_POINT('Ctrl Pts',(-0.0025414824976516,-0.0175869245226136,
-0.0120820020899993));
#35285=CARTESIAN_POINT('Ctrl Pts',(-0.00251296309993666,-0.0176166602558637,
-0.0125669427677188));
#35286=CARTESIAN_POINT('Ctrl Pts',(-0.00235772085899037,-0.0176463959891139,
-0.0130072090173266));
#35287=CARTESIAN_POINT('Ctrl Pts',(-0.00220247861804409,-0.0176761317223641,
-0.0134474752669345));
#35288=CARTESIAN_POINT('Ctrl Pts',(-0.00192051160882463,-0.0177058674556142,
-0.0138430567057876));
#35289=CARTESIAN_POINT('Ctrl Pts',(-0.00155496962887267,-0.0177356031888644,
-0.0141334205148503));
#35290=CARTESIAN_POINT('Ctrl Pts',(-0.00118942764892072,-0.0177653389221146,
-0.014423784323913));
#35291=CARTESIAN_POINT('Ctrl Pts',(-0.000740306567027435,-0.0177950746553647,
-0.0146089337847607));
#35292=CARTESIAN_POINT('Ctrl Pts',(-0.000276332539189543,-0.0178248103886149,
-0.0146605344185718));
#35293=CARTESIAN_POINT('Ctrl Pts',(0.000187641488648348,-0.0178545461218651,
-0.014712135052383));
#35294=CARTESIAN_POINT('Ctrl Pts',(0.000666458784610825,-0.0178842818551152,
-0.014630191083476));
#35295=CARTESIAN_POINT('Ctrl Pts',(0.00108687388580177,-0.0179140175883654,
-0.0144272317879128));
#35296=CARTESIAN_POINT('Ctrl Pts',(0.00150728898699271,-0.0179437533216156,
-0.0142242724923496));
#35297=CARTESIAN_POINT('Ctrl Pts',(0.00186930350615625,-0.0179734890548657,
-0.013900260938493));
#35298=CARTESIAN_POINT('Ctrl Pts',(0.00211745136178973,-0.0180032247881159,
-0.0135049130032205));
#35299=CARTESIAN_POINT('Ctrl Pts',(0.00236559817464578,-0.0180329603964093,
-0.0131095667292959));
#35300=CARTESIAN_POINT('Ctrl Pts',(0.00250000021304311,-0.0180626960047028,
-0.0126429497555809));
#35301=CARTESIAN_POINT('Ctrl Pts',(0.00249999999999974,-0.0180924316129961,
-0.0121758521463073));
#35302=CARTESIAN_POINT('',(0.00249999972323816,-0.0190923959387205,-0.0121750282773563));
#35303=CARTESIAN_POINT('Ctrl Pts',(0.00249999998387073,-0.0180924495244571,
-0.012175569303585));
#35304=CARTESIAN_POINT('Ctrl Pts',(0.00249994481879298,-0.0181233634206488,
-0.0116899321120859));
#35305=CARTESIAN_POINT('Ctrl Pts',(0.00235409908043358,-0.0181542773168405,
-0.0112043354005097));
#35306=CARTESIAN_POINT('Ctrl Pts',(0.00208678918439825,-0.0181851912130322,
-0.0107991503774748));
#35307=CARTESIAN_POINT('Ctrl Pts',(0.00199384948267087,-0.0181959395180291,
-0.0106582735309988));
#35308=CARTESIAN_POINT('Ctrl Pts',(0.00188667534136289,-0.018206687823026,
-0.0105269712305407));
#35309=CARTESIAN_POINT('Ctrl Pts',(0.00176759243584567,-0.018217436128023,
-0.010407911833698));
#35310=CARTESIAN_POINT('Ctrl Pts',(0.00143140152045128,-0.0182477803867574,
-0.0100717872872149));
#35311=CARTESIAN_POINT('Ctrl Pts',(0.000994966013488791,-0.0182781246454917,
-0.0098333052659455));
#35312=CARTESIAN_POINT('Ctrl Pts',(0.00052880017530072,-0.0183084689042261,
-0.00973241915104269));
#35313=CARTESIAN_POINT('Ctrl Pts',(0.00035492747743972,-0.0183197868466803,
-0.00969479017968124));
#35314=CARTESIAN_POINT('Ctrl Pts',(0.000177183507666847,-0.0183311047891346,
-0.00967583842259123));
#35315=CARTESIAN_POINT('Ctrl Pts',(-2.0960162221961E-7,-0.0183424227315888,
-0.00967585329534467));
#35316=CARTESIAN_POINT('Ctrl Pts',(-0.00047757315541562,-0.0183728792315804,
-0.00967589331781491));
#35317=CARTESIAN_POINT('Ctrl Pts',(-0.000956456302177873,-0.0184033357315721,
-0.00981697710992422));
#35318=CARTESIAN_POINT('Ctrl Pts',(-0.00135829552168139,-0.0184337922315637,
-0.0100770361730915));
#35319=CARTESIAN_POINT('Ctrl Pts',(-0.00150614212993305,-0.0184449979327607,
-0.0101727183478725));
#35320=CARTESIAN_POINT('Ctrl Pts',(-0.00164370139022194,-0.0184562036339577,
-0.0102840036490499));
#35321=CARTESIAN_POINT('Ctrl Pts',(-0.00176788886171212,-0.0184674093351546,
-0.0104082082507451));
#35322=CARTESIAN_POINT('Ctrl Pts',(-0.00210536041935918,-0.0184978601156729,
-0.0107457263586352));
#35323=CARTESIAN_POINT('Ctrl Pts',(-0.00234420066788555,-0.0185283108961913,
-0.0111840193628629));
#35324=CARTESIAN_POINT('Ctrl Pts',(-0.00244448756983183,-0.0185587616767095,
-0.0116519444004551));
#35325=CARTESIAN_POINT('Ctrl Pts',(-0.00248141137363274,-0.0185699730973799,
-0.0118242258444551));
#35326=CARTESIAN_POINT('Ctrl Pts',(-0.00250000950067293,-0.0185811845180502,
-0.0120002691096592));
#35327=CARTESIAN_POINT('Ctrl Pts',(-0.0024999999963431,-0.0185923959387205,
-0.0121759885068293));
#35328=CARTESIAN_POINT('Ctrl Pts',(-0.00249997418210687,-0.0186228467192388,
-0.0126532511975605));
#35329=CARTESIAN_POINT('Ctrl Pts',(-0.00235896206199205,-0.018653297499757,
-0.0131320547624161));
#35330=CARTESIAN_POINT('Ctrl Pts',(-0.00209900534106159,-0.0186837482802753,
-0.0135338579176971));
#35331=CARTESIAN_POINT('Ctrl Pts',(-0.00200329402907474,-0.0186949597009456,
-0.0136817944935038));
#35332=CARTESIAN_POINT('Ctrl Pts',(-0.00189196193403086,-0.018706171121616,
-0.0138194350006231));
#35333=CARTESIAN_POINT('Ctrl Pts',(-0.00176769763421554,-0.0187173825422863,
-0.0139436895555572));
#35334=CARTESIAN_POINT('Ctrl Pts',(-0.00143012617404289,-0.018747839042278,
-0.0142812345431729));
#35335=CARTESIAN_POINT('Ctrl Pts',(-0.000991746055560251,-0.0187782955422696,
-0.0145201097185846));
#35336=CARTESIAN_POINT('Ctrl Pts',(-0.000523724419950059,-0.0188087520422614,
-0.0146203803843723));
#35337=CARTESIAN_POINT('Ctrl Pts',(-0.000351527660513317,-0.0188199577434583,
-0.0146572724474768));
#35338=CARTESIAN_POINT('Ctrl Pts',(-0.000175573044316863,-0.0188311634446552,
-0.0146758575599681));
#35339=CARTESIAN_POINT('Ctrl Pts',(6.08389199934128E-8,-0.0188423691458522,
-0.0146758532858178));
#35340=CARTESIAN_POINT('Ctrl Pts',(0.00047566516762695,-0.0188727134045866,
-0.0146758417117163));
#35341=CARTESIAN_POINT('Ctrl Pts',(0.000952945835934379,-0.0189030576633209,
-0.0145357883099573));
#35342=CARTESIAN_POINT('Ctrl Pts',(0.0013538351280994,-0.0189334019220553,
-0.0142775503260774));
#35343=CARTESIAN_POINT('Ctrl Pts',(0.00150336067686838,-0.0189447198645095,
-0.0141812315243351));
#35344=CARTESIAN_POINT('Ctrl Pts',(0.00164240318950303,-0.0189560378069638,
-0.0140689863748748));
#35345=CARTESIAN_POINT('Ctrl Pts',(0.00176778367472126,-0.018967355749418,
-0.0139436035176114));
#35346=CARTESIAN_POINT('Ctrl Pts',(0.00211024868725995,-0.0189982696456097,
-0.0136011320260544));
#35347=CARTESIAN_POINT('Ctrl Pts',(0.00235093846666087,-0.0190291835418014,
-0.0131553101000555));
#35348=CARTESIAN_POINT('Ctrl Pts',(0.00244880189405485,-0.0190600974379931,
-0.0126792112940174));
#35349=CARTESIAN_POINT('Ctrl Pts',(0.00248282756196641,-0.01907084574299,
-0.0125136787728425));
#35350=CARTESIAN_POINT('Ctrl Pts',(0.0024999990853136,-0.0190815940479869,
-0.01234471570696));
#35351=CARTESIAN_POINT('Ctrl Pts',(0.00249999999996332,-0.0190923423529838,
-0.0121758668289893));
#35352=CARTESIAN_POINT('',(0.00249999972741721,-0.0200925477005089,-0.0121764841472801));
#35353=CARTESIAN_POINT('Ctrl Pts',(0.00249999944651301,-0.0190924495244571,
-0.0121741897257233));
#35354=CARTESIAN_POINT('Ctrl Pts',(0.00249967628899577,-0.0191233739581301,
-0.0116885485653149));
#35355=CARTESIAN_POINT('Ctrl Pts',(0.00235356029135108,-0.0191542983918031,
-0.0112030290255191));
#35356=CARTESIAN_POINT('Ctrl Pts',(0.00208602297944995,-0.0191852228254761,
-0.0107979896760339));
#35357=CARTESIAN_POINT('Ctrl Pts',(0.00199308843554419,-0.0191959650584697,
-0.010657290993892));
#35358=CARTESIAN_POINT('Ctrl Pts',(0.00188595038429507,-0.0192067072914634,
-0.0105261574625068));
#35359=CARTESIAN_POINT('Ctrl Pts',(0.00176692942331025,-0.0192174495244571,
-0.0104072492005511));
#35360=CARTESIAN_POINT('Ctrl Pts',(0.00143060615072211,-0.0192478043705736,
-0.0100712443870478));
#35361=CARTESIAN_POINT('Ctrl Pts',(0.000994072722768003,-0.0192781592166902,
-0.00983292461567489));
#35362=CARTESIAN_POINT('Ctrl Pts',(0.000527861249261944,-0.0193085140628067,
-0.00973221614051378));
#35363=CARTESIAN_POINT('Ctrl Pts',(0.000354126205227666,-0.0193198258833568,
-0.00969468683812412));
#35364=CARTESIAN_POINT('Ctrl Pts',(0.000176533840600821,-0.019331137703907,
-0.00967580342092681));
#35365=CARTESIAN_POINT('Ctrl Pts',(-7.04769819689285E-7,-0.0193424495244571,
-0.0096758533858982));
#35366=CARTESIAN_POINT('Ctrl Pts',(-0.000478076729573463,-0.0193729166215054,
-0.00967598796084355));
#35367=CARTESIAN_POINT('Ctrl Pts',(-0.000956938538252152,-0.0194033837185538,
-0.00981717134421778));
#35368=CARTESIAN_POINT('Ctrl Pts',(-0.00135872957220158,-0.0194338508156022,
-0.0100773171420934));
#35369=CARTESIAN_POINT('Ctrl Pts',(-0.00150642617255667,-0.0194450503852205,
-0.0101729455824924));
#35370=CARTESIAN_POINT('Ctrl Pts',(-0.00164385041494005,-0.0194562499548387,
-0.0102841474371042));
#35371=CARTESIAN_POINT('Ctrl Pts',(-0.00176792630945377,-0.0194674495244571,
-0.0104082457044457));
#35372=CARTESIAN_POINT('Ctrl Pts',(-0.00210539650822995,-0.0194979108884482,
-0.0107457767543861));
#35373=CARTESIAN_POINT('Ctrl Pts',(-0.00234422876329441,-0.0195283722524392,
-0.0111840826282489));
#35374=CARTESIAN_POINT('Ctrl Pts',(-0.00244450313034634,-0.0195588336164303,
-0.0116520170089608));
#35375=CARTESIAN_POINT('Ctrl Pts',(-0.00248138935230773,-0.0195700389191059,
-0.0118241480523946));
#35376=CARTESIAN_POINT('Ctrl Pts',(-0.00249998214814256,-0.0195812442217815,
-0.0120000337511903));
#35377=CARTESIAN_POINT('Ctrl Pts',(-0.00249999998709464,-0.0195924495244571,
-0.012175599265259));
#35378=CARTESIAN_POINT('Ctrl Pts',(-0.00250004848188573,-0.0196229108884482,
-0.0126528701773575));
#35379=CARTESIAN_POINT('Ctrl Pts',(-0.0023591062861405,-0.0196533722524392,
-0.0131317021386709));
#35380=CARTESIAN_POINT('Ctrl Pts',(-0.00209920516654239,-0.0196838336164303,
-0.0135335490067995));
#35381=CARTESIAN_POINT('Ctrl Pts',(-0.0020035997723886,-0.0196950389191059,
-0.0136813695636186));
#35382=CARTESIAN_POINT('Ctrl Pts',(-0.00189239965550865,-0.0197062442217815,
-0.0138189145415262));
#35383=CARTESIAN_POINT('Ctrl Pts',(-0.00176828548092616,-0.0197174495244571,
-0.0139431015594235));
#35384=CARTESIAN_POINT('Ctrl Pts',(-0.00143082037966594,-0.0197479166215054,
-0.0142807647208706));
#35385=CARTESIAN_POINT('Ctrl Pts',(-0.000992511726133087,-0.0197783837185537,
-0.0145197870193782));
#35386=CARTESIAN_POINT('Ctrl Pts',(-0.000524516037558449,-0.0198088508156021,
-0.0146202106512542));
#35387=CARTESIAN_POINT('Ctrl Pts',(-0.000352482900073631,-0.0198200503852204,
-0.0146571259325079));
#35388=CARTESIAN_POINT('Ctrl Pts',(-0.000176692611848837,-0.0198312499548388,
-0.014675767862736));
#35389=CARTESIAN_POINT('Ctrl Pts',(-1.21281238046647E-6,-0.0198424495244571,
-0.0146758529923753));
#35390=CARTESIAN_POINT('Ctrl Pts',(0.000474400313029194,-0.0198728043705736,
-0.0146760837241972));
#35391=CARTESIAN_POINT('Ctrl Pts',(0.000951759243660809,-0.0199031592166902,
-0.0145362685350562));
#35392=CARTESIAN_POINT('Ctrl Pts',(0.00135278359530711,-0.0199335140628067,
-0.0142782273123366));
#35393=CARTESIAN_POINT('Ctrl Pts',(0.00150222647123657,-0.0199448258833568,
-0.0141820675098875));
#35394=CARTESIAN_POINT('Ctrl Pts',(0.00164121270041218,-0.019956137703907,
-0.0140700040924385));
#35395=CARTESIAN_POINT('Ctrl Pts',(0.00176656997634155,-0.0199674495244571,
-0.01394481640621));
#35396=CARTESIAN_POINT('Ctrl Pts',(0.00210927367710781,-0.0199983739581303,
-0.0136025763324464));
#35397=CARTESIAN_POINT('Ctrl Pts',(0.00235026996938759,-0.0200292983918035,
-0.0131569149011769));
#35398=CARTESIAN_POINT('Ctrl Pts',(0.00244845842858246,-0.0200602228254768,
-0.0126808793487603));
#35399=CARTESIAN_POINT('Ctrl Pts',(0.00248256619324154,-0.0200709650584702,
-0.0125155186869849));
#35400=CARTESIAN_POINT('Ctrl Pts',(0.00249985251929391,-0.0200817072914636,
-0.0123467222292437));
#35401=CARTESIAN_POINT('Ctrl Pts',(0.00249999905682766,-0.0200924495244571,
-0.0121780248898416));
#35402=CARTESIAN_POINT('',(0.00249999999999813,-0.0210924016317463,-0.0121758502265542));
#35403=CARTESIAN_POINT('Ctrl Pts',(0.00249999999999579,-0.0200925876067202,
-0.0121758578723672));
#35404=CARTESIAN_POINT('Ctrl Pts',(0.00250000088291571,-0.0201232524092462,
-0.0116945251893599));
#35405=CARTESIAN_POINT('Ctrl Pts',(0.00235859969628574,-0.0201525642010006,
-0.0112380345259211));
#35406=CARTESIAN_POINT('Ctrl Pts',(0.00209855644319116,-0.0201841557313721,
-0.0108159596537342));
#35407=CARTESIAN_POINT('Ctrl Pts',(0.00206718492720256,-0.0201877656541674,
-0.0107687593266094));
#35408=CARTESIAN_POINT('Ctrl Pts',(0.00175006943670304,-0.0202225469736906,
-0.0103247030656945));
#35409=CARTESIAN_POINT('Ctrl Pts',(0.0013651500455325,-0.0202520137354763,
-0.010036664202749));
#35410=CARTESIAN_POINT('Ctrl Pts',(0.000561164206619752,-0.0203074924422943,
-0.00970100797496499));
#35411=CARTESIAN_POINT('Ctrl Pts',(0.000143409931365646,-0.0203335043873267,
-0.00965099224594665));
#35412=CARTESIAN_POINT('Ctrl Pts',(-0.000616036517871959,-0.0203820729533282,
-0.00972310203715264));
#35413=CARTESIAN_POINT('Ctrl Pts',(-0.000957753383009871,-0.0204046295742975,
-0.0098435059109142));
#35414=CARTESIAN_POINT('Ctrl Pts',(-0.0015259109359658,-0.0204462893830545,
-0.0101686832292785));
#35415=CARTESIAN_POINT('Ctrl Pts',(-0.00175283236942671,-0.0204653925708423,
-0.0103724766563074));
#35416=CARTESIAN_POINT('Ctrl Pts',(-0.00210085664408624,-0.0205001384570194,
-0.0107934676866464));
#35417=CARTESIAN_POINT('Ctrl Pts',(-0.00222243362220393,-0.0205157811554087,
-0.0110101717401975));
#35418=CARTESIAN_POINT('Ctrl Pts',(-0.00234911679547337,-0.0205366695864338,
-0.0113134981106694));
#35419=CARTESIAN_POINT('Ctrl Pts',(-0.00238204707436731,-0.0205432031273489,
-0.0114109864453164));
#35420=CARTESIAN_POINT('Ctrl Pts',(-0.00243357549085177,-0.0205553781071763,
-0.0115954397446258));
#35421=CARTESIAN_POINT('Ctrl Pts',(-0.0024522147205405,-0.0205610195460884,
-0.011682387300099));
#35422=CARTESIAN_POINT('Ctrl Pts',(-0.00247950787235856,-0.020571546984231,
-0.0118458435498237));
#35423=CARTESIAN_POINT('Ctrl Pts',(-0.00248801985791747,-0.0205764329834614,
-0.0119223870026145));
#35424=CARTESIAN_POINT('Ctrl Pts',(-0.00249552276806611,-0.0205828105879445,
-0.0120225949860141));
#35425=CARTESIAN_POINT('Ctrl Pts',(-0.00249723367102841,-0.0205847778903784,
-0.0120535529673888));
#35426=CARTESIAN_POINT('Ctrl Pts',(-0.00249902446490594,-0.0205879816792375,
-0.012104019675008));
#35427=CARTESIAN_POINT('Ctrl Pts',(-0.00249943337907817,-0.0205890917480586,
-0.0121215172175532));
#35428=CARTESIAN_POINT('Ctrl Pts',(-0.00249981312615746,-0.0205904789322726,
-0.0121433885497522));
#35429=CARTESIAN_POINT('Ctrl Pts',(-0.00249999256379323,-0.0205907560476657,
-0.0121477556401092));
#35430=CARTESIAN_POINT('Ctrl Pts',(-0.00250000725685106,-0.0205942339146019,
-0.012202611695506));
#35431=CARTESIAN_POINT('Ctrl Pts',(-0.00249920257363735,-0.0205974346661451,
-0.0122531107066766));
#35432=CARTESIAN_POINT('Ctrl Pts',(-0.0024948669570304,-0.0206030813157931,
-0.01234204919432));
#35433=CARTESIAN_POINT('Ctrl Pts',(-0.00249192331425481,-0.020605527213898,
-0.0123805224298522));
#35434=CARTESIAN_POINT('Ctrl Pts',(-0.00248031131675541,-0.0206130664403408,
-0.0124988715853413));
#35435=CARTESIAN_POINT('Ctrl Pts',(-0.00246824224566287,-0.020618361300807,
-0.01258158571656));
#35436=CARTESIAN_POINT('Ctrl Pts',(-0.00241993022737028,-0.0206341006264045,
-0.0128249234266664));
#35437=CARTESIAN_POINT('Ctrl Pts',(-0.00237242236421832,-0.0206443998357345,
-0.0129809906837992));
#35438=CARTESIAN_POINT('Ctrl Pts',(-0.00224761580526192,-0.0206651083145812,
-0.0132825859980184));
#35439=CARTESIAN_POINT('Ctrl Pts',(-0.00217004468113035,-0.020675517584098,
-0.0134279412711221));
#35440=CARTESIAN_POINT('Ctrl Pts',(-0.00198816583959298,-0.0206963137002469,
-0.013700325271695));
#35441=CARTESIAN_POINT('Ctrl Pts',(-0.00188391087056668,-0.020706700546879,
-0.0138274099627527));
#35442=CARTESIAN_POINT('Ctrl Pts',(-0.00153699680145617,-0.0207378762373913,
-0.0141745226749268));
#35443=CARTESIAN_POINT('Ctrl Pts',(-0.00125969929053859,-0.0207586802318874,
-0.0143599649981351));
#35444=CARTESIAN_POINT('Ctrl Pts',(-0.000654815182332665,-0.0208003032688987,
-0.0146106845637142));
#35445=CARTESIAN_POINT('Ctrl Pts',(-0.000327493358863664,-0.0208211223114141,
-0.0146757914697553));
#35446=CARTESIAN_POINT('Ctrl Pts',(0.000478376746627,-0.0208724523882349,
-0.0146759436934712));
#35447=CARTESIAN_POINT('Ctrl Pts',(0.000958122796932754,-0.0209029755972295,
-0.0145341502276829));
#35448=CARTESIAN_POINT('Ctrl Pts',(0.0015072169308343,-0.0209446959549672,
-0.0141781084150004));
#35449=CARTESIAN_POINT('Ctrl Pts',(0.00164404399136796,-0.0209558741894894,
-0.0140673205596144));
#35450=CARTESIAN_POINT('Ctrl Pts',(0.00210759434674393,-0.0209978211139755,
-0.0136038550902574));
#35451=CARTESIAN_POINT('Ctrl Pts',(0.00234767621310324,-0.0210286086970427,
-0.0131616003846502));
#35452=CARTESIAN_POINT('Ctrl Pts',(0.00248215348338499,-0.0210704099800494,
-0.0125202443438541));
#35453=CARTESIAN_POINT('Ctrl Pts',(0.00250000021067322,-0.0210814043918721,
-0.012347970180121));
#35454=CARTESIAN_POINT('Ctrl Pts',(0.00249999999999813,-0.0210924016317463,
-0.0121758502265542));
#35455=CARTESIAN_POINT('',(0.0024999998213867,-0.022092406279442,-0.012175193061947));
#35456=CARTESIAN_POINT('Ctrl Pts',(0.00249999988477308,-0.0210924495244571,
-0.0121750942512416));
#35457=CARTESIAN_POINT('Ctrl Pts',(0.00249985243829347,-0.0211233650347228,
-0.0116894565292411));
#35458=CARTESIAN_POINT('Ctrl Pts',(0.00235391411686965,-0.0211542805449884,
-0.0112038870833032));
#35459=CARTESIAN_POINT('Ctrl Pts',(0.00208652671078272,-0.0211851960552541,
-0.0107987526057108));
#35460=CARTESIAN_POINT('Ctrl Pts',(0.00199357142069997,-0.0211959436079039,
-0.0106579105464745));
#35461=CARTESIAN_POINT('Ctrl Pts',(0.00188638697405189,-0.0212066911605536,
-0.0105266434104093));
#35462=CARTESIAN_POINT('Ctrl Pts',(0.00176729866884987,-0.0212174387132034,
-0.0104076181734915));
#35463=CARTESIAN_POINT('Ctrl Pts',(0.0014310510541324,-0.0212477845892019,
-0.0100715486330199));
#35464=CARTESIAN_POINT('Ctrl Pts',(0.000994574777890654,-0.0212781304652003,
-0.00983313893831883));
#35465=CARTESIAN_POINT('Ctrl Pts',(0.00052839112564458,-0.0213084763411988,
-0.00973233066167));
#35466=CARTESIAN_POINT('Ctrl Pts',(0.000354532657022751,-0.0213197935281157,
-0.00969473523652343));
#35467=CARTESIAN_POINT('Ctrl Pts',(0.0001768069587554,-0.0213311107150327,
-0.0096758132432822));
#35468=CARTESIAN_POINT('Ctrl Pts',(-5.65296794099548E-7,-0.0213424279019496,
-0.00967585335047019));
#35469=CARTESIAN_POINT('Ctrl Pts',(-0.000477929976962419,-0.02137288602121,
-0.00967596129156228));
#35470=CARTESIAN_POINT('Ctrl Pts',(-0.000956793938650606,-0.0214033441404702,
-0.00981711385692225));
#35471=CARTESIAN_POINT('Ctrl Pts',(-0.00135859660307426,-0.0214338022597306,
-0.0100772310551608));
#35472=CARTESIAN_POINT('Ctrl Pts',(-0.00150641190896486,-0.0214450072033856,
-0.0101729230617834));
#35473=CARTESIAN_POINT('Ctrl Pts',(-0.0016439400878006,-0.0214562121470408,
-0.0102842129945245));
#35474=CARTESIAN_POINT('Ctrl Pts',(-0.00176809815021911,-0.0214674170906958,
-0.0104084175929071));
#35475=CARTESIAN_POINT('Ctrl Pts',(-0.00210553052273885,-0.0214978694886136,
-0.0107459764392172));
#35476=CARTESIAN_POINT('Ctrl Pts',(-0.00234431904705325,-0.0215283218865315,
-0.0111842987747312));
#35477=CARTESIAN_POINT('Ctrl Pts',(-0.00244455018892782,-0.0215587742844493,
-0.0116522366578946));
#35478=CARTESIAN_POINT('Ctrl Pts',(-0.00248144901564452,-0.0215699849494469,
-0.0118245020690442));
#35479=CARTESIAN_POINT('Ctrl Pts',(-0.00250002608530036,-0.0215811956144444,
-0.0120005262168479));
#35480=CARTESIAN_POINT('Ctrl Pts',(-0.00249999997238889,-0.021592406279442,
-0.0121762248448264));
#35481=CARTESIAN_POINT('Ctrl Pts',(-0.00249992903986427,-0.0216228586773597,
-0.0126534886408611));
#35482=CARTESIAN_POINT('Ctrl Pts',(-0.00235887103208122,-0.0216533110752775,
-0.0131322797429597));
#35483=CARTESIAN_POINT('Ctrl Pts',(-0.00209887538814559,-0.0216837634731953,
-0.0135340587588769));
#35484=CARTESIAN_POINT('Ctrl Pts',(-0.00200316128139836,-0.0216949741381929,
-0.0136819686201198));
#35485=CARTESIAN_POINT('Ctrl Pts',(-0.00189183109921226,-0.0217061848031906,
-0.0138195833748683));
#35486=CARTESIAN_POINT('Ctrl Pts',(-0.00176757270783774,-0.0217173954681882,
-0.0139438144633115));
#35487=CARTESIAN_POINT('Ctrl Pts',(-0.00142997659695858,-0.0217478535874485,
-0.0142813363951889));
#35488=CARTESIAN_POINT('Ctrl Pts',(-0.000991578519381806,-0.0217783117067088,
-0.0145201807728917));
#35489=CARTESIAN_POINT('Ctrl Pts',(-0.000523548797234617,-0.0218087698259691,
-0.0146204180038266));
#35490=CARTESIAN_POINT('Ctrl Pts',(-0.000351369857991001,-0.0218199747696242,
-0.0146572933116937));
#35491=CARTESIAN_POINT('Ctrl Pts',(-0.000175435271197161,-0.0218311797132794,
-0.0146758657712238));
#35492=CARTESIAN_POINT('Ctrl Pts',(1.77819740284356E-7,-0.0218423846569345,
-0.0146758532802341));
#35493=CARTESIAN_POINT('Ctrl Pts',(0.00047578334220584,-0.021872730532933,
-0.0146758194514139));
#35494=CARTESIAN_POINT('Ctrl Pts',(0.000953058397251753,-0.0219030764089314,
-0.0145357430466052));
#35495=CARTESIAN_POINT('Ctrl Pts',(0.00135393608389562,-0.0219334222849299,
-0.0142774852906743));
#35496=CARTESIAN_POINT('Ctrl Pts',(0.00150343935448162,-0.0219447394718468,
-0.0141811706778827));
#35497=CARTESIAN_POINT('Ctrl Pts',(0.00164246131298928,-0.0219560566587638,
-0.0140689339964588));
#35498=CARTESIAN_POINT('Ctrl Pts',(0.00176782419267002,-0.0219673738456807,
-0.0139435629979674));
#35499=CARTESIAN_POINT('Ctrl Pts',(0.00211028185658907,-0.0219982893559464,
-0.0136010831556415));
#35500=CARTESIAN_POINT('Ctrl Pts',(0.00235096149551733,-0.022029204866212,
-0.0131552550642329));
#35501=CARTESIAN_POINT('Ctrl Pts',(0.00244881377882811,-0.0220601203764777,
-0.012679153471956));
#35502=CARTESIAN_POINT('Ctrl Pts',(0.00248283141456312,-0.0220708679291274,
-0.0125136402106303));
#35503=CARTESIAN_POINT('Ctrl Pts',(0.00249999892493164,-0.0220816154817772,
-0.0123446976407022));
#35504=CARTESIAN_POINT('Ctrl Pts',(0.00249999999994932,-0.0220923630344269,
-0.0121758692053469));
#35505=CARTESIAN_POINT('',(0.00249999957091393,-0.0230925272726456,-0.0121768329188578));
#35506=CARTESIAN_POINT('Ctrl Pts',(0.00249999964282408,-0.0220924495244571,
-0.0121745169185471));
#35507=CARTESIAN_POINT('Ctrl Pts',(0.00249974004482518,-0.0221233733501191,
-0.0116888760627414));
#35508=CARTESIAN_POINT('Ctrl Pts',(0.00235368778652483,-0.022154297175781,
-0.0112033376886623));
#35509=CARTESIAN_POINT('Ctrl Pts',(0.00208620381233168,-0.022185221001443,
-0.0107982634878833));
#35510=CARTESIAN_POINT('Ctrl Pts',(0.00199328071033653,-0.0221959638424477,
-0.0106575419684423));
#35511=CARTESIAN_POINT('Ctrl Pts',(0.00188615069187808,-0.0222067066834524,
-0.0105263851913197));
#35512=CARTESIAN_POINT('Ctrl Pts',(0.00176713455698379,-0.0222174495244571,
-0.0104074541637598));
#35513=CARTESIAN_POINT('Ctrl Pts',(0.00143085079516353,-0.0222478037532254,
-0.0100714108753393));
#35514=CARTESIAN_POINT('Ctrl Pts',(0.000994345731519502,-0.0222781579819937,
-0.00983304058934352));
#35515=CARTESIAN_POINT('Ctrl Pts',(0.000528146602411794,-0.022308512210762,
-0.00973227779839309));
#35516=CARTESIAN_POINT('Ctrl Pts',(0.000354403143582682,-0.0223198246486604,
-0.00969472544205448));
#35517=CARTESIAN_POINT('Ctrl Pts',(0.000176799616673616,-0.0223311370865588,
-0.00967582128046176));
#35518=CARTESIAN_POINT('Ctrl Pts',(-4.51998086409324E-7,-0.0223424495244571,
-0.00967585332741856));
#35519=CARTESIAN_POINT('Ctrl Pts',(-0.000477823260289689,-0.022372916004356,
-0.00967593963577877));
#35520=CARTESIAN_POINT('Ctrl Pts',(-0.000956698784724591,-0.0224033824842549,
-0.00981707420232769));
#35521=CARTESIAN_POINT('Ctrl Pts',(-0.00135851583923652,-0.0224338489641538,
-0.0100771787728368));
#35522=CARTESIAN_POINT('Ctrl Pts',(-0.00150623313614594,-0.0224450491509216,
-0.0101727992638984));
#35523=CARTESIAN_POINT('Ctrl Pts',(-0.00164367812918537,-0.0224562493376893,
-0.0102839965356232));
#35524=CARTESIAN_POINT('Ctrl Pts',(-0.00176777389185949,-0.0224674495244571,
-0.0104080932725121));
#35525=CARTESIAN_POINT('Ctrl Pts',(-0.00210527270547203,-0.02249791027239,
-0.0107455947356616));
#35526=CARTESIAN_POINT('Ctrl Pts',(-0.00234414264356883,-0.022528371020323,
-0.0111838793575966));
#35527=CARTESIAN_POINT('Ctrl Pts',(-0.00244445757818406,-0.0225588317682559,
-0.0116518044830498));
#35528=CARTESIAN_POINT('Ctrl Pts',(-0.00248136149819129,-0.0225700376869897,
-0.0118239450667558));
#35529=CARTESIAN_POINT('Ctrl Pts',(-0.00249996959653367,-0.0225812436057234,
-0.0119998424534536));
#35530=CARTESIAN_POINT('Ctrl Pts',(-0.00249999996261091,-0.0225924495244571,
-0.0121754209146634));
#35531=CARTESIAN_POINT('Ctrl Pts',(-0.0025000825059031,-0.0226229102723899,
-0.0126526911302003));
#35532=CARTESIAN_POINT('Ctrl Pts',(-0.00235917485964853,-0.0226533710203227,
-0.0131315326026438));
#35533=CARTESIAN_POINT('Ctrl Pts',(-0.00209930299428055,-0.0226838317682555,
-0.0135333977382077));
#35534=CARTESIAN_POINT('Ctrl Pts',(-0.00200370117219264,-0.0226950376869894,
-0.013681236132099));
#35535=CARTESIAN_POINT('Ctrl Pts',(-0.0018925015674253,-0.0227062436057232,
-0.013818798540917));
#35536=CARTESIAN_POINT('Ctrl Pts',(-0.00176838524989491,-0.0227174495244571,
-0.0139430017262638));
#35537=CARTESIAN_POINT('Ctrl Pts',(-0.00143093971035745,-0.022747916004356,
-0.0142806834406874));
#35538=CARTESIAN_POINT('Ctrl Pts',(-0.000992645225224244,-0.0227783824842549,
-0.0145197303711406));
#35539=CARTESIAN_POINT('Ctrl Pts',(-0.000524655831827541,-0.0228088489641538,
-0.0146201806496847));
#35540=CARTESIAN_POINT('Ctrl Pts',(-0.000352612043744256,-0.0228200491509216,
-0.0146571085089024));
#35541=CARTESIAN_POINT('Ctrl Pts',(-0.000176809501660097,-0.0228312493376894,
-0.0146757605083209));
#35542=CARTESIAN_POINT('Ctrl Pts',(-1.31674182171623E-6,-0.0228424495244571,
-0.0146758529397963));
#35543=CARTESIAN_POINT('Ctrl Pts',(0.000474295628738454,-0.0228728037532255,
-0.0146761034433107));
#35544=CARTESIAN_POINT('Ctrl Pts',(0.000951659784619451,-0.0229031579819938,
-0.0145363085163652));
#35545=CARTESIAN_POINT('Ctrl Pts',(0.00135269456445851,-0.0229335122107622,
-0.0142782845970376));
#35546=CARTESIAN_POINT('Ctrl Pts',(0.00150215252224747,-0.0229448246486605,
-0.0141821240394448));
#35547=CARTESIAN_POINT('Ctrl Pts',(0.00164115295742169,-0.0229561370865589,
-0.0140700570709453));
#35548=CARTESIAN_POINT('Ctrl Pts',(0.00176652276641499,-0.0229674495244571,
-0.0139448635510104));
#35549=CARTESIAN_POINT('Ctrl Pts',(0.00210923528792769,-0.022998373350119,
-0.0136026329355339));
#35550=CARTESIAN_POINT('Ctrl Pts',(0.00235024342465923,-0.023029297175781,
-0.013156978340393));
#35551=CARTESIAN_POINT('Ctrl Pts',(0.00244844473207978,-0.0230602210014429,
-0.0126809457473519));
#35552=CARTESIAN_POINT('Ctrl Pts',(0.00248255956132539,-0.0230709638424477,
-0.0125155735027911));
#35553=CARTESIAN_POINT('Ctrl Pts',(0.00249985049107578,-0.0230817066834523,
-0.0123467644820629));
#35554=CARTESIAN_POINT('Ctrl Pts',(0.00249999903102137,-0.0230924495244571,
-0.0121780543981421));
#35555=CARTESIAN_POINT('',(0.00250015411382638,-0.02409267137066,-0.0121754468914277));
#35556=CARTESIAN_POINT('Ctrl Pts',(0.00249999999998422,-0.0230925890616768,
-0.0121758621692742));
#35557=CARTESIAN_POINT('Ctrl Pts',(0.00250000171777091,-0.0231233655601217,
-0.0116923989266971));
#35558=CARTESIAN_POINT('Ctrl Pts',(0.00235737737085954,-0.0231527215417898,
-0.0112349651717997));
#35559=CARTESIAN_POINT('Ctrl Pts',(0.00212674943784686,-0.0231806570105422,
-0.0108617236017027));
#35560=CARTESIAN_POINT('Ctrl Pts',(0.00205135317620363,-0.0231897895986188,
-0.010739704474585));
#35561=CARTESIAN_POINT('Ctrl Pts',(0.00196673295883021,-0.0231987703694879,
-0.0106262870985233));
#35562=CARTESIAN_POINT('Ctrl Pts',(0.0018751024366552,-0.0232075993232843,
-0.0105223748766447));
#35563=CARTESIAN_POINT('Ctrl Pts',(0.00156402163431762,-0.0232375731569542,
-0.0101695983499222));
#35564=CARTESIAN_POINT('Ctrl Pts',(0.00117274164898975,-0.0232657971974777,
-0.00992911309264385));
#35565=CARTESIAN_POINT('Ctrl Pts',(0.000777232675165815,-0.0232922714290193,
-0.00979974104833058));
#35566=CARTESIAN_POINT('Ctrl Pts',(0.000699884479445959,-0.0232974488944583,
-0.00977444024641079));
#35567=CARTESIAN_POINT('Ctrl Pts',(0.000622300010692386,-0.0233025594364456,
-0.00975324549795641));
#35568=CARTESIAN_POINT('Ctrl Pts',(0.000544923280299288,-0.0233076030548627,
-0.00973596422789419));
#35569=CARTESIAN_POINT('Ctrl Pts',(0.000104622388244895,-0.0233363030228884,
-0.00963762770494246));
#35570=CARTESIAN_POINT('Ctrl Pts',(-0.00032401863768543,-0.0233628359980385,
-0.00966754509154558));
#35571=CARTESIAN_POINT('Ctrl Pts',(-0.000691942356854824,-0.0233872020603341,
-0.00977351780316071));
#35572=CARTESIAN_POINT('Ctrl Pts',(-0.000719292763144957,-0.0233890133643321,
-0.00978139551412994));
#35573=CARTESIAN_POINT('Ctrl Pts',(-0.000746330545010817,-0.023390812693939,
-0.0097896890216873));
#35574=CARTESIAN_POINT('Ctrl Pts',(-0.000773046138872332,-0.0233926000491877,
-0.0097983757015587));
#35575=CARTESIAN_POINT('Ctrl Pts',(-0.00115914581460374,-0.0234184313028566,
-0.00992391752177489));
#35576=CARTESIAN_POINT('Ctrl Pts',(-0.00147308347060864,-0.0234417615118279,
-0.0101295750295813));
#35577=CARTESIAN_POINT('Ctrl Pts',(-0.00171174468177345,-0.0234625903062594,
-0.0103537857399451));
#35578=CARTESIAN_POINT('Ctrl Pts',(-0.00195040589293826,-0.0234834191006908,
-0.0105779964503089));
#35579=CARTESIAN_POINT('Ctrl Pts',(-0.00211476129448352,-0.0235017464805822,
-0.0108194934548951));
#35580=CARTESIAN_POINT('Ctrl Pts',(-0.00222770154972694,-0.0235175738260776,
-0.0110412406630851));
#35581=CARTESIAN_POINT('Ctrl Pts',(-0.00234064180497036,-0.0235334011715729,
-0.0112629878712752));
#35582=CARTESIAN_POINT('Ctrl Pts',(-0.00240271876911905,-0.0235467284826722,
-0.011464576329171));
#35583=CARTESIAN_POINT('Ctrl Pts',(-0.00243983608043265,-0.0235575506086425,
-0.0116306928508889));
#35584=CARTESIAN_POINT('Ctrl Pts',(-0.00245839473608945,-0.0235629616716276,
-0.0117137511117478));
#35585=CARTESIAN_POINT('Ctrl Pts',(-0.00247059122038172,-0.0235677464383304,
-0.0117879608720915));
#35586=CARTESIAN_POINT('Ctrl Pts',(-0.00247904539026384,-0.0235719114734548,
-0.0118528456194485));
#35587=CARTESIAN_POINT('Ctrl Pts',(-0.00248749956014596,-0.0235760765085792,
-0.0119177303668055));
#35588=CARTESIAN_POINT('Ctrl Pts',(-0.0024921973665701,-0.0235796218121251,
-0.0119732972404837));
#35589=CARTESIAN_POINT('Ctrl Pts',(-0.00249506056939557,-0.0235825206539539,
-0.0120187776517592));
#35590=CARTESIAN_POINT('Ctrl Pts',(-0.0024964921708083,-0.0235839700748683,
-0.012041517857397));
#35591=CARTESIAN_POINT('Ctrl Pts',(-0.00249746073549553,-0.0235852578803534,
-0.0120617362495059));
#35592=CARTESIAN_POINT('Ctrl Pts',(-0.00249816045946761,-0.0235864183625859,
-0.0120799662762149));
#35593=CARTESIAN_POINT('Ctrl Pts',(-0.0024988601834397,-0.0235875788448184,
-0.0120981963029239));
#35594=CARTESIAN_POINT('Ctrl Pts',(-0.00249927457514363,-0.0235886120037982,
-0.0121144391812369));
#35595=CARTESIAN_POINT('Ctrl Pts',(-0.00249951245441347,-0.0235893781501396,
-0.0121264823413376));
#35596=CARTESIAN_POINT('Ctrl Pts',(-0.00249975033368331,-0.023590144296481,
-0.0121385255014383));
#35597=CARTESIAN_POINT('Ctrl Pts',(-0.00249984712543923,-0.0235906434301841,
-0.0121463673677798));
#35598=CARTESIAN_POINT('Ctrl Pts',(-0.00249992599526052,-0.0235912943128788,
-0.0121566174288783));
#35599=CARTESIAN_POINT('Ctrl Pts',(-0.00249996543017117,-0.0235916197542261,
-0.0121617424594276));
#35600=CARTESIAN_POINT('Ctrl Pts',(-0.00249997734888517,-0.0235918394918372,
-0.0121652016109821));
#35601=CARTESIAN_POINT('Ctrl Pts',(-0.00249997918792211,-0.023591868492253,
-0.012165652308355));
#35602=CARTESIAN_POINT('Ctrl Pts',(-0.00249998102695905,-0.0235918974926687,
-0.0121661030057279));
#35603=CARTESIAN_POINT('Ctrl Pts',(-0.00250002847430832,-0.0235921907273404,
-0.012170729115383));
#35604=CARTESIAN_POINT('Ctrl Pts',(-0.00249998763931371,-0.0235930136443261,
-0.0121837147926892));
#35605=CARTESIAN_POINT('Ctrl Pts',(-0.00249994680431911,-0.0235938365613117,
-0.0121967004699954));
#35606=CARTESIAN_POINT('Ctrl Pts',(-0.00249928104897629,-0.0235973078898677,
-0.0122515009405181));
#35607=CARTESIAN_POINT('Ctrl Pts',(-0.00249703476091654,-0.023600232019034,
-0.012297580041113));
#35608=CARTESIAN_POINT('Ctrl Pts',(-0.00249478847285679,-0.0236031561482002,
-0.012343659141708));
#35609=CARTESIAN_POINT('Ctrl Pts',(-0.00249187034452298,-0.0236055330779767,
-0.0123810623250591));
#35610=CARTESIAN_POINT('Ctrl Pts',(-0.00248805263063428,-0.023608010349694,
-0.0124199723296372));
#35611=CARTESIAN_POINT('Ctrl Pts',(-0.00248041720285686,-0.0236129648931285,
-0.0124977923387934));
#35612=CARTESIAN_POINT('Ctrl Pts',(-0.00246825871826857,-0.0236183208043258,
-0.0125815028094976));
#35613=CARTESIAN_POINT('Ctrl Pts',(-0.00245213816847964,-0.02362357025559,
-0.0126626986446394));
#35614=CARTESIAN_POINT('Ctrl Pts',(-0.00243601761869071,-0.0236288197068541,
-0.0127438944797812));
#35615=CARTESIAN_POINT('Ctrl Pts',(-0.00241625300993701,-0.0236339626981851,
-0.012822672110062));
#35616=CARTESIAN_POINT('Ctrl Pts',(-0.00239260239173008,-0.0236391344875873,
-0.0129007352045886));
#35617=CARTESIAN_POINT('Ctrl Pts',(-0.00236895177352315,-0.0236443062769895,
-0.0129787982991151));
#35618=CARTESIAN_POINT('Ctrl Pts',(-0.00234133816747274,-0.0236495068644631,
-0.0130561057737264));
#35619=CARTESIAN_POINT('Ctrl Pts',(-0.00231001880530941,-0.023654703045686,
-0.0131317890161534));
#35620=CARTESIAN_POINT('Ctrl Pts',(-0.00224738008098274,-0.0236650954081317,
-0.0132831555010074));
#35621=CARTESIAN_POINT('Ctrl Pts',(-0.00216995704282236,-0.0236754701455747,
-0.0134280726485577));
#35622=CARTESIAN_POINT('Ctrl Pts',(-0.00207910465144895,-0.023685853140187,
-0.0135641341833234));
#35623=CARTESIAN_POINT('Ctrl Pts',(-0.00198825226007553,-0.0236962361347994,
-0.013700195718089));
#35624=CARTESIAN_POINT('Ctrl Pts',(-0.00188395549441474,-0.0237066273865811,
-0.0138273654487582));
#35625=CARTESIAN_POINT('Ctrl Pts',(-0.00176827181384625,-0.0237170205390933,
-0.0139431152344189));
#35626=CARTESIAN_POINT('Ctrl Pts',(-0.00153690445270928,-0.0237378068441178,
-0.0141746148057404));
#35627=CARTESIAN_POINT('Ctrl Pts',(-0.00125955589036972,-0.0237586007520643,
-0.0143600247471864));
#35628=CARTESIAN_POINT('Ctrl Pts',(-0.000957255209870739,-0.0237794072501214,
-0.0144853256209183));
#35629=CARTESIAN_POINT('Ctrl Pts',(-0.000654954529371758,-0.0238002137481785,
-0.0146106264946503));
#35630=CARTESIAN_POINT('Ctrl Pts',(-0.000327662745678227,-0.023821032836346,
-0.0146757918206047));
#35631=CARTESIAN_POINT('Ctrl Pts',(-4.69308788134662E-7,-0.02384186317877,
-0.014675853242508));
#35632=CARTESIAN_POINT('Ctrl Pts',(0.000326724128101958,-0.0238626935211941,
-0.0146759146644112));
#35633=CARTESIAN_POINT('Ctrl Pts',(0.000653877233610468,-0.0238835351178747,
-0.0146109397642855));
#35634=CARTESIAN_POINT('Ctrl Pts',(0.000956388057863023,-0.0239043883250395,
-0.0144856848567764));
#35635=CARTESIAN_POINT('Ctrl Pts',(0.00125889888211558,-0.0239252415322042,
-0.0143604299492672));
#35636=CARTESIAN_POINT('Ctrl Pts',(0.00153643866694449,-0.0239461063498532,
-0.0141749069905738));
#35637=CARTESIAN_POINT('Ctrl Pts',(0.00176760817590136,-0.0239669826889295,
-0.0139437790023297));
#35638=CARTESIAN_POINT('Ctrl Pts',(0.0021151382352358,-0.0239983672577275,
-0.0135963113634064));
#35639=CARTESIAN_POINT('Ctrl Pts',(0.00235715461429183,-0.0240297778658631,
-0.0131433768144827));
#35640=CARTESIAN_POINT('Ctrl Pts',(0.00245257461427401,-0.0240612145511598,
-0.0126604951764301));
#35641=CARTESIAN_POINT('Ctrl Pts',(0.00248409625812313,-0.0240715995438019,
-0.0125009770144219));
#35642=CARTESIAN_POINT('Ctrl Pts',(0.00250000029698955,-0.0240819873822101,
-0.012338390140462));
#35643=CARTESIAN_POINT('Ctrl Pts',(0.00249999999999583,-0.0240923780677479,
-0.0121758487185883));
#35644=CARTESIAN_POINT('',(0.00249999990985199,-0.0250924186728815,-0.012175385970229));
#35645=CARTESIAN_POINT('Ctrl Pts',(0.00249999974369977,-0.0240924495244571,
-0.0121747212525069));
#35646=CARTESIAN_POINT('Ctrl Pts',(0.00249977984012064,-0.0241233665601626,
-0.0116890831297981));
#35647=CARTESIAN_POINT('Ctrl Pts',(0.00235376883046109,-0.024154283595868,
-0.011203535107439));
#35648=CARTESIAN_POINT('Ctrl Pts',(0.00208632057554545,-0.0241852006315734,
-0.0107984403288524));
#35649=CARTESIAN_POINT('Ctrl Pts',(0.00199335298094986,-0.02419594769157,
-0.0106576254741796));
#35650=CARTESIAN_POINT('Ctrl Pts',(0.00188616035506248,-0.0242066947515666,
-0.010526385852805));
#35651=CARTESIAN_POINT('Ctrl Pts',(0.00176706770513845,-0.0242174418115632,
-0.010407387362245));
#35652=CARTESIAN_POINT('Ctrl Pts',(0.00143077553186628,-0.0242477892105408,
-0.010071361074879));
#35653=CARTESIAN_POINT('Ctrl Pts',(0.000994267223898821,-0.0242781366095183,
-0.00983300824219008));
#35654=CARTESIAN_POINT('Ctrl Pts',(0.00052806958498167,-0.0243084840084958,
-0.00973226115336212));
#35655=CARTESIAN_POINT('Ctrl Pts',(0.000354222155843106,-0.0243198007052203,
-0.00969469206050567));
#35656=CARTESIAN_POINT('Ctrl Pts',(0.000176510666734036,-0.0243311174019448,
-0.00967579345856524));
#35657=CARTESIAN_POINT('Ctrl Pts',(-8.4534646565241E-7,-0.0243424340986693,
-0.00967585342948023));
#35658=CARTESIAN_POINT('Ctrl Pts',(-0.000478210896877666,-0.0243728937434441,
-0.00967601484520181));
#35659=CARTESIAN_POINT('Ctrl Pts',(-0.000957059738941487,-0.0244033533882188,
-0.00981722155050242));
#35660=CARTESIAN_POINT('Ctrl Pts',(-0.0013588336126529,-0.0244338130329935,
-0.0100773845083475));
#35661=CARTESIAN_POINT('Ctrl Pts',(-0.00150662442522366,-0.0244450174839208,
-0.0101730843471288));
#35662=CARTESIAN_POINT('Ctrl Pts',(-0.00164412826440501,-0.024456221934848,
-0.0102843780503469));
#35663=CARTESIAN_POINT('Ctrl Pts',(-0.00176826327412012,-0.0244674263857754,
-0.0104085827941326));
#35664=CARTESIAN_POINT('Ctrl Pts',(-0.00210566471563643,-0.0244978803077024,
-0.0107461737742488));
#35665=CARTESIAN_POINT('Ctrl Pts',(-0.00234441242205592,-0.0245283342296294,
-0.0111845192387378));
#35666=CARTESIAN_POINT('Ctrl Pts',(-0.00244459956833509,-0.0245587881515564,
-0.0116524672430912));
#35667=CARTESIAN_POINT('Ctrl Pts',(-0.00248147873688702,-0.0245699983253314,
-0.0118247202113313));
#35668=CARTESIAN_POINT('Ctrl Pts',(-0.00250003919620521,-0.0245812084991065,
-0.0120007294925313));
#35669=CARTESIAN_POINT('Ctrl Pts',(-0.00249999993758005,-0.0245924186728815,
-0.0121764119454272));
#35670=CARTESIAN_POINT('Ctrl Pts',(-0.00249989328632472,-0.0246228725948085,
-0.0126536765991072));
#35671=CARTESIAN_POINT('Ctrl Pts',(-0.0023587989597219,-0.0246533265167354,
-0.0131324578205044));
#35672=CARTESIAN_POINT('Ctrl Pts',(-0.00209877251553004,-0.0246837804386625,
-0.0135342177177973));
#35673=CARTESIAN_POINT('Ctrl Pts',(-0.00200305605469169,-0.0246949906124375,
-0.0136821066588439));
#35674=CARTESIAN_POINT('Ctrl Pts',(-0.00189172719648904,-0.0247062007862125,
-0.0138197012239855));
#35675=CARTESIAN_POINT('Ctrl Pts',(-0.00176747325647235,-0.0247174109599876,
-0.0139439138872319));
#35676=CARTESIAN_POINT('Ctrl Pts',(-0.0014298575378662,-0.0247478706047623,
-0.0142814174509523));
#35677=CARTESIAN_POINT('Ctrl Pts',(-0.000991445184562082,-0.0247783302495369,
-0.0145202373086957));
#35678=CARTESIAN_POINT('Ctrl Pts',(-0.000523409044334443,-0.0248087898943116,
-0.0146204479303199));
#35679=CARTESIAN_POINT('Ctrl Pts',(-0.000351243938529629,-0.024819994345239,
-0.0146573099817553));
#35680=CARTESIAN_POINT('Ctrl Pts',(-0.000175324927440846,-0.0248311987961663,
-0.0146758723746888));
#35681=CARTESIAN_POINT('Ctrl Pts',(2.71971265063508E-7,-0.0248424032470937,
-0.0146758532717644));
#35682=CARTESIAN_POINT('Ctrl Pts',(0.000475878422558642,-0.0248727506460713,
-0.0146758015312488));
#35683=CARTESIAN_POINT('Ctrl Pts',(0.000953148934426867,-0.0249030980450488,
-0.0145357066301931));
#35684=CARTESIAN_POINT('Ctrl Pts',(0.00135401726721916,-0.0249334454440264,
-0.0142774329876573));
#35685=CARTESIAN_POINT('Ctrl Pts',(0.00150350307165344,-0.0249447621407509,
-0.0141811214557643));
#35686=CARTESIAN_POINT('Ctrl Pts',(0.00164250888723086,-0.0249560788374753,
-0.0140688911999047));
#35687=CARTESIAN_POINT('Ctrl Pts',(0.00176785790397681,-0.0249673955341998,
-0.0139435292838344));
#35688=CARTESIAN_POINT('Ctrl Pts',(0.00211030942677976,-0.0249983125699053,
-0.0136010425202822));
#35689=CARTESIAN_POINT('Ctrl Pts',(0.00235098062427899,-0.025029229605611,
-0.0131552093338355));
#35690=CARTESIAN_POINT('Ctrl Pts',(0.00244882364769221,-0.0250601466413165,
-0.0126791054524783));
#35691=CARTESIAN_POINT('Ctrl Pts',(0.00248283482692923,-0.025070893701313,
-0.0125136071483643));
#35692=CARTESIAN_POINT('Ctrl Pts',(0.00249999900623557,-0.0250816407613094,
-0.0123446805186293));
#35693=CARTESIAN_POINT('Ctrl Pts',(0.00249999999995669,-0.0250923878213059,
-0.0121758680029006));
#35694=CARTESIAN_POINT('',(0.00249999972657487,-0.0260925452264452,-0.0121764958944254));
#35695=CARTESIAN_POINT('Ctrl Pts',(0.00249999981974729,-0.0250924495244571,
-0.0121749039375575));
#35696=CARTESIAN_POINT('Ctrl Pts',(0.00249981540284905,-0.0251233724506544,
-0.0116892635544426));
#35697=CARTESIAN_POINT('Ctrl Pts',(0.00235383859928715,-0.0251542953768517,
-0.0112037029975709));
#35698=CARTESIAN_POINT('Ctrl Pts',(0.00208641781767861,-0.025185218303049,
-0.010798587629514));
#35699=CARTESIAN_POINT('Ctrl Pts',(0.00199350618779638,-0.0251959620435183,
-0.0106578359313471));
#35700=CARTESIAN_POINT('Ctrl Pts',(0.00188638296860404,-0.0252067057839877,
-0.0105266489217477));
#35701=CARTESIAN_POINT('Ctrl Pts',(0.00176736936274355,-0.0252174495244571,
-0.0104076888327712));
#35702=CARTESIAN_POINT('Ctrl Pts',(0.00143113101664912,-0.0252478028399471,
-0.0100716016830753));
#35703=CARTESIAN_POINT('Ctrl Pts',(0.000994658671625173,-0.0252781561554371,
-0.0098331736123015));
#35704=CARTESIAN_POINT('Ctrl Pts',(0.000528473902838359,-0.0253085094709272,
-0.00973234856300654));
#35705=CARTESIAN_POINT('Ctrl Pts',(0.00035471654166248,-0.0253198228221038,
-0.00969476883994628));
#35706=CARTESIAN_POINT('Ctrl Pts',(0.000177095770510817,-0.0253311361732804,
-0.00967584087809031));
#35707=CARTESIAN_POINT('Ctrl Pts',(-1.750795227525E-7,-0.0253424495244571,
-0.00967585329268867));
#35708=CARTESIAN_POINT('Ctrl Pts',(-0.000477545299838025,-0.0253729150913717,
-0.00967588672378889));
#35709=CARTESIAN_POINT('Ctrl Pts',(-0.000956435630825558,-0.0254033806582862,
-0.00981696765543438));
#35710=CARTESIAN_POINT('Ctrl Pts',(-0.00135828107907325,-0.0254338462252008,
-0.0100770268263114));
#35711=CARTESIAN_POINT('Ctrl Pts',(-0.00150602528364958,-0.0254450473249529,
-0.0101726412858295));
#35712=CARTESIAN_POINT('Ctrl Pts',(-0.00164349666043961,-0.025456248424705,
-0.0102838371082915));
#35713=CARTESIAN_POINT('Ctrl Pts',(-0.00176761700091796,-0.0254674495244571,
-0.010407936394262));
#35714=CARTESIAN_POINT('Ctrl Pts',(-0.00210514504448296,-0.02549790936102,
-0.0107454071830146));
#35715=CARTESIAN_POINT('Ctrl Pts',(-0.00234405371722318,-0.025528369197583,
-0.0111836696319958));
#35716=CARTESIAN_POINT('Ctrl Pts',(-0.00244441050475252,-0.025558829034146,
-0.0116515849542553));
#35717=CARTESIAN_POINT('Ctrl Pts',(-0.00248133392898926,-0.0255700358642497,
-0.0118237410821666));
#35718=CARTESIAN_POINT('Ctrl Pts',(-0.00249995784166091,-0.0255812426943533,
-0.0119996564809227));
#35719=CARTESIAN_POINT('Ctrl Pts',(-0.00249999992819427,-0.0255924495244571,
-0.0121752540965862));
#35720=CARTESIAN_POINT('Ctrl Pts',(-0.00250011431816146,-0.02562290936102,
-0.0126525232819346));
#35721=CARTESIAN_POINT('Ctrl Pts',(-0.00235923919965624,-0.0256533691975828,
-0.0131313733530485));
#35722=CARTESIAN_POINT('Ctrl Pts',(-0.00209939501672301,-0.0256838290341457,
-0.0135332554243782));
#35723=CARTESIAN_POINT('Ctrl Pts',(-0.00200379274369099,-0.0256950358642495,
-0.0136811164966417));
#35724=CARTESIAN_POINT('Ctrl Pts',(-0.00189258855932867,-0.0257062426943533,
-0.0138187003778426));
#35725=CARTESIAN_POINT('Ctrl Pts',(-0.00176846425227196,-0.0257174495244571,
-0.0139429226650592));
#35726=CARTESIAN_POINT('Ctrl Pts',(-0.00143103454669657,-0.0257479150913717,
-0.0142806187279443));
#35727=CARTESIAN_POINT('Ctrl Pts',(-0.000992751745445068,-0.0257783806582862,
-0.0145196850860781));
#35728=CARTESIAN_POINT('Ctrl Pts',(-0.000524767767902572,-0.0258088462252008,
-0.0146201566207968));
#35729=CARTESIAN_POINT('Ctrl Pts',(-0.000352706790683817,-0.0258200473249529,
-0.0146570964120631));
#35730=CARTESIAN_POINT('Ctrl Pts',(-0.000176885396462903,-0.025831248424705,
-0.0146757564858568));
#35731=CARTESIAN_POINT('Ctrl Pts',(-1.37345940904288E-6,-0.0258424495244571,
-0.0146758529092799));
#35732=CARTESIAN_POINT('Ctrl Pts',(0.000474237803374116,-0.0258728028399471,
-0.0146761142024249));
#35733=CARTESIAN_POINT('Ctrl Pts',(0.000951604262650088,-0.0259031561554371,
-0.0145363307230201));
#35734=CARTESIAN_POINT('Ctrl Pts',(0.00135264445426317,-0.0259335094709272,
-0.0142783168368607));
#35735=CARTESIAN_POINT('Ctrl Pts',(0.00150212099250688,-0.0259448228221038,
-0.0141821493620578));
#35736=CARTESIAN_POINT('Ctrl Pts',(0.0016411380949844,-0.0259561361732805,
-0.0140700717454712));
#35737=CARTESIAN_POINT('Ctrl Pts',(0.00176652158658883,-0.0259674495244572,
-0.0139448647291767));
#35738=CARTESIAN_POINT('Ctrl Pts',(0.00210923387375378,-0.0259983724506545,
-0.0136026348042137));
#35739=CARTESIAN_POINT('Ctrl Pts',(0.00235024223510933,-0.0260292953768519,
-0.0131569809680466));
#35740=CARTESIAN_POINT('Ctrl Pts',(0.00244844407310773,-0.0260602183030492,
-0.0126809489417202));
#35741=CARTESIAN_POINT('Ctrl Pts',(0.00248256293541502,-0.0260709620435185,
-0.0125155582373186));
#35742=CARTESIAN_POINT('Ctrl Pts',(0.00249985412379925,-0.0260817057839878,
-0.0123467299594587));
#35743=CARTESIAN_POINT('Ctrl Pts',(0.0024999990774521,-0.0260924495244571,
-0.0121780010152726));
#35744=CARTESIAN_POINT('',(0.00250030482084482,-0.0270929049799219,-0.0121755425884962));
#35745=CARTESIAN_POINT('Ctrl Pts',(0.00249999999998503,-0.0260925855360718,
-0.0121758619383234));
#35746=CARTESIAN_POINT('Ctrl Pts',(0.00250000168063414,-0.026123477185258,
-0.0116902243085716));
#35747=CARTESIAN_POINT('Ctrl Pts',(0.00235421253766726,-0.0261543704232938,
-0.0112046101782478));
#35748=CARTESIAN_POINT('Ctrl Pts',(0.00199403555690222,-0.0261960117468405,
-0.0106585198828652));
#35749=CARTESIAN_POINT('Ctrl Pts',(0.00188688869552743,-0.0262067545940619,
-0.0105272170746364));
#35750=CARTESIAN_POINT('Ctrl Pts',(0.00143168700788836,-0.0262478328793858,
-0.0100719809913161));
#35751=CARTESIAN_POINT('Ctrl Pts',(0.000995281622552827,-0.0262781746182928,
-0.00983343888535285));
#35752=CARTESIAN_POINT('Ctrl Pts',(0.000355274318464984,-0.0263198252081222,
-0.00969484091355799));
#35753=CARTESIAN_POINT('Ctrl Pts',(0.000177548413150109,-0.0263311385297115,
-0.00967586537989346));
#35754=CARTESIAN_POINT('Ctrl Pts',(-0.000477186214621105,-0.0263728930165037,
-0.0096758207626205));
#35755=CARTESIAN_POINT('Ctrl Pts',(-0.000956084164253438,-0.0264033256581309,
-0.00981682778217999));
#35756=CARTESIAN_POINT('Ctrl Pts',(-0.00150581592258683,-0.0264450043787476,
-0.0101724736200223));
#35757=CARTESIAN_POINT('Ctrl Pts',(-0.00164338878537718,-0.0264562192685052,
-0.0102837326518929));
#35758=CARTESIAN_POINT('Ctrl Pts',(-0.00210513380752868,-0.0264979387827995,
-0.0107453867082514));
#35759=CARTESIAN_POINT('Ctrl Pts',(-0.00234405249367148,-0.0265284892035263,
-0.0111836595020973));
#35760=CARTESIAN_POINT('Ctrl Pts',(-0.00248135359723824,-0.0265701233990174,
-0.0118238344146244));
#35761=CARTESIAN_POINT('Ctrl Pts',(-0.00249997733682184,-0.0265813094217105,
-0.0119998426203243));
#35762=CARTESIAN_POINT('Ctrl Pts',(-0.00250006149980523,-0.0266227971072005,
-0.012652885375613));
#35763=CARTESIAN_POINT('Ctrl Pts',(-0.00235908466725583,-0.0266529419769236,
-0.0131318040709003));
#35764=CARTESIAN_POINT('Ctrl Pts',(-0.00200345043979713,-0.0266942330651809,
-0.0136815752320274));
#35765=CARTESIAN_POINT('Ctrl Pts',(-0.00189219565810716,-0.0267053439854017,
-0.013819156319645));
#35766=CARTESIAN_POINT('Ctrl Pts',(-0.00143061510762509,-0.0267467057992126,
-0.014280867634229));
#35767=CARTESIAN_POINT('Ctrl Pts',(-0.000992428644244417,-0.0267770625758946,
-0.0145197947799587));
#35768=CARTESIAN_POINT('Ctrl Pts',(-0.000352195105386843,-0.0268186881980405,
-0.0146571913964735));
#35769=CARTESIAN_POINT('Ctrl Pts',(-0.000176051527598052,-0.0268299035408566,
-0.0146758371889194));
#35770=CARTESIAN_POINT('Ctrl Pts',(0.000475393790923074,-0.0268714776936433,
-0.0146758967939031));
#35771=CARTESIAN_POINT('Ctrl Pts',(0.000952706281399202,-0.0269018704543449,
-0.0145358883263421));
#35772=CARTESIAN_POINT('Ctrl Pts',(0.00150320018578933,-0.0269436776881657,
-0.0141813551430691));
#35773=CARTESIAN_POINT('Ctrl Pts',(0.00164228050286924,-0.0269550442330534,
-0.0140690963115757));
#35774=CARTESIAN_POINT('Ctrl Pts',(0.00211017853281865,-0.0269974831572675,
-0.0136012369892513));
#35775=CARTESIAN_POINT('Ctrl Pts',(0.002350891697643,-0.0270286110534918,
-0.0131554239049857));
#35776=CARTESIAN_POINT('Ctrl Pts',(0.0024828208666546,-0.0270706431659741,
-0.0125137508768078));
#35777=CARTESIAN_POINT('Ctrl Pts',(0.00250000040700823,-0.0270814960885248,
-0.0123447418903043));
#35778=CARTESIAN_POINT('Ctrl Pts',(0.00249999999999274,-0.0270923558261894,
-0.0121758472618626));
#35779=CARTESIAN_POINT('',(0.00214222575379317,-0.0271787743239008,-0.0108871062905246));
#35780=CARTESIAN_POINT('Ctrl Pts',(0.00249999955999433,-0.0270924495244571,
-0.0121743700373619));
#35781=CARTESIAN_POINT('Ctrl Pts',(0.0024997320825269,-0.027121224457605,
-0.0117235398244762));
#35782=CARTESIAN_POINT('Ctrl Pts',(0.00237462822344567,-0.0271499993907529,
-0.0112734183970132));
#35783=CARTESIAN_POINT('Ctrl Pts',(0.00214222575379317,-0.0271787743239008,
-0.0108871062905246));
#35784=CARTESIAN_POINT('',(0.000601546286298534,-0.0271787743898723,-0.0146024027019709));
#35785=CARTESIAN_POINT('Origin',(0.,-0.0271787743898623,-0.0121758532865581));
#35786=CARTESIAN_POINT('Ctrl Pts',(0.000601546286299188,-0.0271787743898619,
-0.0146024027019708));
#35787=CARTESIAN_POINT('Ctrl Pts',(0.000126738896001363,-0.027147632217151,
-0.0147201083709866));
#35788=CARTESIAN_POINT('Ctrl Pts',(-0.000383109998025324,-0.02711649004444,
-0.0146942108575127));
#35789=CARTESIAN_POINT('Ctrl Pts',(-0.000843239394494906,-0.0270853478717291,
-0.0145293501154431));
#35790=CARTESIAN_POINT('Ctrl Pts',(-0.0008686421319187,-0.0270836285804987,
-0.0145202485145143));
#35791=CARTESIAN_POINT('Ctrl Pts',(-0.000893894938573373,-0.0270819092892684,
-0.0145107365109282));
#35792=CARTESIAN_POINT('Ctrl Pts',(-0.000918984460815858,-0.027080189998038,
-0.0145008194284146));
#35793=CARTESIAN_POINT('Ctrl Pts',(-0.00136814286693025,-0.0270494108504236,
-0.0143232815330307));
#35794=CARTESIAN_POINT('Ctrl Pts',(-0.001764642299577,-0.0270186317028091,
-0.0140114859226347));
#35795=CARTESIAN_POINT('Ctrl Pts',(-0.00204312006724602,-0.0269878525551947,
-0.0136165685224103));
#35796=CARTESIAN_POINT('Ctrl Pts',(-0.00206196005624111,-0.0269857702388677,
-0.0135898509875188));
#35797=CARTESIAN_POINT('Ctrl Pts',(-0.00208027307942609,-0.0269836879225407,
-0.0135627678475282));
#35798=CARTESIAN_POINT('Ctrl Pts',(-0.0020980451501482,-0.0269816056062137,
-0.0135353408914812));
#35799=CARTESIAN_POINT('Ctrl Pts',(-0.00236143589829022,-0.0269507446635681,
-0.0131288600381567));
#35800=CARTESIAN_POINT('Ctrl Pts',(-0.00250323124197211,-0.0269198837209227,
-0.0126433620392557));
#35801=CARTESIAN_POINT('Ctrl Pts',(-0.00249994239890872,-0.0268890227782772,
-0.0121588826608035));
#35802=CARTESIAN_POINT('Ctrl Pts',(-0.0024997292038465,-0.0268870222569812,
-0.0121274769022309));
#35803=CARTESIAN_POINT('Ctrl Pts',(-0.00249892415377076,-0.0268850217356852,
-0.0120960794293595));
#35804=CARTESIAN_POINT('Ctrl Pts',(-0.00249752835018408,-0.0268830212143892,
-0.0120647131046851));
#35805=CARTESIAN_POINT('Ctrl Pts',(-0.00247600401678539,-0.0268521716824375,
-0.0115810209604391));
#35806=CARTESIAN_POINT('Ctrl Pts',(-0.00230970714499795,-0.0268213221504857,
-0.011103562613496));
#35807=CARTESIAN_POINT('Ctrl Pts',(-0.00202594829224241,-0.026790472618534,
-0.0107110893065395));
#35808=CARTESIAN_POINT('Ctrl Pts',(-0.00200744222498325,-0.0267884606865443,
-0.0106854931450614));
#35809=CARTESIAN_POINT('Ctrl Pts',(-0.00198845358085418,-0.0267864487545546,
-0.0106602512927708));
#35810=CARTESIAN_POINT('Ctrl Pts',(-0.00196899678345204,-0.0267844368225649,
-0.0106353820382852));
#35811=CARTESIAN_POINT('Ctrl Pts',(-0.00167066011192626,-0.0267535872906131,
-0.0102540546053463));
#35812=CARTESIAN_POINT('Ctrl Pts',(-0.00125806535609302,-0.0267227377586614,
-0.00996184533361782));
#35813=CARTESIAN_POINT('Ctrl Pts',(-0.000799163457009108,-0.0266918882267096,
-0.00980702704367298));
#35814=CARTESIAN_POINT('Ctrl Pts',(-0.000769234983140153,-0.0266898762947199,
-0.00979693016860164));
#35815=CARTESIAN_POINT('Ctrl Pts',(-0.000739119260466096,-0.0266878643627303,
-0.00978740194915553));
#35816=CARTESIAN_POINT('Ctrl Pts',(-0.000708838650548186,-0.0266858524307406,
-0.00977844890525548));
#35817=CARTESIAN_POINT('Ctrl Pts',(-0.000244365611328204,-0.0266549914880951,
-0.00964111853041157));
#35818=CARTESIAN_POINT('Ctrl Pts',(0.000261411968019987,-0.0266241305454496,
-0.00964279177763323));
#35819=CARTESIAN_POINT('Ctrl Pts',(0.000725083113859513,-0.0265932696028041,
-0.00978331185995839));
#35820=CARTESIAN_POINT('Ctrl Pts',(0.000755140005258831,-0.0265912690815081,
-0.00979242089529899));
#35821=CARTESIAN_POINT('Ctrl Pts',(0.000785021163560474,-0.0265892685602122,
-0.00980209517023468));
#35822=CARTESIAN_POINT('Ctrl Pts',(0.000814704975023284,-0.0265872680389162,
-0.00981232714884092));
#35823=CARTESIAN_POINT('Ctrl Pts',(0.00127140714391061,-0.0265564888913018,
-0.00996975190634997));
#35824=CARTESIAN_POINT('Ctrl Pts',(0.00168135077208624,-0.0265257097436874,
-0.0102636595335939));
#35825=CARTESIAN_POINT('Ctrl Pts',(0.00197705538432398,-0.026494930596073,
-0.0106457382558119));
#35826=CARTESIAN_POINT('Ctrl Pts',(0.00199706082923621,-0.026492848279746,
-0.010671587209508));
#35827=CARTESIAN_POINT('Ctrl Pts',(0.00201655600260596,-0.0264907659634189,
-0.0106978243520202));
#35828=CARTESIAN_POINT('Ctrl Pts',(0.0020355260119502,-0.0264886836470919,
-0.0107244285194158));
#35829=CARTESIAN_POINT('Ctrl Pts',(0.00231923281463639,-0.0264575414743809,
-0.0111223083060285));
#35830=CARTESIAN_POINT('Ctrl Pts',(0.00248283134186161,-0.0264263993016699,
-0.0116058591319997));
#35831=CARTESIAN_POINT('Ctrl Pts',(0.00249868673047212,-0.0263952571289589,
-0.0120948309256781));
#35832=CARTESIAN_POINT('Ctrl Pts',(0.00249956207179293,-0.0263935378377284,
-0.0121218259887593));
#35833=CARTESIAN_POINT('Ctrl Pts',(0.00249999986217964,-0.026391818546498,
-0.012148833995825));
#35834=CARTESIAN_POINT('Ctrl Pts',(0.00249999999996746,-0.0263900992552675,
-0.0121758405315141));
#35835=CARTESIAN_POINT('Origin',(0.,-0.0271787743898723,-0.0121758532865581));
#35836=CARTESIAN_POINT('',(-0.00299896195254882,-0.0191803670938455,-0.012169853924649));
#35837=CARTESIAN_POINT('',(0.00299896819192659,-0.019680486974571,-0.0121759389411417));
#35838=CARTESIAN_POINT('Ctrl Pts',(-0.00299896195254882,-0.0191803670938455,
-0.012169853924649));
#35839=CARTESIAN_POINT('Ctrl Pts',(-0.00299880224766938,-0.0191818636123297,
-0.0121992568003792));
#35840=CARTESIAN_POINT('Ctrl Pts',(-0.00299852404358193,-0.0191833290209218,
-0.0122250123092027));
#35841=CARTESIAN_POINT('Ctrl Pts',(-0.00299800114766971,-0.0191846148334388,
-0.0122482025519681));
#35842=CARTESIAN_POINT('Ctrl Pts',(-0.00299740209262557,-0.0191860879229316,
-0.0122747704244237));
#35843=CARTESIAN_POINT('Ctrl Pts',(-0.00299648390590115,-0.0191873213968317,
-0.0122979737332858));
#35844=CARTESIAN_POINT('Ctrl Pts',(-0.00299528035553771,-0.0191885761336485,
-0.0123217600538735));
#35845=CARTESIAN_POINT('Ctrl Pts',(-0.00299287325481085,-0.0191910856072822,
-0.0123693326950491));
#35846=CARTESIAN_POINT('Ctrl Pts',(-0.0029892837839955,-0.0191937517300053,
-0.0124192300566519));
#35847=CARTESIAN_POINT('Ctrl Pts',(-0.00298449948012424,-0.0191963745757028,
-0.0124685748257699));
#35848=CARTESIAN_POINT('Ctrl Pts',(-0.0029749308723817,-0.0192016202670976,
-0.0125672643640059));
#35849=CARTESIAN_POINT('Ctrl Pts',(-0.00296064216996607,-0.0192065882359609,
-0.0126637584356527));
#35850=CARTESIAN_POINT('Ctrl Pts',(-0.00294167528334986,-0.0192114919847212,
-0.01275981020314));
#35851=CARTESIAN_POINT('Ctrl Pts',(-0.00292270839673364,-0.0192163957334815,
-0.0128558619706273));
#35852=CARTESIAN_POINT('Ctrl Pts',(-0.00289904298078549,-0.0192212721522644,
-0.0129514639649636));
#35853=CARTESIAN_POINT('Ctrl Pts',(-0.00287077868553411,-0.0192260969694797,
-0.0130455753309895));
#35854=CARTESIAN_POINT('Ctrl Pts',(-0.00284251439028272,-0.019230921786695,
-0.0131396866970154));
#35855=CARTESIAN_POINT('Ctrl Pts',(-0.00280965551856699,-0.0192356858357989,
-0.0132323106181608));
#35856=CARTESIAN_POINT('Ctrl Pts',(-0.0027723055452403,-0.0192404774689402,
-0.013323121329571));
#35857=CARTESIAN_POINT('Ctrl Pts',(-0.00270257498363687,-0.0192494232121411,
-0.0134926604575071));
#35858=CARTESIAN_POINT('Ctrl Pts',(-0.00261717238342509,-0.019258491751231,
-0.0136559066227712));
#35859=CARTESIAN_POINT('Ctrl Pts',(-0.00251731130281746,-0.0192682599616135,
-0.0138097133907207));
#35860=CARTESIAN_POINT('Ctrl Pts',(-0.00251019465052561,-0.0192689560982503,
-0.0138206745107183));
#35861=CARTESIAN_POINT('Ctrl Pts',(-0.00250300455829962,-0.0192696557883602,
-0.0138315880401406));
#35862=CARTESIAN_POINT('Ctrl Pts',(-0.00249574239501426,-0.0192703592407384,
-0.013842453612651));
#35863=CARTESIAN_POINT('Ctrl Pts',(-0.00238657733645111,-0.0192809335582027,
-0.0140057852278754));
#35864=CARTESIAN_POINT('Ctrl Pts',(-0.00226104203758436,-0.0192922469269428,
-0.0141580541481476));
#35865=CARTESIAN_POINT('Ctrl Pts',(-0.00212187971374463,-0.0193034712736315,
-0.0142965100605622));
#35866=CARTESIAN_POINT('Ctrl Pts',(-0.00184355506606512,-0.0193259199670087,
-0.0145734218853915));
#35867=CARTESIAN_POINT('Ctrl Pts',(-0.00151080520325619,-0.0193478617734335,
-0.0147952418066359));
#35868=CARTESIAN_POINT('Ctrl Pts',(-0.00114835782098663,-0.0193677192990411,
-0.0149461198238439));
#35869=CARTESIAN_POINT('Ctrl Pts',(-0.000790043872778773,-0.0193873503648183,
-0.0150952771931288));
#35870=CARTESIAN_POINT('Ctrl Pts',(-0.000402166286245195,-0.0194051547993873,
-0.0151750374146334));
#35871=CARTESIAN_POINT('Ctrl Pts',(-1.39131433410026E-5,-0.0194258308536781,
-0.0151767688928234));
#35872=CARTESIAN_POINT('Ctrl Pts',(-9.43433704985339E-6,-0.0194260693682754,
-0.0151767888667902));
#35873=CARTESIAN_POINT('Ctrl Pts',(-4.95535653832698E-6,-0.0194263082650118,
-0.0151767984904286));
#35874=CARTESIAN_POINT('Ctrl Pts',(-4.76237866949609E-7,-0.0194265475510998,
-0.0151767977970567));
#35875=CARTESIAN_POINT('Ctrl Pts',(0.000392283102934089,-0.0194475297694933,
-0.0151767369975265));
#35876=CARTESIAN_POINT('Ctrl Pts',(0.000784350710633772,-0.0194711918902264,
-0.0150970096259685));
#35877=CARTESIAN_POINT('Ctrl Pts',(0.00114706628041126,-0.0194929067069842,
-0.014946525686211));
#35878=CARTESIAN_POINT('Ctrl Pts',(0.00150978185018874,-0.019514621523742,
-0.0147960417464534));
#35879=CARTESIAN_POINT('Ctrl Pts',(0.00184354545898445,-0.0195344202044027,
-0.014574687276006));
#35880=CARTESIAN_POINT('Ctrl Pts',(0.00212119098327946,-0.0195531656601654,
-0.0142974175110577));
#35881=CARTESIAN_POINT('Ctrl Pts',(0.00226334811709381,-0.0195627635107702,
-0.014155452769582));
#35882=CARTESIAN_POINT('Ctrl Pts',(0.00239186651239939,-0.0195731695487958,
-0.0140003848492412));
#35883=CARTESIAN_POINT('Ctrl Pts',(0.00250275064154011,-0.0195840122226612,
-0.0138334451870744));
#35884=CARTESIAN_POINT('Ctrl Pts',(0.00282499616095954,-0.0196155226209365,
-0.013348294078764));
#35885=CARTESIAN_POINT('Ctrl Pts',(0.00299816054098966,-0.0196507207089565,
-0.0127602146141065));
#35886=CARTESIAN_POINT('Ctrl Pts',(0.00299896819192659,-0.019680486974571,
-0.0121759389411417));
#35887=CARTESIAN_POINT('',(0.00299999984374834,-0.0246800791551026,-0.0121768215375359));
#35888=CARTESIAN_POINT('Ctrl Pts',(0.00299999999774018,-0.0196810819667495,
-0.0121759697293255));
#35889=CARTESIAN_POINT('Ctrl Pts',(0.00300000942085986,-0.0196932559099264,
-0.0119331950198641));
#35890=CARTESIAN_POINT('Ctrl Pts',(0.00297055154201463,-0.0197045033254348,
-0.0116913234487237));
#35891=CARTESIAN_POINT('Ctrl Pts',(0.00288497146224982,-0.0197215353186389,
-0.0113452722338703));
#35892=CARTESIAN_POINT('Ctrl Pts',(0.00285142836003338,-0.0197270473697668,
-0.0112365570788726));
#35893=CARTESIAN_POINT('Ctrl Pts',(0.00280154164464815,-0.0197343362154213,
-0.0111024332638439));
#35894=CARTESIAN_POINT('Ctrl Pts',(0.00279087696749342,-0.0197358535763954,
-0.0110750028145183));
#35895=CARTESIAN_POINT('Ctrl Pts',(0.00277416703216802,-0.0197381779544933,
-0.0110338276581702));
#35896=CARTESIAN_POINT('Ctrl Pts',(0.00276841903686469,-0.0197389686957665,
-0.0110199634666039));
#35897=CARTESIAN_POINT('Ctrl Pts',(0.00275771198906117,-0.0197404268147673,
-0.0109946760528532));
#35898=CARTESIAN_POINT('Ctrl Pts',(0.00275278551259007,-0.0197410923173646,
-0.010983239779294));
#35899=CARTESIAN_POINT('Ctrl Pts',(0.00274132094684287,-0.0197426287040395,
-0.0109570755732567));
#35900=CARTESIAN_POINT('Ctrl Pts',(0.00273473526014656,-0.0197435023038016,
-0.0109423693256647));
#35901=CARTESIAN_POINT('Ctrl Pts',(0.0027129404632505,-0.0197463630938318,
-0.0108947327789585));
#35902=CARTESIAN_POINT('Ctrl Pts',(0.00269725301474739,-0.0197483757861134,
-0.0108620261826589));
#35903=CARTESIAN_POINT('Ctrl Pts',(0.0025954709778507,-0.019761118544118,
-0.0106593317430168));
#35904=CARTESIAN_POINT('Ctrl Pts',(0.00249394052655557,-0.019772456052928,
-0.0104975916122593));
#35905=CARTESIAN_POINT('Ctrl Pts',(0.00228706715201482,-0.0197923412922303,
-0.0102286892166359));
#35906=CARTESIAN_POINT('Ctrl Pts',(0.00218772104820752,-0.019800934113632,
-0.0101176965903746));
#35907=CARTESIAN_POINT('Ctrl Pts',(0.00204046551884058,-0.0198123102878746,
-0.00997594539406847));
#35908=CARTESIAN_POINT('Ctrl Pts',(0.00199932318697792,-0.0198153622794282,
-0.00993848840368143));
#35909=CARTESIAN_POINT('Ctrl Pts',(0.00193639885452232,-0.0198198473456321,
-0.00988432323864402));
#35910=CARTESIAN_POINT('Ctrl Pts',(0.00191539231956945,-0.0198213157146306,
-0.00986673596299922));
#35911=CARTESIAN_POINT('Ctrl Pts',(0.00187704472145465,-0.0198239454088719,
-0.0098355136715209));
#35912=CARTESIAN_POINT('Ctrl Pts',(0.0018597887736179,-0.0198251107002371,
-0.00982177763943566));
#35913=CARTESIAN_POINT('Ctrl Pts',(0.001822282715594,-0.0198276056542681,
-0.00979259200263082));
#35914=CARTESIAN_POINT('Ctrl Pts',(0.00180198408116384,-0.0198289327384977,
-0.00977720740474276));
#35915=CARTESIAN_POINT('Ctrl Pts',(0.00174571834056147,-0.0198325499745693,
-0.00973568028140222));
#35916=CARTESIAN_POINT('Ctrl Pts',(0.00170936151388481,-0.0198348198162695,
-0.00971007545957484));
#35917=CARTESIAN_POINT('Ctrl Pts',(0.00149261545771245,-0.0198479892643146,
-0.00956452763602865));
#35918=CARTESIAN_POINT('Ctrl Pts',(0.00130023521666765,-0.0198581755577152,
-0.00946359988869757));
#35919=CARTESIAN_POINT('Ctrl Pts',(0.000996835947108489,-0.0198736423375735,
-0.00934419474795427));
#35920=CARTESIAN_POINT('Ctrl Pts',(0.000892909671420817,-0.0198788562507925,
-0.00930972665712547));
#35921=CARTESIAN_POINT('Ctrl Pts',(0.000730074500464841,-0.0198871927288724,
-0.00926543870069178));
#35922=CARTESIAN_POINT('Ctrl Pts',(0.000672363449334335,-0.0198901792665594,
-0.0092515673234337));
#35923=CARTESIAN_POINT('Ctrl Pts',(0.000595150796872156,-0.0198942613762364,
-0.00923541495603533));
#35924=CARTESIAN_POINT('Ctrl Pts',(0.000575980754474471,-0.0198952818794518,
-0.0092315998704853));
#35925=CARTESIAN_POINT('Ctrl Pts',(0.000544069140181193,-0.0198969943083237,
-0.00922557262594156));
#35926=CARTESIAN_POINT('Ctrl Pts',(0.000531347732794319,-0.0198976805498759,
-0.00922325497541845));
#35927=CARTESIAN_POINT('Ctrl Pts',(0.000506939874544787,-0.0198990047216707,
-0.0092189710781141));
#35928=CARTESIAN_POINT('Ctrl Pts',(0.000495256090501816,-0.0198996418414808,
-0.00921699171050771));
#35929=CARTESIAN_POINT('Ctrl Pts',(0.00046321519864308,-0.0199013973612555,
-0.00921175870693947));
#35930=CARTESIAN_POINT('Ctrl Pts',(0.000442836148301305,-0.0199025231115508,
-0.00920864566046527));
#35931=CARTESIAN_POINT('Ctrl Pts',(0.000359542717456324,-0.019907157220927,
-0.0091967991606986));
#35932=CARTESIAN_POINT('Ctrl Pts',(0.000296393888987575,-0.019910746820327,
-0.0091898552821384));
#35933=CARTESIAN_POINT('Ctrl Pts',(6.65736953401946E-5,-0.0199239765889576,
-0.00917194590946633));
#35934=CARTESIAN_POINT('Ctrl Pts',(-0.00010071849450859,-0.0199339043657393,
-0.00917289703441693));
#35935=CARTESIAN_POINT('Ctrl Pts',(-0.000376889693571773,-0.0199501171452961,
-0.00919757977549564));
#35936=CARTESIAN_POINT('Ctrl Pts',(-0.000486101343359905,-0.0199564864687802,
-0.00921344419637997));
#35937=CARTESIAN_POINT('Ctrl Pts',(-0.000665312466432556,-0.0199667846106084,
-0.0092496572911397));
#35938=CARTESIAN_POINT('Ctrl Pts',(-0.000735885303288047,-0.0199708006126325,
-0.00926660291706258));
#35939=CARTESIAN_POINT('Ctrl Pts',(-0.000834885786172269,-0.0199763769904146,
-0.00929420812692323));
#35940=CARTESIAN_POINT('Ctrl Pts',(-0.000863869378479237,-0.019978002586475,
-0.00930276385362857));
#35941=CARTESIAN_POINT('Ctrl Pts',(-0.00091409052330962,-0.0199808080416776,
-0.00931841744172763));
#35942=CARTESIAN_POINT('Ctrl Pts',(-0.000935386692247302,-0.0199819941215276,
-0.00932531774659095));
#35943=CARTESIAN_POINT('Ctrl Pts',(-0.000979314076889665,-0.0199844338868793,
-0.00934009623424393));
#35944=CARTESIAN_POINT('Ctrl Pts',(-0.00100193218597993,-0.0199856863665396,
-0.00934800851370281));
#35945=CARTESIAN_POINT('Ctrl Pts',(-0.0010605615242782,-0.0199889245151301,
-0.00936931001272005));
#35946=CARTESIAN_POINT('Ctrl Pts',(-0.00109641516670566,-0.0199908963149319,
-0.00938312167629061));
#35947=CARTESIAN_POINT('Ctrl Pts',(-0.0012831739973483,-0.0200011374855641,
-0.00945921676269332));
#35948=CARTESIAN_POINT('Ctrl Pts',(-0.00142908240008463,-0.0200090154656167,
-0.00953305550697632));
#35949=CARTESIAN_POINT('Ctrl Pts',(-0.00170369694802678,-0.0200243327118081,
-0.00970145330428935));
#35950=CARTESIAN_POINT('Ctrl Pts',(-0.00183231026747759,-0.0200317587103755,
-0.00979512378401006));
#35951=CARTESIAN_POINT('Ctrl Pts',(-0.00199021555579363,-0.0200419362372399,
-0.00993053393145888));
#35952=CARTESIAN_POINT('Ctrl Pts',(-0.00202674145422159,-0.0200443743030958,
-0.00996344834147788));
#35953=CARTESIAN_POINT('Ctrl Pts',(-0.00208764533376151,-0.0200486174838141,
-0.0100211046748876));
#35954=CARTESIAN_POINT('Ctrl Pts',(-0.00211243314293161,-0.0200503976619801,
-0.0100454001323372));
#35955=CARTESIAN_POINT('Ctrl Pts',(-0.00214802909963873,-0.0200530429173887,
-0.0100815211149638));
#35956=CARTESIAN_POINT('Ctrl Pts',(-0.00215917365006069,-0.0200538842751676,
-0.0100930125858848));
#35957=CARTESIAN_POINT('Ctrl Pts',(-0.00217880792384195,-0.0200553913300773,
-0.0101135849830775));
#35958=CARTESIAN_POINT('Ctrl Pts',(-0.00218733395524536,-0.0200560542955639,
-0.0101226302875094));
#35959=CARTESIAN_POINT('Ctrl Pts',(-0.00220623921133514,-0.0200575436798906,
-0.0101429383593398));
#35960=CARTESIAN_POINT('Ctrl Pts',(-0.00221658846832652,-0.0200583721440548,
-0.0101542276780704));
#35961=CARTESIAN_POINT('Ctrl Pts',(-0.00224762053487566,-0.0200608949479944,
-0.0101886032574669));
#35962=CARTESIAN_POINT('Ctrl Pts',(-0.00226803186464373,-0.0200626071380429,
-0.0102119306656247));
#35963=CARTESIAN_POINT('Ctrl Pts',(-0.00237867623234598,-0.0200721648017542,
-0.0103424078821197));
#35964=CARTESIAN_POINT('Ctrl Pts',(-0.0024616746123822,-0.0200803677998503,
-0.0104554535792134));
#35965=CARTESIAN_POINT('Ctrl Pts',(-0.00260416314206305,-0.0200960553509669,
-0.0106810602528687));
#35966=CARTESIAN_POINT('Ctrl Pts',(-0.00266500079234953,-0.0201035189721637,
-0.0107924352771941));
#35967=CARTESIAN_POINT('Ctrl Pts',(-0.00275158144974282,-0.0201153152728251,
-0.0109779887758199));
#35968=CARTESIAN_POINT('Ctrl Pts',(-0.00278178615861875,-0.0201197444727173,
-0.0110499105920363));
#35969=CARTESIAN_POINT('Ctrl Pts',(-0.00282921700862539,-0.0201272750004197,
-0.0111764543467603));
#35970=CARTESIAN_POINT('Ctrl Pts',(-0.00284774534043282,-0.0201304138390153,
-0.0112305415912974));
#35971=CARTESIAN_POINT('Ctrl Pts',(-0.00287293470464104,-0.0201349989912632,
-0.0113115546823074));
#35972=CARTESIAN_POINT('Ctrl Pts',(-0.00288078569278209,-0.0201364829528375,
-0.0113380945167813));
#35973=CARTESIAN_POINT('Ctrl Pts',(-0.00289418241640879,-0.0201391187464281,
-0.0113857984891497));
#35974=CARTESIAN_POINT('Ctrl Pts',(-0.00289986594512205,-0.0201402749035637,
-0.0114069215752569));
#35975=CARTESIAN_POINT('Ctrl Pts',(-0.00291159796098504,-0.0201427470703293,
-0.0114525054334494));
#35976=CARTESIAN_POINT('Ctrl Pts',(-0.00291757035792206,-0.0201440605934702,
-0.0114769841571138));
#35977=CARTESIAN_POINT('Ctrl Pts',(-0.00293294300647906,-0.0201476003020756,
-0.0115436261188216));
#35978=CARTESIAN_POINT('Ctrl Pts',(-0.00294174230999734,-0.0201498076448016,
-0.0115859225366728));
#35979=CARTESIAN_POINT('Ctrl Pts',(-0.00299131615892334,-0.0201635277426357,
-0.0118530195192053));
#35980=CARTESIAN_POINT('Ctrl Pts',(-0.00300721299564807,-0.0201742288384246,
-0.0120816661477068));
#35981=CARTESIAN_POINT('Ctrl Pts',(-0.00299241555553404,-0.0201899561963817,
-0.0124124718653403));
#35982=CARTESIAN_POINT('Ctrl Pts',(-0.00298256687078906,-0.0201948644538741,
-0.0125147218640876));
#35983=CARTESIAN_POINT('Ctrl Pts',(-0.00295911256298726,-0.0202027714239048,
-0.0126727590124251));
#35984=CARTESIAN_POINT('Ctrl Pts',(-0.00294911614480763,-0.0202056502094231,
-0.0127290039632965));
#35985=CARTESIAN_POINT('Ctrl Pts',(-0.00293360498392159,-0.0202096058214925,
-0.012803813373982));
#35986=CARTESIAN_POINT('Ctrl Pts',(-0.0029295068379246,-0.0202106133370104,
-0.0128226621625127));
#35987=CARTESIAN_POINT('Ctrl Pts',(-0.00292236951597387,-0.0202123100750276,
-0.0128540290138118));
#35988=CARTESIAN_POINT('Ctrl Pts',(-0.00291943088581132,-0.020212993836971,
-0.0128665697285904));
#35989=CARTESIAN_POINT('Ctrl Pts',(-0.00291322411689053,-0.0202144090540339,
-0.0128923099448489));
#35990=CARTESIAN_POINT('Ctrl Pts',(-0.00290994686141008,-0.0202151409576377,
-0.0129055067301678));
#35991=CARTESIAN_POINT('Ctrl Pts',(-0.00290096427991589,-0.0202171063427593,
-0.012940654327349));
#35992=CARTESIAN_POINT('Ctrl Pts',(-0.00289509965088559,-0.0202183482269523,
-0.0129625631033061));
#35993=CARTESIAN_POINT('Ctrl Pts',(-0.00286538194683253,-0.0202244419059285,
-0.0130687459525988));
#35994=CARTESIAN_POINT('Ctrl Pts',(-0.00283809595356002,-0.0202294493686955,
-0.0131520090316973));
#35995=CARTESIAN_POINT('Ctrl Pts',(-0.00273316094970527,-0.0202467199716527,
-0.0134304088053662));
#35996=CARTESIAN_POINT('Ctrl Pts',(-0.00263868528334712,-0.0202592514776756,
-0.0136185691746219));
#35997=CARTESIAN_POINT('Ctrl Pts',(-0.00248801231823542,-0.0202752362849872,
-0.0138535228774343));
#35998=CARTESIAN_POINT('Ctrl Pts',(-0.00244868556063563,-0.0202791419270268,
-0.0139104196688076));
#35999=CARTESIAN_POINT('Ctrl Pts',(-0.0023761801214289,-0.0202858874761807,
-0.0140079313815856));
#36000=CARTESIAN_POINT('Ctrl Pts',(-0.00234383847415808,-0.0202887549861224,
-0.0140491295043748));
#36001=CARTESIAN_POINT('Ctrl Pts',(-0.00229334912919302,-0.0202930262566952,
-0.014110088826567));
#36002=CARTESIAN_POINT('Ctrl Pts',(-0.00227598896752729,-0.0202944605377628,
-0.0141304866627678));
#36003=CARTESIAN_POINT('Ctrl Pts',(-0.00224527058404976,-0.0202969402845401,
-0.0141656159004601));
#36004=CARTESIAN_POINT('Ctrl Pts',(-0.00223203493829109,-0.0202979906240181,
-0.0141804518286653));
#36005=CARTESIAN_POINT('Ctrl Pts',(-0.00220173096618436,-0.0203003554421572,
-0.0142137474843456));
#36006=CARTESIAN_POINT('Ctrl Pts',(-0.00218457600651364,-0.0203016662110502,
-0.0142321265492309));
#36007=CARTESIAN_POINT('Ctrl Pts',(-0.00213749974708217,-0.0203051902298643,
-0.0142813077883869));
#36008=CARTESIAN_POINT('Ctrl Pts',(-0.00210714436952688,-0.0203073849279842,
-0.0143116872377933));
#36009=CARTESIAN_POINT('Ctrl Pts',(-0.00188553440550454,-0.0203228940255787,
-0.0145241479132106));
#36010=CARTESIAN_POINT('Ctrl Pts',(-0.00167164363907698,-0.0203350745480223,
-0.0146809153804785));
#36011=CARTESIAN_POINT('Ctrl Pts',(-0.00134576887739119,-0.0203528626470813,
-0.0148592171273823));
#36012=CARTESIAN_POINT('Ctrl Pts',(-0.00124885408079294,-0.0203580880841256,
-0.0149056692558978));
#36013=CARTESIAN_POINT('Ctrl Pts',(-0.00112316556939509,-0.0203650261742712,
-0.0149578170334922));
#36014=CARTESIAN_POINT('Ctrl Pts',(-0.00109650929841579,-0.0203665066015079,
-0.0149684310258501));
#36015=CARTESIAN_POINT('Ctrl Pts',(-0.00105582192866817,-0.0203687856210796,
-0.0149839595694495));
#36016=CARTESIAN_POINT('Ctrl Pts',(-0.00104189911941838,-0.0203695688786154,
-0.0149891550918779));
#36017=CARTESIAN_POINT('Ctrl Pts',(-0.00101622404757766,-0.0203710204979734,
-0.0149985194322769));
#36018=CARTESIAN_POINT('Ctrl Pts',(-0.00100448361276045,-0.0203716871161402,
-0.015002718713082));
#36019=CARTESIAN_POINT('Ctrl Pts',(-0.000977325480671667,-0.020373235510257,
-0.0150122420022128));
#36020=CARTESIAN_POINT('Ctrl Pts',(-0.000961890172656447,-0.0203741201632206,
-0.0150175135958196));
#36021=CARTESIAN_POINT('Ctrl Pts',(-0.00091089574395287,-0.0203770562240958,
-0.0150344665585622));
#36022=CARTESIAN_POINT('Ctrl Pts',(-0.000875162161939421,-0.0203791349404358,
-0.015045607951547));
#36023=CARTESIAN_POINT('Ctrl Pts',(-0.000657360091845289,-0.0203918946501266,
-0.0151090704720735));
#36024=CARTESIAN_POINT('Ctrl Pts',(-0.000470887041336941,-0.0204031659265746,
-0.0151447159342289));
#36025=CARTESIAN_POINT('Ctrl Pts',(-0.000134905140236743,-0.0204229443996268,
-0.0151764735785013));
#36026=CARTESIAN_POINT('Ctrl Pts',(1.33388720978418E-5,-0.0204314966286613,
-0.0151794763981626));
#36027=CARTESIAN_POINT('Ctrl Pts',(0.000216824902070318,-0.0204428391592764,
-0.0151685257942992));
#36028=CARTESIAN_POINT('Ctrl Pts',(0.00027234617117966,-0.020445894970584,
-0.0151639847926802));
#36029=CARTESIAN_POINT('Ctrl Pts',(0.000354954855349634,-0.0204503844475721,
-0.0151549065282144));
#36030=CARTESIAN_POINT('Ctrl Pts',(0.000382156524678651,-0.0204518535096552,
-0.0151515393627822));
#36031=CARTESIAN_POINT('Ctrl Pts',(0.000431157947552576,-0.0204544839487054,
-0.0151447906826176));
#36032=CARTESIAN_POINT('Ctrl Pts',(0.000452973558752462,-0.020455649301627,
-0.0151415406313959));
#36033=CARTESIAN_POINT('Ctrl Pts',(0.000499890259380584,-0.0204581438554286,
-0.0151340212848174));
#36034=CARTESIAN_POINT('Ctrl Pts',(0.000524976948216953,-0.020459470485612,
-0.0151296724132539));
#36035=CARTESIAN_POINT('Ctrl Pts',(0.000593671700948981,-0.0204630851143049,
-0.015116861097396));
#36036=CARTESIAN_POINT('Ctrl Pts',(0.000637152696479634,-0.0204653528529032,
-0.0151077485319775));
#36037=CARTESIAN_POINT('Ctrl Pts',(0.000891826619596656,-0.0204785434197699,
-0.0150484415238024));
#36038=CARTESIAN_POINT('Ctrl Pts',(0.00109726742167923,-0.0204887493580625,
-0.0149764120974078));
#36039=CARTESIAN_POINT('Ctrl Pts',(0.00139163601876189,-0.0205042254131153,
-0.0148357898537147));
#36040=CARTESIAN_POINT('Ctrl Pts',(0.00148747776550082,-0.0205094272115502,
-0.0147834040169232));
#36041=CARTESIAN_POINT('Ctrl Pts',(0.00163061781184453,-0.0205177467488282,
-0.014694701664933));
#36042=CARTESIAN_POINT('Ctrl Pts',(0.00168005016802281,-0.02052072911589,
-0.0146620033628829));
#36043=CARTESIAN_POINT('Ctrl Pts',(0.00174444656171948,-0.0205248063359435,
-0.0146166088785961));
#36044=CARTESIAN_POINT('Ctrl Pts',(0.00176030356309906,-0.0205258263477646,
-0.0146051974353997));
#36045=CARTESIAN_POINT('Ctrl Pts',(0.00178646731883081,-0.0205275381833709,
-0.014585978112248));
#36046=CARTESIAN_POINT('Ctrl Pts',(0.00179683736896153,-0.0205282243315903,
-0.0145782567956686));
#36047=CARTESIAN_POINT('Ctrl Pts',(0.00181661783993641,-0.0205295485289889,
-0.0145633289629271));
#36048=CARTESIAN_POINT('Ctrl Pts',(0.0018260360061562,-0.0205301857701985,
-0.0145561333071093));
#36049=CARTESIAN_POINT('Ctrl Pts',(0.00185172684373345,-0.0205319420189543,
-0.0145362628159982));
#36050=CARTESIAN_POINT('Ctrl Pts',(0.00186791154304711,-0.020533068386712,
-0.0145234758863733));
#36051=CARTESIAN_POINT('Ctrl Pts',(0.00193347393326414,-0.0205377088933039,
-0.0144705702996683));
#36052=CARTESIAN_POINT('Ctrl Pts',(0.00198169872866843,-0.0205413045442231,
-0.0144290547277521));
#36053=CARTESIAN_POINT('Ctrl Pts',(0.0021515462439045,-0.0205545365781522,
-0.0142731645081597));
#36054=CARTESIAN_POINT('Ctrl Pts',(0.00226489024162764,-0.0205644596693824,
-0.014150223232666));
#36055=CARTESIAN_POINT('Ctrl Pts',(0.00243512801042965,-0.0205806659576667,
-0.0139315023930857));
#36056=CARTESIAN_POINT('Ctrl Pts',(0.00249799485177614,-0.0205870334287672,
-0.0138408389070902));
#36057=CARTESIAN_POINT('Ctrl Pts',(0.00259371944215801,-0.020597329027143,
-0.013685118419402));
#36058=CARTESIAN_POINT('Ctrl Pts',(0.00262945491167657,-0.0206013442807375,
-0.013621961810522));
#36059=CARTESIAN_POINT('Ctrl Pts',(0.00267678423629044,-0.0206069198293628,
-0.0135307477982825));
#36060=CARTESIAN_POINT('Ctrl Pts',(0.0026902950449282,-0.0206085453180598,
-0.0135037183578124));
#36061=CARTESIAN_POINT('Ctrl Pts',(0.00271310037616789,-0.0206113506516388,
-0.0134563170420844));
#36062=CARTESIAN_POINT('Ctrl Pts',(0.00272257930431704,-0.020612536715622,
-0.013436037022608));
#36063=CARTESIAN_POINT('Ctrl Pts',(0.00274173307154,-0.0206149765057216,
-0.0133938327297171));
#36064=CARTESIAN_POINT('Ctrl Pts',(0.00275137401338352,-0.0206162290252235,
-0.0133718947748602));
#36065=CARTESIAN_POINT('Ctrl Pts',(0.00277578660096375,-0.0206194674023976,
-0.0133144862066364));
#36066=CARTESIAN_POINT('Ctrl Pts',(0.00279014171648493,-0.0206214393872089,
-0.0132788426576845));
#36067=CARTESIAN_POINT('Ctrl Pts',(0.00286190338657024,-0.0206316848528137,
-0.0130902849029507));
#36068=CARTESIAN_POINT('Ctrl Pts',(0.0029074389690806,-0.0206395665137156,
-0.0129331391784095));
#36069=CARTESIAN_POINT('Ctrl Pts',(0.00297156808176349,-0.02065488406393,
-0.0126174405475281));
#36070=CARTESIAN_POINT('Ctrl Pts',(0.00299077219366521,-0.0206623069356738,
-0.0124595664868214));
#36071=CARTESIAN_POINT('Ctrl Pts',(0.00299944094061995,-0.0206724806131768,
-0.0122518137264891));
#36072=CARTESIAN_POINT('Ctrl Pts',(0.00300028278161035,-0.0206749181885004,
-0.0122026632409654));
#36073=CARTESIAN_POINT('Ctrl Pts',(0.00299965846296588,-0.0206791606015538,
-0.0121188151077759));
#36074=CARTESIAN_POINT('Ctrl Pts',(0.00299879800491358,-0.0206809405146866,
-0.0120841222628853));
#36075=CARTESIAN_POINT('Ctrl Pts',(0.00299666157164527,-0.0206835854488807,
-0.0120334606865239));
#36076=CARTESIAN_POINT('Ctrl Pts',(0.00299585916587873,-0.0206844267587009,
-0.0120174737949181));
#36077=CARTESIAN_POINT('Ctrl Pts',(0.00299420640871956,-0.0206859337642829,
-0.0119890846979385));
#36078=CARTESIAN_POINT('Ctrl Pts',(0.00299340685696831,-0.0206865967291995,
-0.0119766802376367));
#36079=CARTESIAN_POINT('Ctrl Pts',(0.00299145005531643,-0.0206880861586951,
-0.011949002783292));
#36080=CARTESIAN_POINT('Ctrl Pts',(0.00299025293570462,-0.0206889146693103,
-0.0119337335957787));
#36081=CARTESIAN_POINT('Ctrl Pts',(0.00298627937454701,-0.0206914377598778,
-0.0118875886297702));
#36082=CARTESIAN_POINT('Ctrl Pts',(0.00298314129640574,-0.0206931501958046,
-0.0118567469187812));
#36083=CARTESIAN_POINT('Ctrl Pts',(0.0029631186028233,-0.0207027414972802,
-0.0116862428268249));
#36084=CARTESIAN_POINT('Ctrl Pts',(0.00293690505829126,-0.0207109809644874,
-0.0115478618239667));
#36085=CARTESIAN_POINT('Ctrl Pts',(0.00286849300119061,-0.0207267744796425,
-0.0112880893931355));
#36086=CARTESIAN_POINT('Ctrl Pts',(0.00282801573819313,-0.0207343075714324,
-0.0111665432863211));
#36087=CARTESIAN_POINT('Ctrl Pts',(0.00275095547654377,-0.0207461083871148,
-0.0109766159551572));
#36088=CARTESIAN_POINT('Ctrl Pts',(0.00271927640245593,-0.0207504786362945,
-0.0109064190280484));
#36089=CARTESIAN_POINT('Ctrl Pts',(0.00265966502553371,-0.0207579216449709,
-0.0107868286874288));
#36090=CARTESIAN_POINT('Ctrl Pts',(0.00263296872806532,-0.0207610307250221,
-0.0107368662649599));
#36091=CARTESIAN_POINT('Ctrl Pts',(0.00259119171484513,-0.0207655816225221,
-0.0106637401541188));
#36092=CARTESIAN_POINT('Ctrl Pts',(0.0025771808929533,-0.0207670602738008,
-0.010639982412334));
#36093=CARTESIAN_POINT('Ctrl Pts',(0.00255137322697377,-0.0207697010359709,
-0.0105975688924264));
#36094=CARTESIAN_POINT('Ctrl Pts',(0.00253969447675147,-0.0207708672591209,
-0.0105788439028333));
#36095=CARTESIAN_POINT('Ctrl Pts',(0.00251416618964412,-0.0207733564043156,
-0.0105389017805349));
#36096=CARTESIAN_POINT('Ctrl Pts',(0.00250025228299103,-0.0207746768609968,
-0.0105177277077988));
#36097=CARTESIAN_POINT('Ctrl Pts',(0.00246153296909395,-0.0207782561566436,
-0.0104604007090515));
#36098=CARTESIAN_POINT('Ctrl Pts',(0.00243620021526385,-0.0207804954096929,
-0.0104246106242727));
#36099=CARTESIAN_POINT('Ctrl Pts',(0.00227740445250603,-0.0207939546857506,
-0.0102103819121834));
#36100=CARTESIAN_POINT('Ctrl Pts',(0.00212519094255011,-0.0208044110159279,
-0.0100467173973649));
#36101=CARTESIAN_POINT('Ctrl Pts',(0.00187603371900854,-0.0208200099993034,
-0.00983241741400301));
#36102=CARTESIAN_POINT('Ctrl Pts',(0.00179222995620551,-0.0208250605404119,
-0.00976772046284651));
#36103=CARTESIAN_POINT('Ctrl Pts',(0.00165733134163275,-0.020833168007507,
-0.00967452637443893));
#36104=CARTESIAN_POINT('Ctrl Pts',(0.00160852474342964,-0.020836097618851,
-0.00964286476406511));
#36105=CARTESIAN_POINT('Ctrl Pts',(0.00154224646274915,-0.0208401129327455,
-0.00960255721782676));
#36106=CARTESIAN_POINT('Ctrl Pts',(0.00152556406545788,-0.0208411266375725,
-0.00959263222495757));
#36107=CARTESIAN_POINT('Ctrl Pts',(0.00149763342765964,-0.0208428308446952,
-0.00957638014054555));
#36108=CARTESIAN_POINT('Ctrl Pts',(0.00148643825423223,-0.020843515780168,
-0.00956996230039344));
#36109=CARTESIAN_POINT('Ctrl Pts',(0.00146485784422212,-0.020844840283607,
-0.00955777524634868));
#36110=CARTESIAN_POINT('Ctrl Pts',(0.00145447917651087,-0.0208454790753456,
-0.00955199516466442));
#36111=CARTESIAN_POINT('Ctrl Pts',(0.00142586328161577,-0.0208472446804427,
-0.00953628036724891));
#36112=CARTESIAN_POINT('Ctrl Pts',(0.00140755711420797,-0.020848378981683,
-0.00952647331817275));
#36113=CARTESIAN_POINT('Ctrl Pts',(0.0013315541525163,-0.0208531034472814,
-0.00948676675088753));
#36114=CARTESIAN_POINT('Ctrl Pts',(0.00127299825484383,-0.0208567787432643,
-0.00945855735008313));
#36115=CARTESIAN_POINT('Ctrl Pts',(0.00106184419740905,-0.02087004091851,
-0.00936515687992956));
#36116=CARTESIAN_POINT('Ctrl Pts',(0.000904808406850817,-0.0208799028571829,
-0.00931074453435733));
#36117=CARTESIAN_POINT('Ctrl Pts',(0.000597498983964137,-0.0208984491060018,
-0.00923206492601655));
#36118=CARTESIAN_POINT('Ctrl Pts',(0.000448273629090484,-0.0209071353400333,
-0.00920567567001786));
#36119=CARTESIAN_POINT('Ctrl Pts',(0.000252605066647527,-0.0209179846881952,
-0.00918616391769422));
#36120=CARTESIAN_POINT('Ctrl Pts',(0.000207433800087171,-0.0209204537919721,
-0.00918269051722269));
#36121=CARTESIAN_POINT('Ctrl Pts',(0.000136850255024302,-0.0209242579269562,
-0.00917886872314797));
#36122=CARTESIAN_POINT('Ctrl Pts',(0.000111484155088653,-0.0209256142168391,
-0.00917781796280831));
#36123=CARTESIAN_POINT('Ctrl Pts',(6.40541183576163E-5,-0.0209281307089639,
-0.00917645604533503));
#36124=CARTESIAN_POINT('Ctrl Pts',(4.19943152725023E-5,-0.0209292932507632,
-0.0091760660852877));
#36125=CARTESIAN_POINT('Ctrl Pts',(-7.57507594749086E-6,-0.0209318886048304,
-0.00917573674204599));
#36126=CARTESIAN_POINT('Ctrl Pts',(-3.5083739688327E-5,-0.0209333171846789,
-0.00917593231115193));
#36127=CARTESIAN_POINT('Ctrl Pts',(-0.000106187070892492,-0.0209369816788542,
-0.00917741600201071));
#36128=CARTESIAN_POINT('Ctrl Pts',(-0.000149763941693255,-0.0209392001892945,
-0.0091792764321678));
#36129=CARTESIAN_POINT('Ctrl Pts',(-0.000428410252006269,-0.0209532404945661,
-0.00919726663890821));
#36130=CARTESIAN_POINT('Ctrl Pts',(-0.000660920002255194,-0.0209642090100372,
-0.0092400904908678));
#36131=CARTESIAN_POINT('Ctrl Pts',(-0.00101503623141154,-0.0209818633078989,
-0.00934955999582587));
#36132=CARTESIAN_POINT('Ctrl Pts',(-0.00114118855565647,-0.0209883789393967,
-0.00939809988093033));
#36133=CARTESIAN_POINT('Ctrl Pts',(-0.00128551591720627,-0.0209965474965692,
-0.00946512807873946));
#36134=CARTESIAN_POINT('Ctrl Pts',(-0.00130727813672281,-0.0209977992555091,
-0.00947555587172245));
#36135=CARTESIAN_POINT('Ctrl Pts',(-0.0013413829062071,-0.0209997963558616,
-0.00949240673324522));
#36136=CARTESIAN_POINT('Ctrl Pts',(-0.00135381103275982,-0.0210005316270779,
-0.00949865527783052));
#36137=CARTESIAN_POINT('Ctrl Pts',(-0.00137738844339629,-0.0210019416829354,
-0.00951071555053032));
#36138=CARTESIAN_POINT('Ctrl Pts',(-0.00138854531996769,-0.021002615528051,
-0.00951651127214551));
#36139=CARTESIAN_POINT('Ctrl Pts',(-0.0014132828749569,-0.0210041238950519,
-0.00952955992511013));
#36140=CARTESIAN_POINT('Ctrl Pts',(-0.00142684481116017,-0.0210049604700519,
-0.00953684762070687));
#36141=CARTESIAN_POINT('Ctrl Pts',(-0.00147349547495861,-0.0210078699817501,
-0.00956238072356904));
#36142=CARTESIAN_POINT('Ctrl Pts',(-0.00150629405645,-0.0210099713015423,
-0.0095811460362178));
#36143=CARTESIAN_POINT('Ctrl Pts',(-0.00170029169243828,-0.0210226977382789,
-0.00969705730843852));
#36144=CARTESIAN_POINT('Ctrl Pts',(-0.0018524058701787,-0.0210338956861871,
-0.00980857451044751));
#36145=CARTESIAN_POINT('Ctrl Pts',(-0.00210317848294954,-0.0210535572724552,
-0.0100314779950751));
#36146=CARTESIAN_POINT('Ctrl Pts',(-0.00220594287360274,-0.0210620658274687,
-0.0101373417623571));
#36147=CARTESIAN_POINT('Ctrl Pts',(-0.00233629980723495,-0.0210733709046007,
-0.0102930865035584));
#36148=CARTESIAN_POINT('Ctrl Pts',(-0.0023708823466686,-0.0210764296494589,
-0.0103368250088186));
#36149=CARTESIAN_POINT('Ctrl Pts',(-0.00242062610603733,-0.0210809225126571,
-0.0104034760853746));
#36150=CARTESIAN_POINT('Ctrl Pts',(-0.00243672300396489,-0.0210823921058821,
-0.0104256725078518));
#36151=CARTESIAN_POINT('Ctrl Pts',(-0.00246521625306922,-0.0210850231150675,
-0.0104661178417662));
#36152=CARTESIAN_POINT('Ctrl Pts',(-0.0024777197584763,-0.021086188514531,
-0.0104842885379199));
#36153=CARTESIAN_POINT('Ctrl Pts',(-0.0025042180518513,-0.0210886827599708,
-0.0105237214006665));
#36154=CARTESIAN_POINT('Ctrl Pts',(-0.00251814498520116,-0.0210900090411845,
-0.0105450272059759));
#36155=CARTESIAN_POINT('Ctrl Pts',(-0.00255561025165671,-0.0210936216693006,
-0.0106039670403765));
#36156=CARTESIAN_POINT('Ctrl Pts',(-0.00257858757427925,-0.0210958877947361,
-0.0106419509078619));
#36157=CARTESIAN_POINT('Ctrl Pts',(-0.00270909250784214,-0.0211090949608693,
-0.0108689144046996));
#36158=CARTESIAN_POINT('Ctrl Pts',(-0.00279666020176482,-0.0211193162988675,
-0.0110686176684838));
#36159=CARTESIAN_POINT('Ctrl Pts',(-0.00289455212634948,-0.0211347996494708,
-0.0113799666564299));
#36160=CARTESIAN_POINT('Ctrl Pts',(-0.00292154022871089,-0.021139991958695,
-0.0114855868122083));
#36161=CARTESIAN_POINT('Ctrl Pts',(-0.00295423467757847,-0.0211482982237187,
-0.0116504952620033));
#36162=CARTESIAN_POINT('Ctrl Pts',(-0.00296402420910677,-0.021151277319334,
-0.0117088808654383));
#36163=CARTESIAN_POINT('Ctrl Pts',(-0.00297473803497446,-0.021155350702416,
-0.0117868610107671));
#36164=CARTESIAN_POINT('Ctrl Pts',(-0.00297720709618309,-0.0211563703266816,
-0.0118062328936693));
#36165=CARTESIAN_POINT('Ctrl Pts',(-0.00298099596312594,-0.0211580816931108,
-0.0118384659940107));
#36166=CARTESIAN_POINT('Ctrl Pts',(-0.00298242211488947,-0.0211587677664061,
-0.011851314474669));
#36167=CARTESIAN_POINT('Ctrl Pts',(-0.0029849967411681,-0.0211600919805377,
-0.0118759616797686));
#36168=CARTESIAN_POINT('Ctrl Pts',(-0.00298615840161401,-0.0211607293153368,
-0.0118877586641524));
#36169=CARTESIAN_POINT('Ctrl Pts',(-0.002989150519189,-0.0211624861302781,
-0.0119201093193191));
#36170=CARTESIAN_POINT('Ctrl Pts',(-0.00299083884355015,-0.0211636129783424,
-0.0119406751235815));
#36171=CARTESIAN_POINT('Ctrl Pts',(-0.00299687158423067,-0.0211682584856751,
-0.0120247948753659));
#36172=CARTESIAN_POINT('Ctrl Pts',(-0.00299940312266734,-0.0211718588700796,
-0.0120884587491634));
#36173=CARTESIAN_POINT('Ctrl Pts',(-0.00300122478128989,-0.0211850926846474,
-0.0123190145293164));
#36174=CARTESIAN_POINT('Ctrl Pts',(-0.00298861888737859,-0.0211950121219328,
-0.0124856941718688));
#36175=CARTESIAN_POINT('Ctrl Pts',(-0.00294478445964149,-0.021211213351149,
-0.0127592840504605));
#36176=CARTESIAN_POINT('Ctrl Pts',(-0.00292136378111559,-0.0212175793809198,
-0.0128670723621105));
#36177=CARTESIAN_POINT('Ctrl Pts',(-0.00287278238565809,-0.021227872998984,
-0.0130432526598134));
#36178=CARTESIAN_POINT('Ctrl Pts',(-0.00285097235238797,-0.0212318876692016,
-0.0131124525409196));
#36179=CARTESIAN_POINT('Ctrl Pts',(-0.00281655284832227,-0.0212374625696946,
-0.0132092665366904));
#36180=CARTESIAN_POINT('Ctrl Pts',(-0.00280600194062214,-0.0212390879730306,
-0.0132375811673358));
#36181=CARTESIAN_POINT('Ctrl Pts',(-0.00278689265475383,-0.021241893208216,
-0.0132865874584071));
#36182=CARTESIAN_POINT('Ctrl Pts',(-0.00277852718755164,-0.0212430792579223,
-0.013307351308735));
#36183=CARTESIAN_POINT('Ctrl Pts',(-0.00276072713277685,-0.0212455190626807,
-0.0133501445134297));
#36184=CARTESIAN_POINT('Ctrl Pts',(-0.00275125940240042,-0.0212467716105276,
-0.0133721584029861));
#36185=CARTESIAN_POINT('Ctrl Pts',(-0.00272592604562911,-0.0212500101571559,
-0.0134291703209422));
#36186=CARTESIAN_POINT('Ctrl Pts',(-0.00270964976913099,-0.0212519822802417,
-0.0134639816550492));
#36187=CARTESIAN_POINT('Ctrl Pts',(-0.00262067485815676,-0.0212622309455375,
-0.013645124990929));
#36188=CARTESIAN_POINT('Ctrl Pts',(-0.00253677635653375,-0.0212701153474075,
-0.0137856572748455));
#36189=CARTESIAN_POINT('Ctrl Pts',(-0.00234962476401415,-0.0212854331205784,
-0.0140478743764583));
#36190=CARTESIAN_POINT('Ctrl Pts',(-0.00224729947677344,-0.0212928536601149,
-0.0141695533335899));
#36191=CARTESIAN_POINT('Ctrl Pts',(-0.00210132351848718,-0.0213030244664125,
-0.0143175476283018));
#36192=CARTESIAN_POINT('Ctrl Pts',(-0.0020659593705846,-0.0213054616750342,
-0.0143516810969872));
#36193=CARTESIAN_POINT('Ctrl Pts',(-0.00200422401679125,-0.021309703513845,
-0.0144084056512836));
#36194=CARTESIAN_POINT('Ctrl Pts',(-0.00197826927830292,-0.0213114832284217,
-0.0144314362355991));
#36195=CARTESIAN_POINT('Ctrl Pts',(-0.00193976699157837,-0.0213141279213132,
-0.0144644249421457));
#36196=CARTESIAN_POINT('Ctrl Pts',(-0.00192752908158028,-0.021314969194496,
-0.0144747416748173));
#36197=CARTESIAN_POINT('Ctrl Pts',(-0.00190564151295149,-0.021316476162103,
-0.0144928955708241));
#36198=CARTESIAN_POINT('Ctrl Pts',(-0.00189602484649981,-0.0213171391262862,
-0.0145007714131726));
#36199=CARTESIAN_POINT('Ctrl Pts',(-0.00187444928540479,-0.0213186285893507,
-0.0145182184331059));
#36200=CARTESIAN_POINT('Ctrl Pts',(-0.00186246597466497,-0.021319457134808,
-0.0145277578501826));
#36201=CARTESIAN_POINT('Ctrl Pts',(-0.00182600704438916,-0.0213219804386885,
-0.0145563279216827));
#36202=CARTESIAN_POINT('Ctrl Pts',(-0.00180130962606329,-0.0213236930573088,
-0.0145750708045668));
#36203=CARTESIAN_POINT('Ctrl Pts',(-0.00166246850104765,-0.0213333187042689,
-0.0146770851821278));
#36204=CARTESIAN_POINT('Ctrl Pts',(-0.00154284994277481,-0.021341595501662,
-0.0147525897628802));
#36205=CARTESIAN_POINT('Ctrl Pts',(-0.00123769929215294,-0.0213619560712537,
-0.0149163164100325));
#36206=CARTESIAN_POINT('Ctrl Pts',(-0.0010475461800233,-0.0213739865394142,
-0.0149944885071188));
#36207=CARTESIAN_POINT('Ctrl Pts',(-0.000796941372126417,-0.0213885390732949,
-0.0150686113769277));
#36208=CARTESIAN_POINT('Ctrl Pts',(-0.000742553655963941,-0.021391626836907,
-0.0150830477353186));
#36209=CARTESIAN_POINT('Ctrl Pts',(-0.000661011412830097,-0.0213961531723039,
-0.0151022539357962));
#36210=CARTESIAN_POINT('Ctrl Pts',(-0.000634147246587491,-0.0213976279996285,
-0.0151081926574016));
#36211=CARTESIAN_POINT('Ctrl Pts',(-0.000585797080727557,-0.021400253865997,
-0.0151181856329597));
#36212=CARTESIAN_POINT('Ctrl Pts',(-0.000564341511285612,-0.0214014091010214,
-0.0151223760760515));
#36213=CARTESIAN_POINT('Ctrl Pts',(-0.000517950754755852,-0.021403886070058,
-0.0151309112462756));
#36214=CARTESIAN_POINT('Ctrl Pts',(-0.000493002415159303,-0.0214052052205168,
-0.015135175708913));
#36215=CARTESIAN_POINT('Ctrl Pts',(-0.000424817909479392,-0.0214087770513755,
-0.0151459443924384));
#36216=CARTESIAN_POINT('Ctrl Pts',(-0.000381488031400211,-0.0214110102869559,
-0.0151518201144713));
#36217=CARTESIAN_POINT('Ctrl Pts',(-0.000115536105605697,-0.0214245212488271,
-0.0151819799918598));
#36218=CARTESIAN_POINT('Ctrl Pts',(0.00010909390890025,-0.0214350259731176,
-0.0151822219030969));
#36219=CARTESIAN_POINT('Ctrl Pts',(0.00043619871549183,-0.0214506497260402,
-0.0151458350794988));
#36220=CARTESIAN_POINT('Ctrl Pts',(0.00054003720482919,-0.0214556717306781,
-0.0151287194743732));
#36221=CARTESIAN_POINT('Ctrl Pts',(0.000699369742092979,-0.0214637390650677,
-0.0150937705616322));
#36222=CARTESIAN_POINT('Ctrl Pts',(0.00075560798319205,-0.0214666585768238,
-0.0150797153789685));
#36223=CARTESIAN_POINT('Ctrl Pts',(0.000830065265031124,-0.0214706620321117,
-0.0150587975330248));
#36224=CARTESIAN_POINT('Ctrl Pts',(0.000848678370577245,-0.0214716745158966,
-0.0150533732009282));
#36225=CARTESIAN_POINT('Ctrl Pts',(0.000879585921006186,-0.021473377248088,
-0.0150440399969895));
#36226=CARTESIAN_POINT('Ctrl Pts',(0.000891910421517026,-0.0214740619506699,
-0.0150402314378059));
#36227=CARTESIAN_POINT('Ctrl Pts',(0.000915542361791507,-0.0214753865219293,
-0.0150327613075562));
#36228=CARTESIAN_POINT('Ctrl Pts',(0.000926853228380179,-0.0214760256205961,
-0.0150291118342597));
#36229=CARTESIAN_POINT('Ctrl Pts',(0.000957894447307013,-0.0214777930729377,
-0.01501889227325));
#36230=CARTESIAN_POINT('Ctrl Pts',(0.000977578290467563,-0.021478928939772,
-0.0150121842070055));
#36231=CARTESIAN_POINT('Ctrl Pts',(0.00105873833926493,-0.0214836703250271,
-0.0149835804509855));
#36232=CARTESIAN_POINT('Ctrl Pts',(0.00111955842974213,-0.021487361715491,
-0.0149598875027504));
#36233=CARTESIAN_POINT('Ctrl Pts',(0.00135038522493828,-0.0215017839381054,
-0.0148611800566739));
#36234=CARTESIAN_POINT('Ctrl Pts',(0.00151405971007277,-0.0215128631267645,
-0.0147724172285096));
#36235=CARTESIAN_POINT('Ctrl Pts',(0.00176702535379605,-0.0215305777122009,
-0.0146031323507912));
#36236=CARTESIAN_POINT('Ctrl Pts',(0.00186158798475756,-0.0215373627190307,
-0.0145313907886546));
#36237=CARTESIAN_POINT('Ctrl Pts',(0.00199176160682566,-0.0215468811248799,
-0.0144198839227839));
#36238=CARTESIAN_POINT('Ctrl Pts',(0.00203094853441844,-0.0215497731835642,
-0.0143844809876869));
#36239=CARTESIAN_POINT('Ctrl Pts',(0.00208863530351017,-0.0215540729979919,
-0.0143295302260942));
#36240=CARTESIAN_POINT('Ctrl Pts',(0.0021078388763649,-0.0215555118916898,
-0.0143107390272776));
#36241=CARTESIAN_POINT('Ctrl Pts',(0.00214081486899442,-0.0215579966934802,
-0.0142775923882731));
#36242=CARTESIAN_POINT('Ctrl Pts',(0.00215470152783834,-0.0215590475385496,
-0.0142633534437889));
#36243=CARTESIAN_POINT('Ctrl Pts',(0.00218577628607213,-0.0215614097863671,
-0.0142308498739207));
#36244=CARTESIAN_POINT('Ctrl Pts',(0.00220287912141226,-0.0215627175309422,
-0.0142125055821429));
#36245=CARTESIAN_POINT('Ctrl Pts',(0.00224844688518236,-0.0215662243281809,
-0.0141623845326164));
#36246=CARTESIAN_POINT('Ctrl Pts',(0.00227646782318025,-0.0215684051462365,
-0.0141302110496065));
#36247=CARTESIAN_POINT('Ctrl Pts',(0.00247375039618694,-0.0215839689152265,
-0.0138936898067993));
#36248=CARTESIAN_POINT('Ctrl Pts',(0.00261591545379976,-0.0215962035866839,
-0.0136682977111132));
#36249=CARTESIAN_POINT('Ctrl Pts',(0.00277112007888546,-0.0216140268087185,
-0.0133301033872699));
#36250=CARTESIAN_POINT('Ctrl Pts',(0.00281043785297068,-0.0216192232928378,
-0.0132307633683977));
#36251=CARTESIAN_POINT('Ctrl Pts',(0.00285347109973722,-0.0216261259518728,
-0.0131024176386094));
#36252=CARTESIAN_POINT('Ctrl Pts',(0.0028621787970604,-0.0216276025656415,
-0.0130751592611842));
#36253=CARTESIAN_POINT('Ctrl Pts',(0.00287480964959381,-0.0216298768994019,
-0.0130335769388411));
#36254=CARTESIAN_POINT('Ctrl Pts',(0.00287901876515703,-0.0216306593803561,
-0.0130193408779302));
#36255=CARTESIAN_POINT('Ctrl Pts',(0.00288656913398805,-0.0216321103404783,
-0.0129930889744409));
#36256=CARTESIAN_POINT('Ctrl Pts',(0.00288994135691478,-0.0216327770897573,
-0.0129810827391017));
#36257=CARTESIAN_POINT('Ctrl Pts',(0.0028975568477285,-0.0216343267955963,
-0.012953304927055));
#36258=CARTESIAN_POINT('Ctrl Pts',(0.00290174629040852,-0.0216352126465991,
-0.0129375193427555));
#36259=CARTESIAN_POINT('Ctrl Pts',(0.00291514339204965,-0.0216381569526274,
-0.0128853245039356));
#36260=CARTESIAN_POINT('Ctrl Pts',(0.00292379595731421,-0.0216402429176858,
-0.0128487777651147));
#36261=CARTESIAN_POINT('Ctrl Pts',(0.00297190863058026,-0.0216530045343649,
-0.0126270724928342));
#36262=CARTESIAN_POINT('Ctrl Pts',(0.00299445353082488,-0.0216642686155563,
-0.0124386886723795));
#36263=CARTESIAN_POINT('Ctrl Pts',(0.0030027274638194,-0.0216840355884287,
-0.0121015036464619));
#36264=CARTESIAN_POINT('Ctrl Pts',(0.00299540642979166,-0.021692583502484,
-0.0119534829003213));
#36265=CARTESIAN_POINT('Ctrl Pts',(0.00297033202492817,-0.0217039223733126,
-0.0117513181493819));
#36266=CARTESIAN_POINT('Ctrl Pts',(0.00296193783075799,-0.0217069785122006,
-0.0116962417083047));
#36267=CARTESIAN_POINT('Ctrl Pts',(0.00294713196708965,-0.0217114683674922,
-0.0116144582447007));
#36268=CARTESIAN_POINT('Ctrl Pts',(0.00294187989719302,-0.0217129374890491,
-0.011587555774586));
#36269=CARTESIAN_POINT('Ctrl Pts',(0.002931737491046,-0.0217155679921089,
-0.0115391416372691));
#36270=CARTESIAN_POINT('Ctrl Pts',(0.00292697722321101,-0.0217167333504085,
-0.0115176049972699));
#36271=CARTESIAN_POINT('Ctrl Pts',(0.00291621147847062,-0.0217192278702063,
-0.0114713259624122));
#36272=CARTESIAN_POINT('Ctrl Pts',(0.00291012764128102,-0.0217205544616695,
-0.0114466034657669));
#36273=CARTESIAN_POINT('Ctrl Pts',(0.00289256829316838,-0.0217241688677026,
-0.011378971000477));
#36274=CARTESIAN_POINT('Ctrl Pts',(0.00288045321620186,-0.0217264364266493,
-0.0113362329946691));
#36275=CARTESIAN_POINT('Ctrl Pts',(0.00280355853226712,-0.0217396288571486,
-0.0110862686529421));
#36276=CARTESIAN_POINT('Ctrl Pts',(0.00271738883586907,-0.0217498365236231,
-0.0108863027527758));
#36277=CARTESIAN_POINT('Ctrl Pts',(0.0025566054011644,-0.0217653133966032,
-0.0106024248559886));
#36278=CARTESIAN_POINT('Ctrl Pts',(0.00249768783074411,-0.0217705141299547,
-0.0105104820760344));
#36279=CARTESIAN_POINT('Ctrl Pts',(0.002399256479319,-0.0217788321778329,
-0.0103738879571371));
#36280=CARTESIAN_POINT('Ctrl Pts',(0.00236320185483031,-0.021781814178055,
-0.0103268571094016));
#36281=CARTESIAN_POINT('Ctrl Pts',(0.00231344136213341,-0.0217858909679136,
-0.0102657824247298));
#36282=CARTESIAN_POINT('Ctrl Pts',(0.00230095463788213,-0.0217869109363552,
-0.0102507586528688));
#36283=CARTESIAN_POINT('Ctrl Pts',(0.00227996183846282,-0.0217886227194699,
-0.0102259965822281));
#36284=CARTESIAN_POINT('Ctrl Pts',(0.00227153770091601,-0.0217893088593279,
-0.0102161891265516));
#36285=CARTESIAN_POINT('Ctrl Pts',(0.00225526953057183,-0.0217906330585487,
-0.0101974954244839));
#36286=CARTESIAN_POINT('Ctrl Pts',(0.002247435789575,-0.0217912703101578,
-0.0101886006986672));
#36287=CARTESIAN_POINT('Ctrl Pts',(0.00222582488967767,-0.0217930266221008,
-0.0101643540818985));
#36288=CARTESIAN_POINT('Ctrl Pts',(0.00221194201716796,-0.0217941530435087,
-0.010149097762112));
#36289=CARTESIAN_POINT('Ctrl Pts',(0.00215459533492618,-0.0217987941089578,
-0.0100873687365295));
#36290=CARTESIAN_POINT('Ctrl Pts',(0.00210981782575442,-0.0218023902888924,
-0.0100421437281432));
#36291=CARTESIAN_POINT('Ctrl Pts',(0.00194248262051159,-0.021815622521921,
-0.00988355649016529));
#36292=CARTESIAN_POINT('Ctrl Pts',(0.00181195642250678,-0.0218255452048675,
-0.00977904788177661));
#36293=CARTESIAN_POINT('Ctrl Pts',(0.00158192632857605,-0.0218417509279117,
-0.0096244496106172));
#36294=CARTESIAN_POINT('Ctrl Pts',(0.00148710991988152,-0.0218481182380285,
-0.00956804598993847));
#36295=CARTESIAN_POINT('Ctrl Pts',(0.00132510879460373,-0.0218584136150603,
-0.00948339190283278));
#36296=CARTESIAN_POINT('Ctrl Pts',(0.00125961949759353,-0.0218624288033541,
-0.00945213862613759));
#36297=CARTESIAN_POINT('Ctrl Pts',(0.00116533420114157,-0.0218680042792457,
-0.00941127209320417));
#36298=CARTESIAN_POINT('Ctrl Pts',(0.00113743024086137,-0.0218696297582169,
-0.00939967506590343));
#36299=CARTESIAN_POINT('Ctrl Pts',(0.00108855702388138,-0.0218724350804154,
-0.00938022371796871));
#36300=CARTESIAN_POINT('Ctrl Pts',(0.00106766656590156,-0.0218736211426054,
-0.0093721790509184));
#36301=CARTESIAN_POINT('Ctrl Pts',(0.00102423166521441,-0.0218760609338708,
-0.00935600867056513));
#36302=CARTESIAN_POINT('Ctrl Pts',(0.00100167593238024,-0.0218773134562668,
-0.00934791772636746));
#36303=CARTESIAN_POINT('Ctrl Pts',(0.000942707344764414,-0.0218805518515019,
-0.009327559224151));
#36304=CARTESIAN_POINT('Ctrl Pts',(0.000906150956446747,-0.0218825238511704,
-0.00931571923059809));
#36305=CARTESIAN_POINT('Ctrl Pts',(0.000713049804537019,-0.0218927696662601,
-0.00925725116838311));
#36306=CARTESIAN_POINT('Ctrl Pts',(0.000553109596414376,-0.0219006516266715,
-0.00922276080093842));
#36307=CARTESIAN_POINT('Ctrl Pts',(0.000233712367778685,-0.0219159692029597,
-0.00918075848110149));
#36308=CARTESIAN_POINT('Ctrl Pts',(7.48903184489933E-5,-0.0219233918215225,
-0.00917258820905025));
#36309=CARTESIAN_POINT('Ctrl Pts',(-0.000132955502815853,-0.0219335651874415,
-0.00917839791636385));
#36310=CARTESIAN_POINT('Ctrl Pts',(-0.00018204457507849,-0.0219360027229384,
-0.00918097845890368));
#36311=CARTESIAN_POINT('Ctrl Pts',(-0.000265644717133675,-0.0219402450735879,
-0.00918743612987579));
#36312=CARTESIAN_POINT('Ctrl Pts',(-0.000300193144802116,-0.0219420249651103,
-0.00919070871709235));
#36313=CARTESIAN_POINT('Ctrl Pts',(-0.000350582718806955,-0.0219446698729446,
-0.00919636541408512));
#36314=CARTESIAN_POINT('Ctrl Pts',(-0.000366474935124503,-0.0219455111786728,
-0.00919827837994413));
#36315=CARTESIAN_POINT('Ctrl Pts',(-0.000394680110815065,-0.0219470181799374,
-0.00920190269286606));
#36316=CARTESIAN_POINT('Ctrl Pts',(-0.000406998854596002,-0.0219476811446947,
-0.00920356352157882));
#36317=CARTESIAN_POINT('Ctrl Pts',(-0.000434473099811644,-0.0219491705776657,
-0.00920744163858167));
#36318=CARTESIAN_POINT('Ctrl Pts',(-0.000449622029310982,-0.021949999091974,
-0.00920969843609453));
#36319=CARTESIAN_POINT('Ctrl Pts',(-0.000495379012331518,-0.0219525222051482,
-0.00921687361943071));
#36320=CARTESIAN_POINT('Ctrl Pts',(-0.000525927913363199,-0.0219542346604364,
-0.00922215040384301));
#36321=CARTESIAN_POINT('Ctrl Pts',(-0.000698268341881028,-0.0219640330920767,
-0.00925467744159176));
#36322=CARTESIAN_POINT('Ctrl Pts',(-0.000838020304194822,-0.0219724991807633,
-0.00929166136062239));
#36323=CARTESIAN_POINT('Ctrl Pts',(-0.00112197445151132,-0.0219901538864227,
-0.00938919404126638));
#36324=CARTESIAN_POINT('Ctrl Pts',(-0.00126523405204063,-0.0219993148720676,
-0.00945124579585816));
#36325=CARTESIAN_POINT('Ctrl Pts',(-0.00145641618585282,-0.0220116177100778,
-0.00955240137190435));
#36326=CARTESIAN_POINT('Ctrl Pts',(-0.00150893992611529,-0.0220150087000287,
-0.00958225558945518));
#36327=CARTESIAN_POINT('Ctrl Pts',(-0.00160096939735291,-0.0220209650181399,
-0.00963830740734429));
#36328=CARTESIAN_POINT('Ctrl Pts',(-0.0016408224100256,-0.0220235496703174,
-0.00966389304307682));
#36329=CARTESIAN_POINT('Ctrl Pts',(-0.00170143074430163,-0.022027490017923,
-0.00970486175621376));
#36330=CARTESIAN_POINT('Ctrl Pts',(-0.0017226199654381,-0.0220288695109033,
-0.00971958656005426));
#36331=CARTESIAN_POINT('Ctrl Pts',(-0.00176154538277091,-0.0220314079841257,
-0.00974738808106528));
#36332=CARTESIAN_POINT('Ctrl Pts',(-0.0017793324229179,-0.0220325696500739,
-0.00976039027645391));
#36333=CARTESIAN_POINT('Ctrl Pts',(-0.00181857258874413,-0.0220351369951552,
-0.00978974322909495));
#36334=CARTESIAN_POINT('Ctrl Pts',(-0.00183995181243218,-0.0220365388692148,
-0.00980618983867333));
#36335=CARTESIAN_POINT('Ctrl Pts',(-0.00189385431099838,-0.0220400834199648,
-0.00984882531421506));
#36336=CARTESIAN_POINT('Ctrl Pts',(-0.00192605841184427,-0.0220422106275502,
-0.00987540929877964));
#36337=CARTESIAN_POINT('Ctrl Pts',(-0.00210026431969435,-0.0220537927483132,
-0.0100254371190867));
#36338=CARTESIAN_POINT('Ctrl Pts',(-0.00223097199378551,-0.0220627306866264,
-0.0101613629732309));
#36339=CARTESIAN_POINT('Ctrl Pts',(-0.00242805632135967,-0.0220777329034768,
-0.0104092038783085));
#36340=CARTESIAN_POINT('Ctrl Pts',(-0.00250147726794621,-0.0220838043314496,
-0.010514794645838));
#36341=CARTESIAN_POINT('Ctrl Pts',(-0.00259072448680345,-0.0220922945642758,
-0.0106625471479935));
#36342=CARTESIAN_POINT('Ctrl Pts',(-0.00261271141670614,-0.0220944945843775,
-0.0107008320724447));
#36343=CARTESIAN_POINT('Ctrl Pts',(-0.00264919515476018,-0.0220983627385461,
-0.0107677364301181));
#36344=CARTESIAN_POINT('Ctrl Pts',(-0.00266409274639131,-0.0221000114360775,
-0.0107961294979881));
#36345=CARTESIAN_POINT('Ctrl Pts',(-0.00268552129340751,-0.0221024965732946,
-0.0108386112601502));
#36346=CARTESIAN_POINT('Ctrl Pts',(-0.00269240296945313,-0.0221033131810294,
-0.0108525214747711));
#36347=CARTESIAN_POINT('Ctrl Pts',(-0.00270406198285871,-0.022104730099961,
-0.0108765557455737));
#36348=CARTESIAN_POINT('Ctrl Pts',(-0.00270889105787199,-0.0221053272852062,
-0.010886654102348));
#36349=CARTESIAN_POINT('Ctrl Pts',(-0.00272012001133121,-0.0221067405482624,
-0.0109104772793919));
#36350=CARTESIAN_POINT('Ctrl Pts',(-0.00272647247867412,-0.0221075593571746,
-0.0109242235014021));
#36351=CARTESIAN_POINT('Ctrl Pts',(-0.00274514505802295,-0.0221100234681322,
-0.0109654461876865));
#36352=CARTESIAN_POINT('Ctrl Pts',(-0.00275715551332704,-0.0221116854769967,
-0.010993059951077));
#36353=CARTESIAN_POINT('Ctrl Pts',(-0.00283612734214268,-0.0221231336134954,
-0.0111823692331312));
#36354=CARTESIAN_POINT('Ctrl Pts',(-0.00288923950074892,-0.0221334843104636,
-0.0113494656580827));
#36355=CARTESIAN_POINT('Ctrl Pts',(-0.00295710066008395,-0.0221517345325836,
-0.0116524764824545));
#36356=CARTESIAN_POINT('Ctrl Pts',(-0.00297772528765525,-0.0221596437306527,
-0.0117865914270376));
#36357=CARTESIAN_POINT('Ctrl Pts',(-0.00299620029652009,-0.0221719987161479,
-0.0120038413913217));
#36358=CARTESIAN_POINT('Ctrl Pts',(-0.00299979743429729,-0.0221765855549523,
-0.0120862909117538));
#36359=CARTESIAN_POINT('Ctrl Pts',(-0.00300006613385393,-0.0221827892278334,
-0.0122004087489637));
#36360=CARTESIAN_POINT('Ctrl Pts',(-0.00299964069417185,-0.0221844929160432,
-0.0122320279070503));
#36361=CARTESIAN_POINT('Ctrl Pts',(-0.00299806021748773,-0.0221873769809811,
-0.0122860184767575));
#36362=CARTESIAN_POINT('Ctrl Pts',(-0.00299715438798948,-0.0221885648940955,
-0.0123083940273983));
#36363=CARTESIAN_POINT('Ctrl Pts',(-0.00299478752303314,-0.0221909808071725,
-0.0123541714208326));
#36364=CARTESIAN_POINT('Ctrl Pts',(-0.00299330250209953,-0.0221922079845099,
-0.0123775705072845));
#36365=CARTESIAN_POINT('Ctrl Pts',(-0.00298884842571801,-0.0221952941349685,
-0.0124367652798569));
#36366=CARTESIAN_POINT('Ctrl Pts',(-0.00298551052183768,-0.0221971416924579,
-0.012472529952921));
#36367=CARTESIAN_POINT('Ctrl Pts',(-0.00296771426552442,-0.0222053220867497,
-0.0126321697723249));
#36368=CARTESIAN_POINT('Ctrl Pts',(-0.00294618197791558,-0.0222114371849998,
-0.0127551360597183));
#36369=CARTESIAN_POINT('Ctrl Pts',(-0.00288909348363007,-0.0222231872977006,
-0.0129928459641426));
#36370=CARTESIAN_POINT('Ctrl Pts',(-0.00285418507381699,-0.0222288222154665,
-0.013107500304734));
#36371=CARTESIAN_POINT('Ctrl Pts',(-0.00276086151948031,-0.0222415624585182,
-0.0133589345842988));
#36372=CARTESIAN_POINT('Ctrl Pts',(-0.0026989510516914,-0.0222486784599728,
-0.0134940687630364));
#36373=CARTESIAN_POINT('Ctrl Pts',(-0.00261548014216787,-0.0222575493354705,
-0.0136455006917983));
#36374=CARTESIAN_POINT('Ctrl Pts',(-0.00260339506845473,-0.0222588192365489,
-0.0136668039611273));
#36375=CARTESIAN_POINT('Ctrl Pts',(-0.0025840005302212,-0.0222608387541011,
-0.0137000373043808));
#36376=CARTESIAN_POINT('Ctrl Pts',(-0.00257686589707012,-0.0222615779177206,
-0.0137120686990122));
#36377=CARTESIAN_POINT('Ctrl Pts',(-0.00256310140165208,-0.0222629977254138,
-0.0137349145765833));
#36378=CARTESIAN_POINT('Ctrl Pts',(-0.00255648670917778,-0.0222636774529654,
-0.0137457375452049));
#36379=CARTESIAN_POINT('Ctrl Pts',(-0.00254020917814553,-0.0222653434369309,
-0.0137719951758081));
#36380=CARTESIAN_POINT('Ctrl Pts',(-0.00253047412683002,-0.0222663341560335,
-0.0137873843163532));
#36381=CARTESIAN_POINT('Ctrl Pts',(-0.00249421876549608,-0.022270000568166,
-0.0138435581304638));
#36382=CARTESIAN_POINT('Ctrl Pts',(-0.00246684872924702,-0.0222727238273082,
-0.0138837828909727));
#36383=CARTESIAN_POINT('Ctrl Pts',(-0.00239207133013985,-0.0222800140460087,
-0.0139881313970417));
#36384=CARTESIAN_POINT('Ctrl Pts',(-0.00234306512956684,-0.0222846436701589,
-0.0140510604152399));
#36385=CARTESIAN_POINT('Ctrl Pts',(-0.00212251389387266,-0.0223046481960207,
-0.0143121091987214));
#36386=CARTESIAN_POINT('Ctrl Pts',(-0.00192788479875701,-0.0223201747986316,
-0.0144892833378718));
#36387=CARTESIAN_POINT('Ctrl Pts',(-0.00167708118250625,-0.0223370070963812,
-0.0146636796448001));
#36388=CARTESIAN_POINT('Ctrl Pts',(-0.00164093642426968,-0.0223393693352635,
-0.014687667212669));
#36389=CARTESIAN_POINT('Ctrl Pts',(-0.00158296019067432,-0.0223430605417988,
-0.0147243575108832));
#36390=CARTESIAN_POINT('Ctrl Pts',(-0.00156146768515415,-0.0223444083038223,
-0.014737582286195));
#36391=CARTESIAN_POINT('Ctrl Pts',(-0.00152104224537875,-0.0223469058372614,
-0.0147617590700424));
#36392=CARTESIAN_POINT('Ctrl Pts',(-0.00150215157867311,-0.0223480579621607,
-0.0147727781799165));
#36393=CARTESIAN_POINT('Ctrl Pts',(-0.00145913475852153,-0.0223506486410041,
-0.0147972438569291));
#36394=CARTESIAN_POINT('Ctrl Pts',(-0.00143493985121314,-0.0223520827399218,
-0.0148105658809706));
#36395=CARTESIAN_POINT('Ctrl Pts',(-0.00136039271092404,-0.0223564341551935,
-0.0148502809346667));
#36396=CARTESIAN_POINT('Ctrl Pts',(-0.00130947016684187,-0.0223593139268372,
-0.0148755791933653));
#36397=CARTESIAN_POINT('Ctrl Pts',(-0.00118760376923174,-0.0223660153684573,
-0.0149318622843445));
#36398=CARTESIAN_POINT('Ctrl Pts',(-0.00111611861718849,-0.0223697985100823,
-0.014961579134383));
#36399=CARTESIAN_POINT('Ctrl Pts',(-0.000923635682447565,-0.0223797014644557,
-0.0150329950647879));
#36400=CARTESIAN_POINT('Ctrl Pts',(-0.00080098508514844,-0.0223857198465289,
-0.0150697754669045));
#36401=CARTESIAN_POINT('Ctrl Pts',(-0.000539947572133343,-0.0223984430494374,
-0.0151301826462491));
#36402=CARTESIAN_POINT('Ctrl Pts',(-0.000401502187463013,-0.0224051445719702,
-0.0151521587846218));
#36403=CARTESIAN_POINT('Ctrl Pts',(-0.000231165498714199,-0.0224138358757515,
-0.0151670943760587));
#36404=CARTESIAN_POINT('Ctrl Pts',(-0.00020024913034703,-0.0224154313853954,
-0.0151693229937273));
#36405=CARTESIAN_POINT('Ctrl Pts',(-0.000154014054578636,-0.0224178515147535,
-0.0151719364345054));
#36406=CARTESIAN_POINT('Ctrl Pts',(-0.000138717090381707,-0.0224186577817739,
-0.0151726836300155));
#36407=CARTESIAN_POINT('Ctrl Pts',(-0.000110995066660502,-0.0224201300717305,
-0.0151738250378248));
#36408=CARTESIAN_POINT('Ctrl Pts',(-9.85723484036395E-5,-0.0224207939515171,
-0.0151742591971416));
#36409=CARTESIAN_POINT('Ctrl Pts',(-7.01456901468166E-5,-0.022422322497064,
-0.0151750758259489));
#36410=CARTESIAN_POINT('Ctrl Pts',(-5.41411408996982E-5,-0.0224231897987845,
-0.0151754074155413));
#36411=CARTESIAN_POINT('Ctrl Pts',(-3.43016299497264E-6,-0.0224259574924225,
-0.0151760520897919));
#36412=CARTESIAN_POINT('Ctrl Pts',(3.12783665409965E-5,-0.0224278808984236,
-0.0151758909675471));
#36413=CARTESIAN_POINT('Ctrl Pts',(0.000115125658412668,-0.0224325852705832,
-0.0151740465859631));
#36414=CARTESIAN_POINT('Ctrl Pts',(0.000164240481776405,-0.0224353889560151,
-0.015171757427574));
#36415=CARTESIAN_POINT('Ctrl Pts',(0.000371733148112998,-0.0224473794009763,
-0.0151569690381535));
#36416=CARTESIAN_POINT('Ctrl Pts',(0.000529041856396036,-0.0224568150509789,
-0.0151331072210719));
#36417=CARTESIAN_POINT('Ctrl Pts',(0.000842667011886648,-0.0224756435907731,
-0.0150596980503088));
#36418=CARTESIAN_POINT('Ctrl Pts',(0.0009983284072594,-0.0224849933752691,
-0.0150095789023201));
#36419=CARTESIAN_POINT('Ctrl Pts',(0.00118464014059581,-0.0224960464107419,
-0.0149323190444764));
#36420=CARTESIAN_POINT('Ctrl Pts',(0.0012198405390155,-0.0224981295230377,
-0.0149169233298935));
#36421=CARTESIAN_POINT('Ctrl Pts',(0.00127650075573758,-0.0225014753064585,
-0.0148908339352574));
#36422=CARTESIAN_POINT('Ctrl Pts',(0.00129814439834198,-0.0225027516175345,
-0.0148805520254744));
#36423=CARTESIAN_POINT('Ctrl Pts',(0.00133976615710941,-0.022505203294868,
-0.0148601646965864));
#36424=CARTESIAN_POINT('Ctrl Pts',(0.00135975884324625,-0.0225063797011921,
-0.014850092809491));
#36425=CARTESIAN_POINT('Ctrl Pts',(0.00140647101227962,-0.0225091263036935,
-0.0148259009212793));
#36426=CARTESIAN_POINT('Ctrl Pts',(0.00143309381572103,-0.0225106900898947,
-0.0148115989828092));
#36427=CARTESIAN_POINT('Ctrl Pts',(0.00152289044467476,-0.0225159633104295,
-0.0147615968092931));
#36428=CARTESIAN_POINT('Ctrl Pts',(0.00158498533151552,-0.0225196068228695,
-0.0147240070075853));
#36429=CARTESIAN_POINT('Ctrl Pts',(0.00173787272045709,-0.0225286315201982,
-0.0146237016948439));
#36430=CARTESIAN_POINT('Ctrl Pts',(0.00182668324072589,-0.0225339220731381,
-0.0145581617647929));
#36431=CARTESIAN_POINT('Ctrl Pts',(0.00204043508879636,-0.0225471067924608,
-0.014381422086363));
#36432=CARTESIAN_POINT('Ctrl Pts',(0.00216005926051084,-0.0225549086665976,
-0.0142644046738105));
#36433=CARTESIAN_POINT('Ctrl Pts',(0.00231082028504639,-0.0225662505602816,
-0.0140900466921178));
#36434=CARTESIAN_POINT('Ctrl Pts',(0.00235078930311023,-0.0225694322918355,
-0.0140407434832586));
#36435=CARTESIAN_POINT('Ctrl Pts',(0.00240162659897542,-0.022573773316639,
-0.0139738005642736));
#36436=CARTESIAN_POINT('Ctrl Pts',(0.0024139209104093,-0.0225748475444231,
-0.0139572601820664));
#36437=CARTESIAN_POINT('Ctrl Pts',(0.00243301373169981,-0.0225765569991578,
-0.0139310127049008));
#36438=CARTESIAN_POINT('Ctrl Pts',(0.00243992701338234,-0.0225771847431408,
-0.013921389468448));
#36439=CARTESIAN_POINT('Ctrl Pts',(0.00245426591355026,-0.022578505809994,
-0.0139011782035867));
#36440=CARTESIAN_POINT('Ctrl Pts',(0.0024616803286926,-0.0225791999030353,
-0.0138905827648177));
#36441=CARTESIAN_POINT('Ctrl Pts',(0.002480131856961,-0.0225809544236205,
-0.0138638486210385));
#36442=CARTESIAN_POINT('Ctrl Pts',(0.00249108004436049,-0.0225820204401341,
-0.0138476494612212));
#36443=CARTESIAN_POINT('Ctrl Pts',(0.00253464584589147,-0.0225863609092288,
-0.0137818104555379));
#36444=CARTESIAN_POINT('Ctrl Pts',(0.0025659426011696,-0.0225897073016119,
-0.0137313164614743));
#36445=CARTESIAN_POINT('Ctrl Pts',(0.00265065524652938,-0.0225993744060296,
-0.0135851203895325));
#36446=CARTESIAN_POINT('Ctrl Pts',(0.00270035450372961,-0.0226058094553392,
-0.0134873755430876));
#36447=CARTESIAN_POINT('Ctrl Pts',(0.00283193651514683,-0.0226249749353865,
-0.0131892294871944));
#36448=CARTESIAN_POINT('Ctrl Pts',(0.00289762989870859,-0.0226376229889528,
-0.0129824276156023));
#36449=CARTESIAN_POINT('Ctrl Pts',(0.002949323349224,-0.0226520122311989,
-0.0127267349323925));
#36450=CARTESIAN_POINT('Ctrl Pts',(0.00295716772792673,-0.0226544368677631,
-0.0126829411705067));
#36451=CARTESIAN_POINT('Ctrl Pts',(0.00296796806537692,-0.0226582025795226,
-0.0126138195551786));
#36452=CARTESIAN_POINT('Ctrl Pts',(0.00297157994979023,-0.0226595637321218,
-0.0125886020549129));
#36453=CARTESIAN_POINT('Ctrl Pts',(0.00297771884988576,-0.0226620847460379,
-0.0125414717133667));
#36454=CARTESIAN_POINT('Ctrl Pts',(0.0029803262215699,-0.0226632470201509,
-0.0125195712387592));
#36455=CARTESIAN_POINT('Ctrl Pts',(0.00298562969415798,-0.0226658360833862,
-0.0124704130636376));
#36456=CARTESIAN_POINT('Ctrl Pts',(0.00298819450458233,-0.0226672587347878,
-0.0124431430168683));
#36457=CARTESIAN_POINT('Ctrl Pts',(0.0029948326521407,-0.0226715353304101,
-0.0123604278865456));
#36458=CARTESIAN_POINT('Ctrl Pts',(0.00299773879177757,-0.0226743536673376,
-0.0123048998635374));
#36459=CARTESIAN_POINT('Ctrl Pts',(0.003002749106918,-0.0226845779136009,
-0.0121003682146989));
#36460=CARTESIAN_POINT('Ctrl Pts',(0.00299529632880228,-0.022691709560899,
-0.0119513435583257));
#36461=CARTESIAN_POINT('Ctrl Pts',(0.0029531023130733,-0.022707838376723,
-0.0116140360066398));
#36462=CARTESIAN_POINT('Ctrl Pts',(0.00291137573080329,-0.0227167550548723,
-0.0114273017333655));
#36463=CARTESIAN_POINT('Ctrl Pts',(0.00284214618952716,-0.0227280377211407,
-0.01121499094986));
#36464=CARTESIAN_POINT('Ctrl Pts',(0.0028315952364804,-0.0227296968193252,
-0.0111843293811954));
#36465=CARTESIAN_POINT('Ctrl Pts',(0.00281514967861382,-0.0227322052645117,
-0.0111389427038347));
#36466=CARTESIAN_POINT('Ctrl Pts',(0.00280963164633446,-0.0227330350391886,
-0.0111240827506006));
#36467=CARTESIAN_POINT('Ctrl Pts',(0.00279948762523685,-0.0227345406621734,
-0.0110974146678914));
#36468=CARTESIAN_POINT('Ctrl Pts',(0.00279490395685265,-0.0227352141113977,
-0.0110855906179998));
#36469=CARTESIAN_POINT('Ctrl Pts',(0.00278521988879893,-0.0227366234938713,
-0.0110610719950753));
#36470=CARTESIAN_POINT('Ctrl Pts',(0.00278010743530948,-0.022737360072112,
-0.0110483827591145));
#36471=CARTESIAN_POINT('Ctrl Pts',(0.00276614362526174,-0.0227393513211228,
-0.0110143967265378));
#36472=CARTESIAN_POINT('Ctrl Pts',(0.00275713333421183,-0.0227406147655919,
-0.0109931666798029));
#36473=CARTESIAN_POINT('Ctrl Pts',(0.00270570164132528,-0.0227477023053815,
-0.0108757660176438));
#36474=CARTESIAN_POINT('Ctrl Pts',(0.0026584963238782,-0.0227537527298463,
-0.0107817794216991));
#36475=CARTESIAN_POINT('Ctrl Pts',(0.00250148702830404,-0.0227722598170136,
-0.0105062685323013));
#36476=CARTESIAN_POINT('Ctrl Pts',(0.00237726799819849,-0.0227848745162435,
-0.0103336908587693));
#36477=CARTESIAN_POINT('Ctrl Pts',(0.00217911778439241,-0.0228017556413523,
-0.0101121926451168));
#36478=CARTESIAN_POINT('Ctrl Pts',(0.00211967007436097,-0.0228065007385733,
-0.0100511767805065));
#36479=CARTESIAN_POINT('Ctrl Pts',(0.00203379013168693,-0.0228129266850183,
-0.00997022921803805));
#36480=CARTESIAN_POINT('Ctrl Pts',(0.00200950818109512,-0.0228146995771691,
-0.00994808381507069));
#36481=CARTESIAN_POINT('Ctrl Pts',(0.00196944927229389,-0.0228175548744493,
-0.00991273766544224));
#36482=CARTESIAN_POINT('Ctrl Pts',(0.00195389224793098,-0.0228186472542774,
-0.00989929275308995));
#36483=CARTESIAN_POINT('Ctrl Pts',(0.00192082308474554,-0.0228209353600627,
-0.00987130195295136));
#36484=CARTESIAN_POINT('Ctrl Pts',(0.00190328107853154,-0.0228221295486507,
-0.00985679327310194));
#36485=CARTESIAN_POINT('Ctrl Pts',(0.00186034961519805,-0.022825006151969,
-0.00982210071252365));
#36486=CARTESIAN_POINT('Ctrl Pts',(0.00183479442940087,-0.0228266802986708,
-0.00980212596924957));
#36487=CARTESIAN_POINT('Ctrl Pts',(0.0017380103619275,-0.0228328856380354,
-0.0097289735191961));
#36488=CARTESIAN_POINT('Ctrl Pts',(0.00166475097203775,-0.022837313136912,
-0.00967855343167439));
#36489=CARTESIAN_POINT('Ctrl Pts',(0.00145827531335508,-0.0228492092109301,
-0.00954957844397204));
#36490=CARTESIAN_POINT('Ctrl Pts',(0.00132105944640269,-0.022856480624913,
-0.00947794847188107));
#36491=CARTESIAN_POINT('Ctrl Pts',(0.00104442860403589,-0.0228707544211676,
-0.00935972736946574));
#36492=CARTESIAN_POINT('Ctrl Pts',(0.000905909573580902,-0.0228777362502304,
-0.00931216398627652));
#36493=CARTESIAN_POINT('Ctrl Pts',(0.000734529195063823,-0.0228867449418894,
-0.00926700010677626));
#36494=CARTESIAN_POINT('Ctrl Pts',(0.00070444943541359,-0.0228883398212591,
-0.00925956955350818));
#36495=CARTESIAN_POINT('Ctrl Pts',(0.00065934003519541,-0.0228907591794718,
-0.00924916485052493));
#36496=CARTESIAN_POINT('Ctrl Pts',(0.000644393129839122,-0.0228915653228285,
-0.00924583759409903));
#36497=CARTESIAN_POINT('Ctrl Pts',(0.000617267434001677,-0.0228930374964899,
-0.00924001687355079));
#36498=CARTESIAN_POINT('Ctrl Pts',(0.00060509771003202,-0.0228937013857558,
-0.00923748447434438));
#36499=CARTESIAN_POINT('Ctrl Pts',(0.000577217386921786,-0.022895230096769,
-0.00923186340251633));
#36500=CARTESIAN_POINT('Ctrl Pts',(0.000561497558760526,-0.0228960975568538,
-0.00922882481404518));
#36501=CARTESIAN_POINT('Ctrl Pts',(0.000511610527919068,-0.0228988662801009,
-0.00921959545242807));
#36502=CARTESIAN_POINT('Ctrl Pts',(0.000477360835994778,-0.0229007905804083,
-0.00921387216832633));
#36503=CARTESIAN_POINT('Ctrl Pts',(0.000394367173750417,-0.022905497614691,
-0.00920148032707446));
#36504=CARTESIAN_POINT('Ctrl Pts',(0.000345544041368787,-0.0229083030992029,
-0.00919541391209181));
#36505=CARTESIAN_POINT('Ctrl Pts',(0.000138308451148491,-0.0229203074734349,
-0.00917482461799437));
#36506=CARTESIAN_POINT('Ctrl Pts',(-2.09767918662082E-5,-0.0229297557057958,
-0.00917171251906662));
#36507=CARTESIAN_POINT('Ctrl Pts',(-0.000342466307622283,-0.0229485812984738,
-0.00919101044932174));
#36508=CARTESIAN_POINT('Ctrl Pts',(-0.000504126132214393,-0.0229579165995115,
-0.00921402295924528));
#36509=CARTESIAN_POINT('Ctrl Pts',(-0.000700588261347361,-0.022968955784303,
-0.00925855127254133));
#36510=CARTESIAN_POINT('Ctrl Pts',(-0.000737878009532388,-0.0229710383253205,
-0.00926775920595564));
#36511=CARTESIAN_POINT('Ctrl Pts',(-0.000798126993262842,-0.0229743834280791,
-0.00928387000461224));
#36512=CARTESIAN_POINT('Ctrl Pts',(-0.000821197557063287,-0.0229756596194627,
-0.00929033624143045));
#36513=CARTESIAN_POINT('Ctrl Pts',(-0.00086567022482869,-0.0229781112188349,
-0.0093033776640103));
#36514=CARTESIAN_POINT('Ctrl Pts',(-0.000887080988239808,-0.0229792876647352,
-0.0093099174016066));
#36515=CARTESIAN_POINT('Ctrl Pts',(-0.000937222337681476,-0.0229820345896755,
-0.00932584840906725));
#36516=CARTESIAN_POINT('Ctrl Pts',(-0.000965888416280869,-0.0229835986541698,
-0.0093354355066179));
#36517=CARTESIAN_POINT('Ctrl Pts',(-0.00106289789811331,-0.0229888740268977,
-0.00936951789488818));
#36518=CARTESIAN_POINT('Ctrl Pts',(-0.00113049717084552,-0.0229925193368616,
-0.00939606059001765));
#36519=CARTESIAN_POINT('Ctrl Pts',(-0.00129827759875929,-0.0230015499381171,
-0.00946907330223513));
#36520=CARTESIAN_POINT('Ctrl Pts',(-0.00139698078253561,-0.0230068444297298,
-0.00951866883164786));
#36521=CARTESIAN_POINT('Ctrl Pts',(-0.00163783387362543,-0.023020043552775,
-0.0096568289468316));
#36522=CARTESIAN_POINT('Ctrl Pts',(-0.00177571317877768,-0.0230278557468406,
-0.0097520505103187));
#36523=CARTESIAN_POINT('Ctrl Pts',(-0.00195372373463717,-0.0230391965145519,
-0.00989836499833351));
#36524=CARTESIAN_POINT('Ctrl Pts',(-0.00200123607809152,-0.0230423640171239,
-0.00993999941923989));
#36525=CARTESIAN_POINT('Ctrl Pts',(-0.00206243655992725,-0.0230466883961414,
-0.00999714291755532));
#36526=CARTESIAN_POINT('Ctrl Pts',(-0.00207733177614196,-0.0230477610313858,
-0.0100113403892821));
#36527=CARTESIAN_POINT('Ctrl Pts',(-0.00210056755779622,-0.0230494685627229,
-0.0100339484814817));
#36528=CARTESIAN_POINT('Ctrl Pts',(-0.00210900663111077,-0.0230500960049795,
-0.0100422574299579));
#36529=CARTESIAN_POINT('Ctrl Pts',(-0.00212656154367453,-0.0230514170883795,
-0.0100597475728918));
#36530=CARTESIAN_POINT('Ctrl Pts',(-0.00213566749634862,-0.023052111507196,
-0.0100689380732353));
#36531=CARTESIAN_POINT('Ctrl Pts',(-0.00215840453463852,-0.0230538679299092,
-0.0100921850649516));
#36532=CARTESIAN_POINT('Ctrl Pts',(-0.00217195786982498,-0.0230549355470293,
-0.0101063165354204));
#36533=CARTESIAN_POINT('Ctrl Pts',(-0.00222623725557716,-0.0230592917244094,
-0.0101640317718339));
#36534=CARTESIAN_POINT('Ctrl Pts',(-0.002265795476054,-0.0230626528545809,
-0.010208690836643));
#36535=CARTESIAN_POINT('Ctrl Pts',(-0.00237467881292944,-0.0230723812373582,
-0.0103392582024945));
#36536=CARTESIAN_POINT('Ctrl Pts',(-0.00244062978192046,-0.0230788643175511,
-0.0104278529158088));
#36537=CARTESIAN_POINT('Ctrl Pts',(-0.00262023135593886,-0.0230979995435695,
-0.0106991619459459));
#36538=CARTESIAN_POINT('Ctrl Pts',(-0.00271931457749544,-0.0231105669534358,
-0.0108907140410943));
#36539=CARTESIAN_POINT('Ctrl Pts',(-0.00281319465099427,-0.0231248916448978,
-0.0111328169037544));
#36540=CARTESIAN_POINT('Ctrl Pts',(-0.00282839011552863,-0.0231273227423607,
-0.0111747545481903));
#36541=CARTESIAN_POINT('Ctrl Pts',(-0.00285079489111302,-0.0231310961601406,
-0.0112411776012326));
#36542=CARTESIAN_POINT('Ctrl Pts',(-0.00285863616818458,-0.0231324586926874,
-0.0112654415883313));
#36543=CARTESIAN_POINT('Ctrl Pts',(-0.0028726803670096,-0.0231349809984428,
-0.0113108713225446));
#36544=CARTESIAN_POINT('Ctrl Pts',(-0.00287896103140741,-0.0231361432051581,
-0.01133201105998));
#36545=CARTESIAN_POINT('Ctrl Pts',(-0.00289250933946686,-0.0231387305260738,
-0.0113795254374897));
#36546=CARTESIAN_POINT('Ctrl Pts',(-0.00289965051084627,-0.0231401515288994,
-0.0114059342641506));
#36547=CARTESIAN_POINT('Ctrl Pts',(-0.00292016100649074,-0.0231444174218248,
-0.0114861213218808));
#36548=CARTESIAN_POINT('Ctrl Pts',(-0.00293240287541535,-0.0231472269774604,
-0.0115401769976581));
#36549=CARTESIAN_POINT('Ctrl Pts',(-0.00297207236807625,-0.0231574592920736,
-0.0117410213835194));
#36550=CARTESIAN_POINT('Ctrl Pts',(-0.00299002971515789,-0.0231646059010671,
-0.0118894622990809));
#36551=CARTESIAN_POINT('Ctrl Pts',(-0.00300559583878791,-0.0231807522976641,
-0.0122294141504176));
#36552=CARTESIAN_POINT('Ctrl Pts',(-0.0029960925765037,-0.0231896718262875,
-0.0124205786570992));
#36553=CARTESIAN_POINT('Ctrl Pts',(-0.00296381075814312,-0.0232009555258161,
-0.0126415501064568));
#36554=CARTESIAN_POINT('Ctrl Pts',(-0.00295861376559142,-0.0232026118335257,
-0.0126734999185925));
#36555=CARTESIAN_POINT('Ctrl Pts',(-0.00295010556193767,-0.0232051167442208,
-0.0127209477958998));
#36556=CARTESIAN_POINT('Ctrl Pts',(-0.00294718672836175,-0.0232059458503163,
-0.0127365146975156));
#36557=CARTESIAN_POINT('Ctrl Pts',(-0.00294170977354681,-0.0232074506346619,
-0.0127644994811818));
#36558=CARTESIAN_POINT('Ctrl Pts',(-0.00293919589356769,-0.0232081239226253,
-0.0127769258528152));
#36559=CARTESIAN_POINT('Ctrl Pts',(-0.00293380447619497,-0.0232095334851328,
-0.0128027333555016));
#36560=CARTESIAN_POINT('Ctrl Pts',(-0.00293091403207324,-0.0232102704110402,
-0.0128161112402563));
#36561=CARTESIAN_POINT('Ctrl Pts',(-0.00292290124489559,-0.0232122635857939,
-0.0128520052848254));
#36562=CARTESIAN_POINT('Ctrl Pts',(-0.00291761039856934,-0.0232135286362112,
-0.0128744824515229));
#36563=CARTESIAN_POINT('Ctrl Pts',(-0.00288665617718246,-0.0232206506095388,
-0.0129994967135615));
#36564=CARTESIAN_POINT('Ctrl Pts',(-0.002855848825205,-0.0232267363709775,
-0.0131006755329025));
#36565=CARTESIAN_POINT('Ctrl Pts',(-0.00274638886205968,-0.023245452260209,
-0.0134020477730704));
#36566=CARTESIAN_POINT('Ctrl Pts',(-0.00265149540460457,-0.0232582410588757,
-0.013595639514043));
#36567=CARTESIAN_POINT('Ctrl Pts',(-0.00249270407568463,-0.0232751102625787,
-0.0138471475353924));
#36568=CARTESIAN_POINT('Ctrl Pts',(-0.00244582931164683,-0.0232796997731493,
-0.0139150251589628));
#36569=CARTESIAN_POINT('Ctrl Pts',(-0.00237667169176011,-0.0232859552279127,
-0.0140068329757861));
#36570=CARTESIAN_POINT('Ctrl Pts',(-0.00235670862254464,-0.0232877068922193,
-0.0140324575884491));
#36571=CARTESIAN_POINT('Ctrl Pts',(-0.00232219008759264,-0.0232906470566577,
-0.014075311496423));
#36572=CARTESIAN_POINT('Ctrl Pts',(-0.0023078496472254,-0.0232918438269465,
-0.0140927096549726));
#36573=CARTESIAN_POINT('Ctrl Pts',(-0.0022783432070652,-0.0232942574521064,
-0.0141276963843144));
#36574=CARTESIAN_POINT('Ctrl Pts',(-0.0022631663700046,-0.0232954737501677,
-0.0141452738280123));
#36575=CARTESIAN_POINT('Ctrl Pts',(-0.00222473302081043,-0.0232984929567715,
-0.0141887553493092));
#36576=CARTESIAN_POINT('Ctrl Pts',(-0.00220122658527684,-0.0233002854819867,
-0.0142144345031235));
#36577=CARTESIAN_POINT('Ctrl Pts',(-0.002100671207382,-0.0233077392388126,
-0.014320516539461));
#36578=CARTESIAN_POINT('Ctrl Pts',(-0.00201962073313046,-0.0233132304196038,
-0.0143970095609957));
#36579=CARTESIAN_POINT('Ctrl Pts',(-0.00173040184436039,-0.023331515734298,
-0.0146410133396785));
#36580=CARTESIAN_POINT('Ctrl Pts',(-0.00150425926905786,-0.023343617765556,
-0.0147851588788914));
#36581=CARTESIAN_POINT('Ctrl Pts',(-0.00123021960874593,-0.0233588937189667,
-0.0149122362854303));
#36582=CARTESIAN_POINT('Ctrl Pts',(-0.00119811876274534,-0.0233606935068962,
-0.0149264429384479));
#36583=CARTESIAN_POINT('Ctrl Pts',(-0.0011509620525543,-0.0233633625733339,
-0.0149463306618513));
#36584=CARTESIAN_POINT('Ctrl Pts',(-0.00113609705993683,-0.0233642075243567,
-0.0149524594849928));
#36585=CARTESIAN_POINT('Ctrl Pts',(-0.00110965097839164,-0.023365718308758,
-0.0149631152596545));
#36586=CARTESIAN_POINT('Ctrl Pts',(-0.00109808995778753,-0.0233663813511167,
-0.0149676901436489));
#36587=CARTESIAN_POINT('Ctrl Pts',(-0.00107228129811609,-0.0233678674723673,
-0.0149777179384334));
#36588=CARTESIAN_POINT('Ctrl Pts',(-0.00105802044053036,-0.0233686925440834,
-0.014983134077151));
#36589=CARTESIAN_POINT('Ctrl Pts',(-0.00101495229980725,-0.0233711946348244,
-0.0149991161721482));
#36590=CARTESIAN_POINT('Ctrl Pts',(-0.000986024379158144,-0.0233728890964912,
-0.0150093488791007));
#36591=CARTESIAN_POINT('Ctrl Pts',(-0.000838439061164374,-0.0233815858327414,
-0.0150590207443831));
#36592=CARTESIAN_POINT('Ctrl Pts',(-0.000717562990775569,-0.0233888727326024,
-0.0150914550096578));
#36593=CARTESIAN_POINT('Ctrl Pts',(-0.000361166688076326,-0.023410222604845,
-0.0151635762786417));
#36594=CARTESIAN_POINT('Ctrl Pts',(-0.000122455609657768,-0.0234242767349491,
-0.0151828397785596));
#36595=CARTESIAN_POINT('Ctrl Pts',(0.000161450816837787,-0.0234399626810071,
-0.0151718504981361));
#36596=CARTESIAN_POINT('Ctrl Pts',(0.000206822055415894,-0.0234424416457245,
-0.0151690606969192));
#36597=CARTESIAN_POINT('Ctrl Pts',(0.000277703535384509,-0.0234462721034308,
-0.0151630828091748));
#36598=CARTESIAN_POINT('Ctrl Pts',(0.000303264674181463,-0.0234476448191112,
-0.0151605961678332));
#36599=CARTESIAN_POINT('Ctrl Pts',(0.000350697010799507,-0.0234501767699155,
-0.0151553662167663));
#36600=CARTESIAN_POINT('Ctrl Pts',(0.000372575828300688,-0.0234513385904576,
-0.0151527095110721));
#36601=CARTESIAN_POINT('Ctrl Pts',(0.000421308516417335,-0.0234539136103442,
-0.0151462462969905));
#36602=CARTESIAN_POINT('Ctrl Pts',(0.00044814420473259,-0.0234553228859412,
-0.0151423162201934));
#36603=CARTESIAN_POINT('Ctrl Pts',(0.000528386912996602,-0.02345951315051,
-0.0151294509372252));
#36604=CARTESIAN_POINT('Ctrl Pts',(0.000581610301473264,-0.0234622607023705,
-0.0151194330323656));
#36605=CARTESIAN_POINT('Ctrl Pts',(0.000837974738500974,-0.0234753842930941,
-0.0150639537211611));
#36606=CARTESIAN_POINT('Ctrl Pts',(0.00103627788179657,-0.0234851475601321,
-0.0149988763968803));
#36607=CARTESIAN_POINT('Ctrl Pts',(0.00135539564432791,-0.0235017481233994,
-0.0148559512421176));
#36608=CARTESIAN_POINT('Ctrl Pts',(0.00148027065097291,-0.0235085161118657,
-0.0147890532592776));
#36609=CARTESIAN_POINT('Ctrl Pts',(0.00162617433732151,-0.0235172830420758,
-0.0146970669449115));
#36610=CARTESIAN_POINT('Ctrl Pts',(0.0016521427825219,-0.02351887898852,
-0.0146801267083532));
#36611=CARTESIAN_POINT('Ctrl Pts',(0.0016905404944525,-0.0235212996522941,
-0.014654221186381));
#36612=CARTESIAN_POINT('Ctrl Pts',(0.00170317188596976,-0.023522106005,
-0.0146455577460638));
#36613=CARTESIAN_POINT('Ctrl Pts',(0.00172593326819518,-0.0235235783755579,
-0.0146296888307665));
#36614=CARTESIAN_POINT('Ctrl Pts',(0.00173608558528243,-0.0235242422487976,
-0.0146225165962814));
#36615=CARTESIAN_POINT('Ctrl Pts',(0.00175920839760339,-0.0235257706797939,
-0.0146059648086507));
#36616=CARTESIAN_POINT('Ctrl Pts',(0.00177214860401666,-0.0235266378718645,
-0.0145965444065685));
#36617=CARTESIAN_POINT('Ctrl Pts',(0.00181289915774787,-0.0235294048528137,
-0.01456637634965));
#36618=CARTESIAN_POINT('Ctrl Pts',(0.00184042440863483,-0.0235313276398202,
-0.0145452501858211));
#36619=CARTESIAN_POINT('Ctrl Pts',(0.00190603417494513,-0.0235360301696671,
-0.0144930603624058));
#36620=CARTESIAN_POINT('Ctrl Pts',(0.00194373338347046,-0.0235388326101583,
-0.0144615293403826));
#36621=CARTESIAN_POINT('Ctrl Pts',(0.00209984895726982,-0.0235508134268864,
-0.0143243005631146));
#36622=CARTESIAN_POINT('Ctrl Pts',(0.00221055291113015,-0.0235602403810694,
-0.0142102196791277));
#36623=CARTESIAN_POINT('Ctrl Pts',(0.00241586060585624,-0.0235790709217195,
-0.0139619999471457));
#36624=CARTESIAN_POINT('Ctrl Pts',(0.00250955849766848,-0.0235884306850111,
-0.0138277705668581));
#36625=CARTESIAN_POINT('Ctrl Pts',(0.0026112132874205,-0.0235994932828823,
-0.0136533652060758));
#36626=CARTESIAN_POINT('Ctrl Pts',(0.00262992283256313,-0.0236015768083667,
-0.0136198000949265));
#36627=CARTESIAN_POINT('Ctrl Pts',(0.00265924540100263,-0.0236049230840802,
-0.0135647334372807));
#36628=CARTESIAN_POINT('Ctrl Pts',(0.00267025417425417,-0.0236061994817181,
-0.0135434485723585));
#36629=CARTESIAN_POINT('Ctrl Pts',(0.00269105157791277,-0.0236086512154649,
-0.0135020291719188));
#36630=CARTESIAN_POINT('Ctrl Pts',(0.00270087214529936,-0.0236098275931987,
-0.0134819125366312));
#36631=CARTESIAN_POINT('Ctrl Pts',(0.00272341720491548,-0.0236125739626949,
-0.0134343888080795));
#36632=CARTESIAN_POINT('Ctrl Pts',(0.00273595472551468,-0.0236141375477828,
-0.0134068954288716));
#36633=CARTESIAN_POINT('Ctrl Pts',(0.00277716940817561,-0.0236194092136078,
-0.013312775030068));
#36634=CARTESIAN_POINT('Ctrl Pts',(0.00280384580791125,-0.0236230514275926,
-0.0132452973815259));
#36635=CARTESIAN_POINT('Ctrl Pts',(0.00286483208484318,-0.0236320718617216,
-0.0130730080707523));
#36636=CARTESIAN_POINT('Ctrl Pts',(0.00289585963240274,-0.0236373595709136,
-0.012967148739534));
#36637=CARTESIAN_POINT('Ctrl Pts',(0.00295904284199911,-0.0236505339000564,
-0.0126973137287968));
#36638=CARTESIAN_POINT('Ctrl Pts',(0.00298346455402076,-0.0236583283326594,
-0.0125319272272697));
#36639=CARTESIAN_POINT('Ctrl Pts',(0.00299802975031829,-0.0236696710627736,
-0.0123018357096217));
#36640=CARTESIAN_POINT('Ctrl Pts',(0.00300002797117741,-0.0236728630743604,
-0.0122381840786));
#36641=CARTESIAN_POINT('Ctrl Pts',(0.00299999054361381,-0.0236772161196921,
-0.012153889558734));
#36642=CARTESIAN_POINT('Ctrl Pts',(0.00299976854987172,-0.0236782914898092,
-0.0121332590510467));
#36643=CARTESIAN_POINT('Ctrl Pts',(0.0029990839987087,-0.0236800023245391,
-0.012100782158435));
#36644=CARTESIAN_POINT('Ctrl Pts',(0.00299876397406545,-0.0236806302852637,
-0.0120889330707929));
#36645=CARTESIAN_POINT('Ctrl Pts',(0.00299794811527417,-0.0236819513424072,
-0.0120641651603841));
#36646=CARTESIAN_POINT('Ctrl Pts',(0.00299743898140654,-0.0236826452036303,
-0.012051247216751));
#36647=CARTESIAN_POINT('Ctrl Pts',(0.00299595105809359,-0.0236843983686079,
-0.0120188222698312));
#36648=CARTESIAN_POINT('Ctrl Pts',(0.00299486523419974,-0.0236854632440509,
-0.0119993209334478));
#36649=CARTESIAN_POINT('Ctrl Pts',(0.00298971982698869,-0.0236897925541175,
-0.0119207414896186));
#36650=CARTESIAN_POINT('Ctrl Pts',(0.00298410203585482,-0.0236931284826456,
-0.0118617818810736));
#36651=CARTESIAN_POINT('Ctrl Pts',(0.00296319571437003,-0.0237027522423811,
-0.0116948584774248));
#36652=CARTESIAN_POINT('Ctrl Pts',(0.00294376189222309,-0.0237091533609841,
-0.0115875091274863));
#36653=CARTESIAN_POINT('Ctrl Pts',(0.00286824243901585,-0.0237283406928037,
-0.0112701011097754));
#36654=CARTESIAN_POINT('Ctrl Pts',(0.00279513604605515,-0.0237410462846934,
-0.0110647988626298));
#36655=CARTESIAN_POINT('Ctrl Pts',(0.00268114283103387,-0.0237554813356063,
-0.0108292114109037));
#36656=CARTESIAN_POINT('Ctrl Pts',(0.00266091923460957,-0.0237579011737365,
-0.0107896785738794));
#36657=CARTESIAN_POINT('Ctrl Pts',(0.00262773162207752,-0.0237616611612863,
-0.01072820882834));
#36658=CARTESIAN_POINT('Ctrl Pts',(0.00261535359962061,-0.0237630212882156,
-0.0107059643253993));
#36659=CARTESIAN_POINT('Ctrl Pts',(0.00259172483963726,-0.0237655413444303,
-0.0106647448157392));
#36660=CARTESIAN_POINT('Ctrl Pts',(0.00258054511684337,-0.023766703671097,
-0.010645731268688));
#36661=CARTESIAN_POINT('Ctrl Pts',(0.00255500200828728,-0.0237692940416021,
-0.0106033660120561));
#36662=CARTESIAN_POINT('Ctrl Pts',(0.00254052608598711,-0.0237707179279876,
-0.0105800842676697));
#36663=CARTESIAN_POINT('Ctrl Pts',(0.00249566212445967,-0.0237750025528376,
-0.0105100874142737));
#36664=CARTESIAN_POINT('Ctrl Pts',(0.00246428904959614,-0.0237778274786264,
-0.0104640164515927));
#36665=CARTESIAN_POINT('Ctrl Pts',(0.00234518414384714,-0.0237879892610772,
-0.0102991787212611));
#36666=CARTESIAN_POINT('Ctrl Pts',(0.00224999924323684,-0.0237950582837991,
-0.0101860533123454));
#36667=CARTESIAN_POINT('Ctrl Pts',(0.00201505041911801,-0.0238110198580356,
-0.00994534071763116));
#36668=CARTESIAN_POINT('Ctrl Pts',(0.0018707964137518,-0.0238198329906898,
-0.00982304171108499));
#36669=CARTESIAN_POINT('Ctrl Pts',(0.00168470088398697,-0.0238312657018724,
-0.00969326558468347));
#36670=CARTESIAN_POINT('Ctrl Pts',(0.0016529595227852,-0.0238332185855835,
-0.00967201956001385));
#36671=CARTESIAN_POINT('Ctrl Pts',(0.00160698944913888,-0.0238360637387799,
-0.00964250468260526));
#36672=CARTESIAN_POINT('Ctrl Pts',(0.00159308379939658,-0.0238369265367141,
-0.0096337371950161));
#36673=CARTESIAN_POINT('Ctrl Pts',(0.00156849450791277,-0.0238384572597799,
-0.00961851467576912));
#36674=CARTESIAN_POINT('Ctrl Pts',(0.00155784156184011,-0.0238391221125371,
-0.00961201135410414));
#36675=CARTESIAN_POINT('Ctrl Pts',(0.00153449332920944,-0.0238405832890102,
-0.00959795717038656));
#36676=CARTESIAN_POINT('Ctrl Pts',(0.00152178287125252,-0.0238413811774976,
-0.00959043358412277));
#36677=CARTESIAN_POINT('Ctrl Pts',(0.00148460701276105,-0.0238437207580452,
-0.00956879752774689));
#36678=CARTESIAN_POINT('Ctrl Pts',(0.00145999782236882,-0.0238452768492956,
-0.0095549366611428));
#36679=CARTESIAN_POINT('Ctrl Pts',(0.00140246836106279,-0.0238489250415796,
-0.00952359545314692));
#36680=CARTESIAN_POINT('Ctrl Pts',(0.00136941097650588,-0.0238510291458285,
-0.00950637721680226));
#36681=CARTESIAN_POINT('Ctrl Pts',(0.00125063463585268,-0.0238585950199303,
-0.00944729831396889));
#36682=CARTESIAN_POINT('Ctrl Pts',(0.00116325269860505,-0.0238641699584645,
-0.00940891621795724));
#36683=CARTESIAN_POINT('Ctrl Pts',(0.00084795183712398,-0.02388400525069,
-0.00928800085618762));
#36684=CARTESIAN_POINT('Ctrl Pts',(0.00061198901376958,-0.0238982542268815,
-0.00922895333819541));
#36685=CARTESIAN_POINT('Ctrl Pts',(0.000329943583971665,-0.0239138851627141,
-0.00919375862347097));
#36686=CARTESIAN_POINT('Ctrl Pts',(0.000288311332469997,-0.023916160630979,
-0.00918944605319591));
#36687=CARTESIAN_POINT('Ctrl Pts',(0.000222008612282317,-0.0239197353439104,
-0.00918397744096975));
#36688=CARTESIAN_POINT('Ctrl Pts',(0.000197391669231275,-0.0239210518606808,
-0.00918225253203083));
#36689=CARTESIAN_POINT('Ctrl Pts',(0.000150622249964357,-0.0239235334687419,
-0.0091795548269802));
#36690=CARTESIAN_POINT('Ctrl Pts',(0.000128474914068545,-0.0239247002811825,
-0.00917852351614038));
#36691=CARTESIAN_POINT('Ctrl Pts',(7.76905004197529E-5,-0.0239273575422776,
-0.00917672262292262));
#36692=CARTESIAN_POINT('Ctrl Pts',(4.90495511143069E-5,-0.023928842852224,
-0.00917611750385087));
#36693=CARTESIAN_POINT('Ctrl Pts',(-4.22941296485705E-5,-0.0239335406998544,
-0.00917549624073787));
#36694=CARTESIAN_POINT('Ctrl Pts',(-0.000104992255973168,-0.0239367060219711,
-0.00917703543593957));
#36695=CARTESIAN_POINT('Ctrl Pts',(-0.000256299349197304,-0.0239442374556768,
-0.00918550163007713));
#36696=CARTESIAN_POINT('Ctrl Pts',(-0.000344738729613,-0.0239485494600936,
-0.00919440248335395));
#36697=CARTESIAN_POINT('Ctrl Pts',(-0.000545584499344328,-0.0239582763654799,
-0.00922367422563607));
#36698=CARTESIAN_POINT('Ctrl Pts',(-0.000657482488847247,-0.0239636465910073,
-0.00924656316237376));
#36699=CARTESIAN_POINT('Ctrl Pts',(-0.000907689727629172,-0.0239759500161392,
-0.00931280612047121));
#36700=CARTESIAN_POINT('Ctrl Pts',(-0.00104469968193725,-0.023982899584126,
-0.00935991046741799));
#36701=CARTESIAN_POINT('Ctrl Pts',(-0.00120015539018096,-0.0239915729879346,
-0.00942626787771243));
#36702=CARTESIAN_POINT('Ctrl Pts',(-0.00122243177870939,-0.0239928356952982,
-0.00943609903565198));
#36703=CARTESIAN_POINT('Ctrl Pts',(-0.00125728484333931,-0.0239948463244324,
-0.00945199028926844));
#36704=CARTESIAN_POINT('Ctrl Pts',(-0.00126994353020839,-0.0239955839457915,
-0.00945786906658127));
#36705=CARTESIAN_POINT('Ctrl Pts',(-0.0012940387654259,-0.0239970029115556,
-0.00946926412476303));
#36706=CARTESIAN_POINT('Ctrl Pts',(-0.00130548199015796,-0.023997683370686,
-0.00947476499309754));
#36707=CARTESIAN_POINT('Ctrl Pts',(-0.00133331782298868,-0.0239993541750954,
-0.00948836414554664));
#36708=CARTESIAN_POINT('Ctrl Pts',(-0.00134967185901501,-0.0240003490445426,
-0.00949653991557034));
#36709=CARTESIAN_POINT('Ctrl Pts',(-0.00140974375741294,-0.0240040496642591,
-0.00952726082024025));
#36710=CARTESIAN_POINT('Ctrl Pts',(-0.00145297804211985,-0.0240068040930066,
-0.00955072970891422));
#36711=CARTESIAN_POINT('Ctrl Pts',(-0.00156589836989284,-0.0240142045036448,
-0.00961567045438753));
#36712=CARTESIAN_POINT('Ctrl Pts',(-0.00163451259410128,-0.0240189152547235,
-0.00965892238592604));
#36713=CARTESIAN_POINT('Ctrl Pts',(-0.00191431720798182,-0.024038808655251,
-0.00985157174534062));
#36714=CARTESIAN_POINT('Ctrl Pts',(-0.00210752725721548,-0.0240541257260356,
-0.0100252101521695));
#36715=CARTESIAN_POINT('Ctrl Pts',(-0.00230480160209691,-0.0240708232947452,
-0.0102549590997473));
#36716=CARTESIAN_POINT('Ctrl Pts',(-0.00233279094855534,-0.0240732264113264,
-0.0102890486935559));
#36717=CARTESIAN_POINT('Ctrl Pts',(-0.00237569514221927,-0.0240769664440387,
-0.010343718659823));
#36718=CARTESIAN_POINT('Ctrl Pts',(-0.00239111682728279,-0.0240783229911736,
-0.0103638916227171));
#36719=CARTESIAN_POINT('Ctrl Pts',(-0.00241945611621449,-0.0240808397212438,
-0.0104019539595377));
#36720=CARTESIAN_POINT('Ctrl Pts',(-0.00243243598096626,-0.0240820022476223,
-0.0104197946446341));
#36721=CARTESIAN_POINT('Ctrl Pts',(-0.00246115110699001,-0.0240845972626595,
-0.0104601926151336));
#36722=CARTESIAN_POINT('Ctrl Pts',(-0.00247677546026185,-0.0240860255239846,
-0.0104828265013731));
#36723=CARTESIAN_POINT('Ctrl Pts',(-0.00252337724409488,-0.0240903386750709,
-0.0105523613026109));
#36724=CARTESIAN_POINT('Ctrl Pts',(-0.00255335063593726,-0.024093187017553,
-0.0105999218259456));
#36725=CARTESIAN_POINT('Ctrl Pts',(-0.00265436373082325,-0.0241030959488388,
-0.0107706606451979));
#36726=CARTESIAN_POINT('Ctrl Pts',(-0.00271796971260307,-0.0241099135746922,
-0.0108980199902509));
#36727=CARTESIAN_POINT('Ctrl Pts',(-0.00284122365024305,-0.024125227474835,
-0.0111960716815049));
#36728=CARTESIAN_POINT('Ctrl Pts',(-0.00289496780241338,-0.0241336481743369,
-0.0113685892165997));
#36729=CARTESIAN_POINT('Ctrl Pts',(-0.00294274324812855,-0.0241449837054204,
-0.0115906563681281));
#36730=CARTESIAN_POINT('Ctrl Pts',(-0.00295151940713886,-0.0241473593751018,
-0.0116366631436839));
#36731=CARTESIAN_POINT('Ctrl Pts',(-0.00296224567888654,-0.024150744668708,
-0.0117010473072671));
#36732=CARTESIAN_POINT('Ctrl Pts',(-0.00296510871728592,-0.0241517094162642,
-0.0117192676521714));
#36733=CARTESIAN_POINT('Ctrl Pts',(-0.00296964436012739,-0.0241533484297562,
-0.0117499764202617));
#36734=CARTESIAN_POINT('Ctrl Pts',(-0.00297140666992105,-0.024154017871949,
-0.0117624513874241));
#36735=CARTESIAN_POINT('Ctrl Pts',(-0.00297494112352456,-0.0241554325833925,
-0.0117886619789096));
#36736=CARTESIAN_POINT('Ctrl Pts',(-0.00297669680059275,-0.0241561786686898,
-0.0118023992207003));
#36737=CARTESIAN_POINT('Ctrl Pts',(-0.00298121629841019,-0.0241582227123249,
-0.0118398206155733));
#36738=CARTESIAN_POINT('Ctrl Pts',(-0.00298379290677064,-0.0241595302210376,
-0.0118635259052746));
#36739=CARTESIAN_POINT('Ctrl Pts',(-0.00299808405839939,-0.0241677545923681,
-0.0120113963404177));
#36740=CARTESIAN_POINT('Ctrl Pts',(-0.00300232786590801,-0.0241749883084336,
-0.0121361514787953));
#36741=CARTESIAN_POINT('Ctrl Pts',(-0.00299292543339883,-0.0241944537032271,
-0.0124680907328181));
#36742=CARTESIAN_POINT('Ctrl Pts',(-0.0029655741872156,-0.0242067291955422,
-0.0126742426040832));
#36743=CARTESIAN_POINT('Ctrl Pts',(-0.00290013222451379,-0.0242225432378703,
-0.0129469332675166));
#36744=CARTESIAN_POINT('Ctrl Pts',(-0.00288050612876583,-0.0242265899030205,
-0.0130172907045883));
#36745=CARTESIAN_POINT('Ctrl Pts',(-0.00284890094943722,-0.0242322433996795,
-0.0131164529252348));
#36746=CARTESIAN_POINT('Ctrl Pts',(-0.00283901196112395,-0.0242339155452147,
-0.013145892194538));
#36747=CARTESIAN_POINT('Ctrl Pts',(-0.00282116586804867,-0.0242367748349669,
-0.0131964072011758));
#36748=CARTESIAN_POINT('Ctrl Pts',(-0.0028134253392826,-0.0242379688864223,
-0.0132175562409481));
#36749=CARTESIAN_POINT('Ctrl Pts',(-0.00279706253746286,-0.0242404019626443,
-0.0132607502246054));
#36750=CARTESIAN_POINT('Ctrl Pts',(-0.00278841602177665,-0.0242416400889513,
-0.0132827843306514));
#36751=CARTESIAN_POINT('Ctrl Pts',(-0.00276558407820692,-0.0242447924676459,
-0.0133390017098491));
#36752=CARTESIAN_POINT('Ctrl Pts',(-0.00275102505997585,-0.0242466942548846,
-0.0133730294725887));
#36753=CARTESIAN_POINT('Ctrl Pts',(-0.00267794369588618,-0.0242557536201294,
-0.0135354590277854));
#36754=CARTESIAN_POINT('Ctrl Pts',(-0.0026110379929825,-0.0242626261821099,
-0.0136599005178529));
#36755=CARTESIAN_POINT('Ctrl Pts',(-0.00250833261636015,-0.0242718130524532,
-0.0138223263822906));
#36756=CARTESIAN_POINT('Ctrl Pts',(-0.00247995185372159,-0.0242742368375516,
-0.0138647715993533));
#36757=CARTESIAN_POINT('Ctrl Pts',(-0.00234010402643788,-0.0242857281933064,
-0.0140627916870461));
#36758=CARTESIAN_POINT('Ctrl Pts',(-0.0022150138999388,-0.0242946959407717,
-0.0142081724513265));
#36759=CARTESIAN_POINT('Ctrl Pts',(-0.00205648872608341,-0.0243058969783698,
-0.0143602658352723));
#36760=CARTESIAN_POINT('Ctrl Pts',(-0.00203575059417655,-0.0243073599010185,
-0.014379605421406));
#36761=CARTESIAN_POINT('Ctrl Pts',(-0.00200365119226635,-0.0243096262983495,
-0.0144087003412662));
#36762=CARTESIAN_POINT('Ctrl Pts',(-0.00199248535873276,-0.0243104150331364,
-0.0144186698520948));
#36763=CARTESIAN_POINT('Ctrl Pts',(-0.00197189184760518,-0.0243118713818575,
-0.0144367817930769));
#36764=CARTESIAN_POINT('Ctrl Pts',(-0.0019624874281233,-0.0243125371556687,
-0.0144449496371799));
#36765=CARTESIAN_POINT('Ctrl Pts',(-0.00194055137058768,-0.0243140915830116,
-0.014463762973664));
#36766=CARTESIAN_POINT('Ctrl Pts',(-0.00192798282004478,-0.0243149832360436,
-0.0144743642348176));
#36767=CARTESIAN_POINT('Ctrl Pts',(-0.00188671358988223,-0.0243179124919269,
-0.0145085971652751));
#36768=CARTESIAN_POINT('Ctrl Pts',(-0.00185766161182833,-0.0243199768675801,
-0.0145317979518989));
#36769=CARTESIAN_POINT('Ctrl Pts',(-0.00178533152702683,-0.024325106633711,
-0.0145873907489847));
#36770=CARTESIAN_POINT('Ctrl Pts',(-0.00174159517949529,-0.0243282000066036,
-0.0146191640112853));
#36771=CARTESIAN_POINT('Ctrl Pts',(-0.00153457327967907,-0.0243427208204296,
-0.0147611762112899));
#36772=CARTESIAN_POINT('Ctrl Pts',(-0.00136153691141119,-0.0243544782662629,
-0.0148563444089712));
#36773=CARTESIAN_POINT('Ctrl Pts',(-0.00106941452980384,-0.0243728244026265,
-0.0149813710614554));
#36774=CARTESIAN_POINT('Ctrl Pts',(-0.000955641409285482,-0.0243796447733796,
-0.0150221372015616));
#36775=CARTESIAN_POINT('Ctrl Pts',(-0.000804799545090952,-0.0243882358332565,
-0.0150661162531718));
#36776=CARTESIAN_POINT('Ctrl Pts',(-0.000769706148129626,-0.0243902042388357,
-0.0150756593020119));
#36777=CARTESIAN_POINT('Ctrl Pts',(-0.000711626713634182,-0.0243934133764966,
-0.0150903243157034));
#36778=CARTESIAN_POINT('Ctrl Pts',(-0.000688739153962839,-0.0243946657342736,
-0.0150958177349251));
#36779=CARTESIAN_POINT('Ctrl Pts',(-0.000643758820624876,-0.0243971036226168,
-0.0151060555057694));
#36780=CARTESIAN_POINT('Ctrl Pts',(-0.00062167245411589,-0.0243982897399379,
-0.0151108207244348));
#36781=CARTESIAN_POINT('Ctrl Pts',(-0.000568685450939444,-0.0244011101683298,
-0.0151216279003162));
#36782=CARTESIAN_POINT('Ctrl Pts',(-0.0005377391137935,-0.0244027370196843,
-0.0151274338730667));
#36783=CARTESIAN_POINT('Ctrl Pts',(-0.000426406157636438,-0.0244085219655865,
-0.0151465123483362));
#36784=CARTESIAN_POINT('Ctrl Pts',(-0.000345575280657453,-0.024412594585354,
-0.0151569967897483));
#36785=CARTESIAN_POINT('Ctrl Pts',(-0.000132199737694094,-0.0244231071782559,
-0.0151758766990228));
#36786=CARTESIAN_POINT('Ctrl Pts',(6.48715944714436E-7,-0.0244294078662443,
-0.0151787883733568));
#36787=CARTESIAN_POINT('Ctrl Pts',(0.000313364980468944,-0.0244442392018449,
-0.0151648841708013));
#36788=CARTESIAN_POINT('Ctrl Pts',(0.000492366994113262,-0.0244527253854847,
-0.0151406576085166));
#36789=CARTESIAN_POINT('Ctrl Pts',(0.000696430413059063,-0.0244633872474118,
-0.0150940427529168));
#36790=CARTESIAN_POINT('Ctrl Pts',(0.000724674107923275,-0.0244648858597611,
-0.0150871575305837));
#36791=CARTESIAN_POINT('Ctrl Pts',(0.000767447975458425,-0.0244671964531476,
-0.015076069175621));
#36792=CARTESIAN_POINT('Ctrl Pts',(0.000782054470761734,-0.0244679928051731,
-0.0150721646275349));
#36793=CARTESIAN_POINT('Ctrl Pts',(0.000808512061225958,-0.0244694496242428,
-0.0150648773652863));
#36794=CARTESIAN_POINT('Ctrl Pts',(0.000820372690964561,-0.0244701080362392,
-0.0150615318053742));
#36795=CARTESIAN_POINT('Ctrl Pts',(0.000847752412282308,-0.0244716402376234,
-0.0150536262920582));
#36796=CARTESIAN_POINT('Ctrl Pts',(0.000863255504750196,-0.0244725168827634,
-0.0150490138344148));
#36797=CARTESIAN_POINT('Ctrl Pts',(0.000912798500201012,-0.0244753457871115,
-0.0150338367041929));
#36798=CARTESIAN_POINT('Ctrl Pts',(0.000946686645037905,-0.024477322451287,
-0.0150227910267888));
#36799=CARTESIAN_POINT('Ctrl Pts',(0.00102855657802995,-0.0244821861649201,
-0.0149944825789868));
#36800=CARTESIAN_POINT('Ctrl Pts',(0.00107631003869392,-0.0244850978421941,
-0.0149765953247235));
#36801=CARTESIAN_POINT('Ctrl Pts',(0.0012829169667477,-0.0244979589918213,
-0.0148931412285657));
#36802=CARTESIAN_POINT('Ctrl Pts',(0.00143642617006764,-0.0245081856067871,
-0.0148152112498838));
#36803=CARTESIAN_POINT('Ctrl Pts',(0.0017083842645252,-0.0245268305120799,
-0.0146463606072049));
#36804=CARTESIAN_POINT('Ctrl Pts',(0.00182838862450916,-0.0245352819933739,
-0.0145589159267533));
#36805=CARTESIAN_POINT('Ctrl Pts',(0.00197026495764921,-0.0245454736888598,
-0.0144384811783818));
#36806=CARTESIAN_POINT('Ctrl Pts',(0.00199861960093413,-0.0245475224839742,
-0.0144134745342386));
#36807=CARTESIAN_POINT('Ctrl Pts',(0.00204406848245994,-0.0245508273779867,
-0.0143718387259144));
#36808=CARTESIAN_POINT('Ctrl Pts',(0.00206144986247046,-0.0245520965025603,
-0.0143555304460652));
#36809=CARTESIAN_POINT('Ctrl Pts',(0.00209481577950532,-0.0245545436449413,
-0.0143234683354241));
#36810=CARTESIAN_POINT('Ctrl Pts',(0.002110821474379,-0.024555722571682,
-0.0143077389044522));
#36811=CARTESIAN_POINT('Ctrl Pts',(0.00214820825818189,-0.0245584892800598,
-0.0142701635648651));
#36812=CARTESIAN_POINT('Ctrl Pts',(0.00216943512202904,-0.0245600703666536,
-0.0142481673558518));
#36813=CARTESIAN_POINT('Ctrl Pts',(0.00224150834893708,-0.0245654790661008,
-0.014171160590113));
#36814=CARTESIAN_POINT('Ctrl Pts',(0.00229062997381936,-0.0245692358539022,
-0.014114570992703));
#36815=CARTESIAN_POINT('Ctrl Pts',(0.00241021144939596,-0.0245786375309269,
-0.0139659111973718));
#36816=CARTESIAN_POINT('Ctrl Pts',(0.0024775492219414,-0.0245841806875644,
-0.0138714884090777));
#36817=CARTESIAN_POINT('Ctrl Pts',(0.00263600350410661,-0.0245983073758991,
-0.0136196301003421));
#36818=CARTESIAN_POINT('Ctrl Pts',(0.00271857249125541,-0.0246067903875411,
-0.0134573988988336));
#36819=CARTESIAN_POINT('Ctrl Pts',(0.00280275794494099,-0.0246181328691637,
-0.0132466472515459));
#36820=CARTESIAN_POINT('Ctrl Pts',(0.00281860531429751,-0.0246204334452691,
-0.013204209011279));
#36821=CARTESIAN_POINT('Ctrl Pts',(0.00283946248174454,-0.0246237279465049,
-0.0131442456962797));
#36822=CARTESIAN_POINT('Ctrl Pts',(0.0028452832819412,-0.0246246800712975,
-0.0131270073529358));
#36823=CARTESIAN_POINT('Ctrl Pts',(0.00285489446407619,-0.0246263108298569,
-0.01309766586315));
#36824=CARTESIAN_POINT('Ctrl Pts',(0.00285876564042425,-0.0246269849350396,
-0.0130855894230883));
#36825=CARTESIAN_POINT('Ctrl Pts',(0.00286674740120017,-0.0246284124479961,
-0.0130601355816776));
#36826=CARTESIAN_POINT('Ctrl Pts',(0.00287084108572552,-0.0246291667128416,
-0.0130467535590475));
#36827=CARTESIAN_POINT('Ctrl Pts',(0.00288185008939962,-0.024631256446154,
-0.0130098445332519));
#36828=CARTESIAN_POINT('Ctrl Pts',(0.0028885706605584,-0.0246326021584463,
-0.0129862610852846));
#36829=CARTESIAN_POINT('Ctrl Pts',(0.00293680454295546,-0.0246427942332822,
-0.0128087739990707));
#36830=CARTESIAN_POINT('Ctrl Pts',(0.00296627808353792,-0.0246521521782912,
-0.0126518741132068));
#36831=CARTESIAN_POINT('Ctrl Pts',(0.00299434044326856,-0.0246677440425888,
-0.0123882387308766));
#36832=CARTESIAN_POINT('Ctrl Pts',(0.00299996571188081,-0.0246739614871394,
-0.0122825746941183));
#36833=CARTESIAN_POINT('Ctrl Pts',(0.00299999984374834,-0.0246800791551026,
-0.0121768215375357));
#36834=CARTESIAN_POINT('',(0.00299999999556417,-0.0266759885990988,-0.0121756901455692));
#36835=CARTESIAN_POINT('Ctrl Pts',(0.00299999984374834,-0.0246800791551026,
-0.0121768215375361));
#36836=CARTESIAN_POINT('Ctrl Pts',(0.0030000271394786,-0.0246849715394514,
-0.0120922492640467));
#36837=CARTESIAN_POINT('Ctrl Pts',(0.00299647877875121,-0.0246897951466881,
-0.012007719316541));
#36838=CARTESIAN_POINT('Ctrl Pts',(0.0029851797271477,-0.0246973003957579,
-0.0118739046611527));
#36839=CARTESIAN_POINT('Ctrl Pts',(0.00297976667861642,-0.0247000442136567,
-0.011824481818541));
#36840=CARTESIAN_POINT('Ctrl Pts',(0.00296977267758926,-0.0247041191505159,
-0.0117503166974606));
#36841=CARTESIAN_POINT('Ctrl Pts',(0.00296610496658861,-0.0247054775876757,
-0.0117254617630247));
#36842=CARTESIAN_POINT('Ctrl Pts',(0.00295883097818313,-0.0247079429921856,
-0.0116801196810558));
#36843=CARTESIAN_POINT('Ctrl Pts',(0.00295532304068977,-0.024709052922994,
-0.0116596185340017));
#36844=CARTESIAN_POINT('Ctrl Pts',(0.00294765741526115,-0.024711325890459,
-0.0116174609867613));
#36845=CARTESIAN_POINT('Ctrl Pts',(0.00294347357689748,-0.0247124880340499,
-0.0115958105855758));
#36846=CARTESIAN_POINT('Ctrl Pts',(0.00293357193311885,-0.0247150736036087,
-0.0115474408326705));
#36847=CARTESIAN_POINT('Ctrl Pts',(0.00292772699980406,-0.024716492944789,
-0.0115207493426016));
#36848=CARTESIAN_POINT('Ctrl Pts',(0.00290938173190182,-0.0247206540978431,
-0.0114421296362844));
#36849=CARTESIAN_POINT('Ctrl Pts',(0.0028958581845863,-0.0247233638757336,
-0.0113904500371739));
#36850=CARTESIAN_POINT('Ctrl Pts',(0.00282939955094125,-0.0247352869549178,
-0.0111616157966445));
#36851=CARTESIAN_POINT('Ctrl Pts',(0.00276153367853952,-0.0247440349531215,
-0.010989212134275));
#36852=CARTESIAN_POINT('Ctrl Pts',(0.0026286760278695,-0.0247580065665102,
-0.0107259716925797));
#36853=CARTESIAN_POINT('Ctrl Pts',(0.00257376619301133,-0.0247632194913892,
-0.010630596062701));
#36854=CARTESIAN_POINT('Ctrl Pts',(0.00248691976406342,-0.0247710047313163,
-0.0104972687386255));
#36855=CARTESIAN_POINT('Ctrl Pts',(0.0024590851232924,-0.0247734423320927,
-0.0104567500457898));
#36856=CARTESIAN_POINT('Ctrl Pts',(0.0024099226142933,-0.0247776847851966,
-0.0103888229955561));
#36857=CARTESIAN_POINT('Ctrl Pts',(0.00238909084963975,-0.0247794647123323,
-0.0103610670769178));
#36858=CARTESIAN_POINT('Ctrl Pts',(0.00235795385591366,-0.0247821096638489,
-0.0103210460613349));
#36859=CARTESIAN_POINT('Ctrl Pts',(0.00234802378661415,-0.0247829509765828,
-0.010308491376139));
#36860=CARTESIAN_POINT('Ctrl Pts',(0.00233020467891303,-0.0247844579850185,
-0.0102863293576096));
#36861=CARTESIAN_POINT('Ctrl Pts',(0.00232235570566486,-0.0247851209498248,
-0.0102766907102858));
#36862=CARTESIAN_POINT('Ctrl Pts',(0.0023047019852878,-0.0247866103758972,
-0.0102552847922193));
#36863=CARTESIAN_POINT('Ctrl Pts',(0.00229486697647337,-0.0247874388831487,
-0.010243543755816));
#36864=CARTESIAN_POINT('Ctrl Pts',(0.00226485497803572,-0.0247899619563692,
-0.0102082677285596));
#36865=CARTESIAN_POINT('Ctrl Pts',(0.00224440323299895,-0.0247916743780112,
-0.010184970321547));
#36866=CARTESIAN_POINT('Ctrl Pts',(0.00212660959357736,-0.0248014779133856,
-0.010054908868805));
#36867=CARTESIAN_POINT('Ctrl Pts',(0.00202202184638895,-0.0248099496334261,
-0.00995497613217003));
#36868=CARTESIAN_POINT('Ctrl Pts',(0.00179053011871227,-0.0248276059760619,
-0.00976374259653401));
#36869=CARTESIAN_POINT('Ctrl Pts',(0.0016628516632203,-0.0248367629338216,
-0.00967401252558521));
#36870=CARTESIAN_POINT('Ctrl Pts',(0.00147681606898583,-0.0248490611889767,
-0.0095638309311238));
#36871=CARTESIAN_POINT('Ctrl Pts',(0.00142393942697235,-0.0248524514176395,
-0.00953463317930624));
#36872=CARTESIAN_POINT('Ctrl Pts',(0.00132809846362635,-0.0248584065537394,
-0.00948542658340009));
#36873=CARTESIAN_POINT('Ctrl Pts',(0.00128547449483161,-0.0248609907740733,
-0.0094648023754128));
#36874=CARTESIAN_POINT('Ctrl Pts',(0.00121889485155252,-0.0248649306120928,
-0.00943451037098353));
#36875=CARTESIAN_POINT('Ctrl Pts',(0.00119527386442428,-0.0248663100176773,
-0.00942412908429987));
#36876=CARTESIAN_POINT('Ctrl Pts',(0.0011512390915213,-0.024868848404098,
-0.0094054500766122));
#36877=CARTESIAN_POINT('Ctrl Pts',(0.00113086229457634,-0.0248700100693831,
-0.00939707011818949));
#36878=CARTESIAN_POINT('Ctrl Pts',(0.00108533696072991,-0.0248725775034092,
-0.00937893154217753));
#36879=CARTESIAN_POINT('Ctrl Pts',(0.00106014525041828,-0.024873979465628,
-0.00936928604667271));
#36880=CARTESIAN_POINT('Ctrl Pts',(0.000995629909773804,-0.0248775244149862,
-0.00934557680984292));
#36881=CARTESIAN_POINT('Ctrl Pts',(0.000956135904486478,-0.0248796519266907,
-0.00933199179282939));
#36882=CARTESIAN_POINT('Ctrl Pts',(0.000737537006826487,-0.0248912171752032,
-0.00926186780337004));
#36883=CARTESIAN_POINT('Ctrl Pts',(0.000553702147464557,-0.0249001400695489,
-0.00922141704469027));
#36884=CARTESIAN_POINT('Ctrl Pts',(0.00023952789727079,-0.0249151378517388,
-0.00918266150627814));
#36885=CARTESIAN_POINT('Ctrl Pts',(0.000110893656095513,-0.0249212202540674,
-0.00917514171568758));
#36886=CARTESIAN_POINT('Ctrl Pts',(-8.29382840763949E-5,-0.0249307537628703,
-0.00917629298347272));
#36887=CARTESIAN_POINT('Ctrl Pts',(-0.000148024479865065,-0.0249340186355012,
-0.00917879999159463));
#36888=CARTESIAN_POINT('Ctrl Pts',(-0.000233088028873369,-0.0249384263639998,
-0.00918485401746374));
#36889=CARTESIAN_POINT('Ctrl Pts',(-0.000253187415226254,-0.0249394781938473,
-0.0091864883461244));
#36890=CARTESIAN_POINT('Ctrl Pts',(-0.000286270943035285,-0.0249412287383808,
-0.00918951448605934));
#36891=CARTESIAN_POINT('Ctrl Pts',(-0.000299265543948449,-0.0249419212212067,
-0.00919078869602892));
#36892=CARTESIAN_POINT('Ctrl Pts',(-0.000323916940709067,-0.024943244883031,
-0.00919336851806675));
#36893=CARTESIAN_POINT('Ctrl Pts',(-0.000335575173114158,-0.0249438751025326,
-0.00919465774238381));
#36894=CARTESIAN_POINT('Ctrl Pts',(-0.000367067573682288,-0.0249455883960714,
-0.00919832739141528));
#36895=CARTESIAN_POINT('Ctrl Pts',(-0.000386885689650826,-0.0249466782517823,
-0.00920083757560438));
#36896=CARTESIAN_POINT('Ctrl Pts',(-0.000464085223446902,-0.0249509654014279,
-0.00921140016014898));
#36897=CARTESIAN_POINT('Ctrl Pts',(-0.000521250793847492,-0.0249542299593569,
-0.00922091602249985));
#36898=CARTESIAN_POINT('Ctrl Pts',(-0.000746175468686555,-0.0249673407682444,
-0.00926508697398773));
#36899=CARTESIAN_POINT('Ctrl Pts',(-0.000911109901030542,-0.0249775256807038,
-0.00931242607945585));
#36900=CARTESIAN_POINT('Ctrl Pts',(-0.00120113197068892,-0.0249956896467627,
-0.00942327987439296));
#36901=CARTESIAN_POINT('Ctrl Pts',(-0.00132755693874223,-0.0250037066676969,
-0.00948197542543346));
#36902=CARTESIAN_POINT('Ctrl Pts',(-0.00149728314555392,-0.0250144876078641,
-0.00957563659779584));
#36903=CARTESIAN_POINT('Ctrl Pts',(-0.0015443795621772,-0.0250174827904314,
-0.00960333002301077));
#36904=CARTESIAN_POINT('Ctrl Pts',(-0.00161376505350052,-0.0250219021941725,
-0.00964672246954577));
#36905=CARTESIAN_POINT('Ctrl Pts',(-0.00163663754514,-0.025023360206945,
-0.00966146311208925));
#36906=CARTESIAN_POINT('Ctrl Pts',(-0.00167767133834964,-0.0250259788418739,
-0.00968870536516019));
#36907=CARTESIAN_POINT('Ctrl Pts',(-0.0016959011985513,-0.0250271432827949,
-0.00970109975096745));
#36908=CARTESIAN_POINT('Ctrl Pts',(-0.00173501163478727,-0.025029644528405,
-0.00972832586253106));
#36909=CARTESIAN_POINT('Ctrl Pts',(-0.00175584232463214,-0.0250309786359784,
-0.00974322638376825));
#36910=CARTESIAN_POINT('Ctrl Pts',(-0.00181283907661768,-0.0250346361936943,
-0.00978511065343833));
#36911=CARTESIAN_POINT('Ctrl Pts',(-0.0018485917528818,-0.0250369385512274,
-0.00981264685138758));
#36912=CARTESIAN_POINT('Ctrl Pts',(-0.00204550391388021,-0.0250496925744515,
-0.00997151011495595));
#36913=CARTESIAN_POINT('Ctrl Pts',(-0.00219329210781418,-0.025059497600809,
-0.0101185024539239));
#36914=CARTESIAN_POINT('Ctrl Pts',(-0.00239729318432934,-0.0250747972721603,
-0.0103685972404435));
#36915=CARTESIAN_POINT('Ctrl Pts',(-0.00246471021951447,-0.0250802559978145,
-0.0104616800527805));
#36916=CARTESIAN_POINT('Ctrl Pts',(-0.0025595396148326,-0.025088933298469,
-0.0106098122484654));
#36917=CARTESIAN_POINT('Ctrl Pts',(-0.00259087771523434,-0.0250920023462928,
-0.0106622221109417));
#36918=CARTESIAN_POINT('Ctrl Pts',(-0.00263020017016898,-0.0250961811488614,
-0.0107327882904812));
#36919=CARTESIAN_POINT('Ctrl Pts',(-0.0026396365257818,-0.0250972112688108,
-0.0107501224249636));
#36920=CARTESIAN_POINT('Ctrl Pts',(-0.00265498900491641,-0.0250989353644997,
-0.0107789991146032));
#36921=CARTESIAN_POINT('Ctrl Pts',(-0.00266100270413413,-0.025099623489405,
-0.0107904895090416));
#36922=CARTESIAN_POINT('Ctrl Pts',(-0.00267235047423996,-0.0251009473524312,
-0.010812518241925));
#36923=CARTESIAN_POINT('Ctrl Pts',(-0.00267769714287106,-0.0251015822329976,
-0.0108230497152173));
#36924=CARTESIAN_POINT('Ctrl Pts',(-0.00269211290247009,-0.0251033241283995,
-0.0108518651181595));
#36925=CARTESIAN_POINT('Ctrl Pts',(-0.00270105766485107,-0.0251044383085421,
-0.0108702101517136));
#36926=CARTESIAN_POINT('Ctrl Pts',(-0.0027362554494885,-0.0251089552167848,
-0.0109443080465254));
#36927=CARTESIAN_POINT('Ctrl Pts',(-0.00276097360798209,-0.0251124342920514,
-0.0110007697374631));
#36928=CARTESIAN_POINT('Ctrl Pts',(-0.00285445578057964,-0.0251268160190748,
-0.0112335697435483));
#36929=CARTESIAN_POINT('Ctrl Pts',(-0.00290820053023947,-0.0251381068496403,
-0.0114154675499832));
#36930=CARTESIAN_POINT('Ctrl Pts',(-0.00296704862807839,-0.0251559913789531,
-0.0117170064762106));
#36931=CARTESIAN_POINT('Ctrl Pts',(-0.00298279797073649,-0.0251627449453282,
-0.0118340366376069));
#36932=CARTESIAN_POINT('Ctrl Pts',(-0.00299563347764602,-0.0251722923041128,
-0.0120053428824403));
#36933=CARTESIAN_POINT('Ctrl Pts',(-0.00299820942203873,-0.0251752405590099,
-0.0120590864430118));
#36934=CARTESIAN_POINT('Ctrl Pts',(-0.00299990679639111,-0.0251796056149532,
-0.0121399208547089));
#36935=CARTESIAN_POINT('Ctrl Pts',(-0.00300010886243288,-0.0251810549876021,
-0.0121669760527427));
#36936=CARTESIAN_POINT('Ctrl Pts',(-0.00299981141119672,-0.0251836644797591,
-0.0122160659536202));
#36937=CARTESIAN_POINT('Ctrl Pts',(-0.00299943511963678,-0.0251848282947188,
-0.0122380992431623));
#36938=CARTESIAN_POINT('Ctrl Pts',(-0.00299809319768953,-0.0251873351886208,
-0.0122858506354184));
#36939=CARTESIAN_POINT('Ctrl Pts',(-0.00299703932724928,-0.0251886754672274,
-0.0123115646102796));
#36940=CARTESIAN_POINT('Ctrl Pts',(-0.00299319585616863,-0.0251923685214541,
-0.0123828970990189));
#36941=CARTESIAN_POINT('Ctrl Pts',(-0.0029896944846547,-0.0251946995049771,
-0.0124284710620837));
#36942=CARTESIAN_POINT('Ctrl Pts',(-0.00296606136054852,-0.0252066824336097,
-0.0126651350908047));
#36943=CARTESIAN_POINT('Ctrl Pts',(-0.00292864567160056,-0.0252157967230421,
-0.0128540558199733));
#36944=CARTESIAN_POINT('Ctrl Pts',(-0.00283730973855783,-0.025230852476253,
-0.0131584290691307));
#36945=CARTESIAN_POINT('Ctrl Pts',(-0.00279368240071036,-0.0252367958495722,
-0.0132763609846854));
#36946=CARTESIAN_POINT('Ctrl Pts',(-0.00272512555053885,-0.0252451244149487,
-0.0134310795476146));
#36947=CARTESIAN_POINT('Ctrl Pts',(-0.00270658974067497,-0.0252472991516676,
-0.0134705632583707));
#36948=CARTESIAN_POINT('Ctrl Pts',(-0.00267307302553228,-0.0252511271985513,
-0.0135380905444445));
#36949=CARTESIAN_POINT('Ctrl Pts',(-0.00265849464954566,-0.0252527616163077,
-0.0135663265130125));
#36950=CARTESIAN_POINT('Ctrl Pts',(-0.00263615882656397,-0.0252552293160507,
-0.0136079516805647));
#36951=CARTESIAN_POINT('Ctrl Pts',(-0.0026287414569832,-0.0252560431686659,
-0.0136215218173752));
#36952=CARTESIAN_POINT('Ctrl Pts',(-0.00261577632345885,-0.0252574572020928,
-0.013644811920748));
#36953=CARTESIAN_POINT('Ctrl Pts',(-0.00261027858707579,-0.0252580543004693,
-0.0136545591172496));
#36954=CARTESIAN_POINT('Ctrl Pts',(-0.00259718858612093,-0.0252594702163244,
-0.0136774665084357));
#36955=CARTESIAN_POINT('Ctrl Pts',(-0.00258955090250267,-0.0252602918072985,
-0.0136905997748071));
#36956=CARTESIAN_POINT('Ctrl Pts',(-0.00256634944299513,-0.0252627727798938,
-0.0137298071533415));
#36957=CARTESIAN_POINT('Ctrl Pts',(-0.00255048961236525,-0.0252644491935699,
-0.0137557028623684));
#36958=CARTESIAN_POINT('Ctrl Pts',(-0.00241664039323987,-0.025278412240182,
-0.0139669805002835));
#36959=CARTESIAN_POINT('Ctrl Pts',(-0.00227900709992473,-0.0252915671254282,
-0.0141391181993388));
#36960=CARTESIAN_POINT('Ctrl Pts',(-0.00204875484969811,-0.0253106048893962,
-0.0143699130791668));
#36961=CARTESIAN_POINT('Ctrl Pts',(-0.00196974481189574,-0.0253167325711406,
-0.014441113337618));
#36962=CARTESIAN_POINT('Ctrl Pts',(-0.00183206378602863,-0.0253266972549476,
-0.0145525227457129));
#36963=CARTESIAN_POINT('Ctrl Pts',(-0.00177544746967256,-0.0253306141489884,
-0.0145951099585081));
#36964=CARTESIAN_POINT('Ctrl Pts',(-0.00169281252376824,-0.0253360802372307,
-0.0146528036382158));
#36965=CARTESIAN_POINT('Ctrl Pts',(-0.00166799560278297,-0.02533769119215,
-0.0146695830318676));
#36966=CARTESIAN_POINT('Ctrl Pts',(-0.00162423459617831,-0.0253404798241438,
-0.0146982254388942));
#36967=CARTESIAN_POINT('Ctrl Pts',(-0.00160540182590532,-0.0253416635086042,
-0.0147102534743738));
#36968=CARTESIAN_POINT('Ctrl Pts',(-0.00156601260719648,-0.0253441060270273,
-0.014734795168874));
#36969=CARTESIAN_POINT('Ctrl Pts',(-0.00154543640099061,-0.0253453635517764,
-0.0147472741812628));
#36970=CARTESIAN_POINT('Ctrl Pts',(-0.00149120137962799,-0.0253486317232652,
-0.0147792803514276));
#36971=CARTESIAN_POINT('Ctrl Pts',(-0.00145730840968821,-0.0253506279964612,
-0.0147984028880236));
#36972=CARTESIAN_POINT('Ctrl Pts',(-0.00127480414179758,-0.0253611501840864,
-0.0148967415019382));
#36973=CARTESIAN_POINT('Ctrl Pts',(-0.00112008471889298,-0.0253692578100808,
-0.0149640024830146));
#36974=CARTESIAN_POINT('Ctrl Pts',(-0.000840686702085648,-0.0253832675895954,
-0.0150584300265544));
#36975=CARTESIAN_POINT('Ctrl Pts',(-0.000718405481583358,-0.0253892092954031,
-0.0150913111756311));
#36976=CARTESIAN_POINT('Ctrl Pts',(-0.000500752380560026,-0.0253999333296747,
-0.0151353091091413));
#36977=CARTESIAN_POINT('Ctrl Pts',(-0.000406242947278311,-0.0254046394816158,
-0.0151497556815451));
#36978=CARTESIAN_POINT('Ctrl Pts',(-0.000288784314962083,-0.02541071732613,
-0.0151620066938834));
#36979=CARTESIAN_POINT('Ctrl Pts',(-0.000266329848170264,-0.0254118895287571,
-0.0151640930537761));
#36980=CARTESIAN_POINT('Ctrl Pts',(-0.000230329878603105,-0.0254137883119842,
-0.0151670290224538));
#36981=CARTESIAN_POINT('Ctrl Pts',(-0.000216798042904016,-0.0254145064304734,
-0.0151680402343232));
#36982=CARTESIAN_POINT('Ctrl Pts',(-0.00019054441623753,-0.0254159089827382,
-0.0151698231025514));
#36983=CARTESIAN_POINT('Ctrl Pts',(-0.000177823794222554,-0.0254165928379668,
-0.0151706055488515));
#36984=CARTESIAN_POINT('Ctrl Pts',(-0.000145879985982581,-0.0254183202401005,
-0.015172366179774));
#36985=CARTESIAN_POINT('Ctrl Pts',(-0.000126651793888489,-0.0254193692054502,
-0.0151732404444429));
#36986=CARTESIAN_POINT('Ctrl Pts',(-5.51238562221319E-5,-0.025423302080105,
-0.0151758031939177));
#36987=CARTESIAN_POINT('Ctrl Pts',(-2.7934491336597E-6,-0.0254262404455392,
-0.0151763081965697));
#36988=CARTESIAN_POINT('Ctrl Pts',(0.000225262751348615,-0.0254392370628772,
-0.0151725432159265));
#36989=CARTESIAN_POINT('Ctrl Pts',(0.000400404943875442,-0.0254496910328864,
-0.0151542030397294));
#36990=CARTESIAN_POINT('Ctrl Pts',(0.000684481379551118,-0.02546663004315,
-0.0150989338718602));
#36991=CARTESIAN_POINT('Ctrl Pts',(0.000794716739886117,-0.0254732041795396,
-0.0150709083107126));
#36992=CARTESIAN_POINT('Ctrl Pts',(0.00097365225308281,-0.0254837826188235,
-0.0150144223723092));
#36993=CARTESIAN_POINT('Ctrl Pts',(0.00104335707163828,-0.0254878805338421,
-0.014989548448926));
#36994=CARTESIAN_POINT('Ctrl Pts',(0.00114033744010028,-0.0254935477396581,
-0.0149508409471969));
#36995=CARTESIAN_POINT('Ctrl Pts',(0.00116842702581515,-0.0254951851776466,
-0.0149391311176765));
#36996=CARTESIAN_POINT('Ctrl Pts',(0.00121689288194461,-0.0254980042721968,
-0.0149180557390365));
#36997=CARTESIAN_POINT('Ctrl Pts',(0.0012373509575093,-0.0254991923230563,
-0.0149088855258758));
#36998=CARTESIAN_POINT('Ctrl Pts',(0.00127938618555014,-0.0255016300766138,
-0.0148894747255589));
#36999=CARTESIAN_POINT('Ctrl Pts',(0.00130094773824838,-0.0255028786547219,
-0.0148792040502657));
#37000=CARTESIAN_POINT('Ctrl Pts',(0.00135652620999398,-0.0255060935888792,
-0.0148519107188751));
#37001=CARTESIAN_POINT('Ctrl Pts',(0.00139034660701288,-0.025508046460882,
-0.0148344964023408));
#37002=CARTESIAN_POINT('Ctrl Pts',(0.00155381147988048,-0.0255174815104599,
-0.0147463548017938));
#37003=CARTESIAN_POINT('Ctrl Pts',(0.0016784503875721,-0.025524650410476,
-0.0146667604106928));
#37004=CARTESIAN_POINT('Ctrl Pts',(0.00193442859958337,-0.0255398989783619,
-0.0144753212762969));
#37005=CARTESIAN_POINT('Ctrl Pts',(0.00206301358235341,-0.0255479049119119,
-0.0143606957851303));
#37006=CARTESIAN_POINT('Ctrl Pts',(0.00221608468519604,-0.0255587930129314,
-0.0141986161868936));
#37007=CARTESIAN_POINT('Ctrl Pts',(0.00225014989421621,-0.0255613179393576,
-0.0141606520412306));
#37008=CARTESIAN_POINT('Ctrl Pts',(0.00230635314405614,-0.0255656968316467,
-0.0140947086696502));
#37009=CARTESIAN_POINT('Ctrl Pts',(0.00232899052884989,-0.0255675236849599,
-0.0140671686263753));
#37010=CARTESIAN_POINT('Ctrl Pts',(0.00236117831096757,-0.0255702255922654,
-0.0140265554917247));
#37011=CARTESIAN_POINT('Ctrl Pts',(0.00237112283675339,-0.0255710754680737,
-0.0140137972841784));
#37012=CARTESIAN_POINT('Ctrl Pts',(0.00238846137611719,-0.0255725853559766,
-0.0139911780923155));
#37013=CARTESIAN_POINT('Ctrl Pts',(0.00239589852966817,-0.0255732424178969,
-0.0139813510361035));
#37014=CARTESIAN_POINT('Ctrl Pts',(0.00241232522660593,-0.0255747150410371,
-0.0139593654460252));
#37015=CARTESIAN_POINT('Ctrl Pts',(0.00242128343066518,-0.0255755325605873,
-0.0139471847492884));
#37016=CARTESIAN_POINT('Ctrl Pts',(0.00244719459557312,-0.025577938527509,
-0.0139113888480944));
#37017=CARTESIAN_POINT('Ctrl Pts',(0.00246389642761711,-0.0255795421838436,
-0.0138875948983747));
#37018=CARTESIAN_POINT('Ctrl Pts',(0.00258167008182509,-0.0255912167304728,
-0.0137145153503037));
#37019=CARTESIAN_POINT('Ctrl Pts',(0.00266944295109022,-0.0256018922760762,
-0.0135566385589283));
#37020=CARTESIAN_POINT('Ctrl Pts',(0.00279629737366019,-0.0256202802424622,
-0.0132705365083005));
#37021=CARTESIAN_POINT('Ctrl Pts',(0.00284198151377146,-0.0256280164503185,
-0.0131457792102502));
#37022=CARTESIAN_POINT('Ctrl Pts',(0.00290213466171848,-0.0256401459853748,
-0.0129402159943772));
#37023=CARTESIAN_POINT('Ctrl Pts',(0.00292182033244563,-0.025644673658923,
-0.0128611295686992));
#37024=CARTESIAN_POINT('Ctrl Pts',(0.00294461775445603,-0.0256508129837517,
-0.012750498823272));
#37025=CARTESIAN_POINT('Ctrl Pts',(0.00295048633783433,-0.0256525091049688,
-0.0127195643178293));
#37026=CARTESIAN_POINT('Ctrl Pts',(0.00295972836828079,-0.0256553963747003,
-0.012666280142606));
#37027=CARTESIAN_POINT('Ctrl Pts',(0.00296333814259151,-0.0256565947877827,
-0.0126439746441169));
#37028=CARTESIAN_POINT('Ctrl Pts',(0.00296977795881066,-0.0256588784301815,
-0.0126011169283942));
#37029=CARTESIAN_POINT('Ctrl Pts',(0.00297264748124694,-0.0256599648234059,
-0.0125805720412986));
#37030=CARTESIAN_POINT('Ctrl Pts',(0.00297964611188767,-0.0256628101403707,
-0.0125263658700173));
#37031=CARTESIAN_POINT('Ctrl Pts',(0.00298341800666489,-0.0256645579799812,
-0.0124926610194363));
#37032=CARTESIAN_POINT('Ctrl Pts',(0.00299550279743585,-0.0256710970114868,
-0.0123651455504515));
#37033=CARTESIAN_POINT('Ctrl Pts',(0.00299996891933946,-0.0256757716585713,
-0.0122710219335788));
#37034=CARTESIAN_POINT('Ctrl Pts',(0.00300005839134703,-0.0256890407294522,
-0.0119984770689181));
#37035=CARTESIAN_POINT('Ctrl Pts',(0.00298421101998347,-0.0256973590325867,
-0.01182046957932));
#37036=CARTESIAN_POINT('Ctrl Pts',(0.00293046389805818,-0.0257118587188384,
-0.0115215674536747));
#37037=CARTESIAN_POINT('Ctrl Pts',(0.00290057606449068,-0.0257179340604047,
-0.0113997338968926));
#37038=CARTESIAN_POINT('Ctrl Pts',(0.00285595038363327,-0.0257256060527422,
-0.0112570873867286));
#37039=CARTESIAN_POINT('Ctrl Pts',(0.00284846105331454,-0.0257268589024376,
-0.0112341245943821));
#37040=CARTESIAN_POINT('Ctrl Pts',(0.00283622121357359,-0.0257288573636554,
-0.0111980788392584));
#37041=CARTESIAN_POINT('Ctrl Pts',(0.0028316553774092,-0.0257295928826786,
-0.0111849337890719));
#37042=CARTESIAN_POINT('Ctrl Pts',(0.00282274332623996,-0.0257310106859931,
-0.0111598406120381));
#37043=CARTESIAN_POINT('Ctrl Pts',(0.00281841236550277,-0.0257316921274252,
-0.0111478876465119));
#37044=CARTESIAN_POINT('Ctrl Pts',(0.00280763254675204,-0.0257333695566859,
-0.0111187168120117));
#37045=CARTESIAN_POINT('Ctrl Pts',(0.00280110116921717,-0.0257343701544008,
-0.0111015301277763));
#37046=CARTESIAN_POINT('Ctrl Pts',(0.00277623917153101,-0.0257381189982614,
-0.0110378764710834));
#37047=CARTESIAN_POINT('Ctrl Pts',(0.00275690765318436,-0.0257409175230551,
-0.0109918115583913));
#37048=CARTESIAN_POINT('Ctrl Pts',(0.00270241336180105,-0.0257484753448215,
-0.0108705362081398));
#37049=CARTESIAN_POINT('Ctrl Pts',(0.00266526390332989,-0.0257533024823443,
-0.0107962672387901));
#37050=CARTESIAN_POINT('Ctrl Pts',(0.00250215346147765,-0.0257730451064716,
-0.0105014219740259));
#37051=CARTESIAN_POINT('Ctrl Pts',(0.00235147810862052,-0.0257880719220853,
-0.010295671813178));
#37052=CARTESIAN_POINT('Ctrl Pts',(0.00214563544523808,-0.0258045804786426,
-0.0100786452832899));
#37053=CARTESIAN_POINT('Ctrl Pts',(0.00211387330061941,-0.0258070390703807,
-0.0100466344531266));
#37054=CARTESIAN_POINT('Ctrl Pts',(0.0020629634525884,-0.0258108451584988,
-0.00999758856376631));
#37055=CARTESIAN_POINT('Ctrl Pts',(0.00204429949412708,-0.0258122134488246,
-0.009980062986314));
#37056=CARTESIAN_POINT('Ctrl Pts',(0.00200915363851221,-0.0258147410317691,
-0.00994789739350922));
#37057=CARTESIAN_POINT('Ctrl Pts',(0.00199273041812558,-0.0258159028462061,
-0.00993319608586866));
#37058=CARTESIAN_POINT('Ctrl Pts',(0.00195567135584683,-0.0258184825632515,
-0.00990075106743063));
#37059=CARTESIAN_POINT('Ctrl Pts',(0.00193495296533104,-0.0258198964657749,
-0.00988310435905266));
#37060=CARTESIAN_POINT('Ctrl Pts',(0.00187191042619904,-0.0258241170346503,
-0.00983087172270445));
#37061=CARTESIAN_POINT('Ctrl Pts',(0.00182887747601515,-0.0258268895016612,
-0.00979715725318942));
#37062=CARTESIAN_POINT('Ctrl Pts',(0.00167250167914293,-0.0258366197536096,
-0.00968139734532663));
#37063=CARTESIAN_POINT('Ctrl Pts',(0.00155436749252544,-0.0258433400581867,
-0.00960612215275029));
#37064=CARTESIAN_POINT('Ctrl Pts',(0.0012798010660304,-0.0258581836513316,
-0.00945705430554906));
#37065=CARTESIAN_POINT('Ctrl Pts',(0.0011213901356715,-0.0258662385396847,
-0.00938798039854426));
#37066=CARTESIAN_POINT('Ctrl Pts',(0.000904484498255154,-0.0258775636091151,
-0.00931489381682784));
#37067=CARTESIAN_POINT('Ctrl Pts',(0.000850539917110885,-0.0258804049318105,
-0.0092983956548905));
#37068=CARTESIAN_POINT('Ctrl Pts',(0.000777092206148273,-0.02588434524141,
-0.00927817851820979));
#37069=CARTESIAN_POINT('Ctrl Pts',(0.000757967793312922,-0.0258853777158257,
-0.00927311731098472));
#37070=CARTESIAN_POINT('Ctrl Pts',(0.000727462656841946,-0.0258870368974471,
-0.00926536624802472));
#37071=CARTESIAN_POINT('Ctrl Pts',(0.000716113542861952,-0.025887656871205,
-0.00926255307835635));
#37072=CARTESIAN_POINT('Ctrl Pts',(0.000692016620857422,-0.0258889794760447,
-0.00925672934873053));
#37073=CARTESIAN_POINT('Ctrl Pts',(0.000679265057995674,-0.0258896830814018,
-0.00925373581236286));
#37074=CARTESIAN_POINT('Ctrl Pts',(0.000646636301346663,-0.0258914922109695,
-0.00924630104767092));
#37075=CARTESIAN_POINT('Ctrl Pts',(0.000626732973111169,-0.0258926040258825,
-0.00924197861950552));
#37076=CARTESIAN_POINT('Ctrl Pts',(0.000541028178600831,-0.025897422411502,
-0.00922427789654304));
#37077=CARTESIAN_POINT('Ctrl Pts',(0.000474835375667756,-0.0259012213897143,
-0.00921290898481249));
#37078=CARTESIAN_POINT('Ctrl Pts',(0.000273376739088949,-0.0259129092387133,
-0.00918523144127569));
#37079=CARTESIAN_POINT('Ctrl Pts',(0.000137329575514236,-0.0259209649263144,
-0.00917590451347279));
#37080=CARTESIAN_POINT('Ctrl Pts',(-0.000176554041602739,-0.0259393958263076,
-0.00917578694708795));
#37081=CARTESIAN_POINT('Ctrl Pts',(-0.000353905770131149,-0.0259496794901596,
-0.00919150501026625));
#37082=CARTESIAN_POINT('Ctrl Pts',(-0.000570080131534526,-0.0259618096690587,
-0.00923021858061489));
#37083=CARTESIAN_POINT('Ctrl Pts',(-0.000611160970754606,-0.0259640980652013,
-0.00923846708717254));
#37084=CARTESIAN_POINT('Ctrl Pts',(-0.000678424191795633,-0.0259678181641809,
-0.00925344497899387));
#37085=CARTESIAN_POINT('Ctrl Pts',(-0.000704711413619019,-0.0259692652466403,
-0.0092596722927942));
#37086=CARTESIAN_POINT('Ctrl Pts',(-0.000752281149067618,-0.0259718723268269,
-0.00927162214038809));
#37087=CARTESIAN_POINT('Ctrl Pts',(-0.000773591333962172,-0.0259730359873158,
-0.00927722568710357));
#37088=CARTESIAN_POINT('Ctrl Pts',(-0.000819685074685722,-0.0259755444342235,
-0.0092898906478453));
#37089=CARTESIAN_POINT('Ctrl Pts',(-0.000844443398024073,-0.0259768863923803,
-0.00929703766635584));
#37090=CARTESIAN_POINT('Ctrl Pts',(-0.000914265194417583,-0.0259806574821131,
-0.00931817149203214));
#37091=CARTESIAN_POINT('Ctrl Pts',(-0.000959095978073966,-0.0259830627481871,
-0.00933290388586636));
#37092=CARTESIAN_POINT('Ctrl Pts',(-0.00106021207072405,-0.025988463978135,
-0.00936879718744386));
#37093=CARTESIAN_POINT('Ctrl Pts',(-0.00111624648618063,-0.0259914398030971,
-0.00939060502486205));
#37094=CARTESIAN_POINT('Ctrl Pts',(-0.00131377751964363,-0.0260019250870548,
-0.00947440103939878));
#37095=CARTESIAN_POINT('Ctrl Pts',(-0.00145109857980862,-0.0260091922277864,
-0.00954561175001733));
#37096=CARTESIAN_POINT('Ctrl Pts',(-0.00170668862246993,-0.0260234664260622,
-0.00970428678456888));
#37097=CARTESIAN_POINT('Ctrl Pts',(-0.00182522328655958,-0.0260304530712585,
-0.0097904855488409));
#37098=CARTESIAN_POINT('Ctrl Pts',(-0.00196064150094307,-0.0260394671347499,
-0.00990498454487402));
#37099=CARTESIAN_POINT('Ctrl Pts',(-0.00198398858325478,-0.0260410620005325,
-0.00992535354261215));
#37100=CARTESIAN_POINT('Ctrl Pts',(-0.0020183975185759,-0.0260434814093708,
-0.0099563249625849));
#37101=CARTESIAN_POINT('Ctrl Pts',(-0.00202970104302239,-0.0260442876217778,
-0.00996665701187283));
#37102=CARTESIAN_POINT('Ctrl Pts',(-0.00205003983561637,-0.0260457601625911,
-0.00998553565174353));
#37103=CARTESIAN_POINT('Ctrl Pts',(-0.00205910175249264,-0.0260464243535992,
-0.00999405251015095));
#37104=CARTESIAN_POINT('Ctrl Pts',(-0.00207971885800195,-0.0260479540977671,
-0.0100136723835053));
#37105=CARTESIAN_POINT('Ctrl Pts',(-0.00209123822985529,-0.0260488222962515,
-0.0100248118111333));
#37106=CARTESIAN_POINT('Ctrl Pts',(-0.00212746526468485,-0.026051594100147,
-0.0100604100142113));
#37107=CARTESIAN_POINT('Ctrl Pts',(-0.00215183651611916,-0.0260535207837809,
-0.010085205516918));
#37108=CARTESIAN_POINT('Ctrl Pts',(-0.00220969227820255,-0.0260582345962579,
-0.0101461519148889));
#37109=CARTESIAN_POINT('Ctrl Pts',(-0.00224272734787067,-0.0260610445306258,
-0.0101827147454583));
#37110=CARTESIAN_POINT('Ctrl Pts',(-0.00237889231780473,-0.0260730839658959,
-0.0103410935989622));
#37111=CARTESIAN_POINT('Ctrl Pts',(-0.0024731143470861,-0.0260825636264007,
-0.0104702223962119));
#37112=CARTESIAN_POINT('Ctrl Pts',(-0.00264146276556717,-0.02610136652058,
-0.0107444302161605));
#37113=CARTESIAN_POINT('Ctrl Pts',(-0.00271497235936262,-0.0261106510162668,
-0.0108892940913171));
#37114=CARTESIAN_POINT('Ctrl Pts',(-0.00279095479310238,-0.0261216422173249,
-0.0110749245195623));
#37115=CARTESIAN_POINT('Ctrl Pts',(-0.00280481021886816,-0.0261237231689978,
-0.0111107182582934));
#37116=CARTESIAN_POINT('Ctrl Pts',(-0.00282619413579598,-0.0261270667385175,
-0.0111692745537152));
#37117=CARTESIAN_POINT('Ctrl Pts',(-0.00283414303494523,-0.0261283429465237,
-0.0111918780119223));
#37118=CARTESIAN_POINT('Ctrl Pts',(-0.00284899790785426,-0.0261307952602463,
-0.0112357933590812));
#37119=CARTESIAN_POINT('Ctrl Pts',(-0.00285593760926345,-0.026131972394603,
-0.0112570920801973));
#37120=CARTESIAN_POINT('Ctrl Pts',(-0.0028716908118266,-0.0261347219926009,
-0.0113073443704551));
#37121=CARTESIAN_POINT('Ctrl Pts',(-0.00288030610176168,-0.0261362880172093,
-0.0113363577821861));
#37122=CARTESIAN_POINT('Ctrl Pts',(-0.00290814704702146,-0.0261415758641783,
-0.0114355957033733));
#37123=CARTESIAN_POINT('Ctrl Pts',(-0.00292525554449036,-0.0261452312859027,
-0.0115063896501784));
#37124=CARTESIAN_POINT('Ctrl Pts',(-0.00296187104492923,-0.0261542941812586,
-0.011686357519684));
#37125=CARTESIAN_POINT('Ctrl Pts',(-0.00297793404631481,-0.0261596099782093,
-0.0117961205545347));
#37126=CARTESIAN_POINT('Ctrl Pts',(-0.00300300929215862,-0.026172885761028,
-0.0120743011820653));
#37127=CARTESIAN_POINT('Ctrl Pts',(-0.00300397348118124,-0.026180752556728,
-0.0122430429054789));
#37128=CARTESIAN_POINT('Ctrl Pts',(-0.00298594305059408,-0.0261920889618934,
-0.0124724044340214));
#37129=CARTESIAN_POINT('Ctrl Pts',(-0.00297922101199773,-0.0261951828448286,
-0.0125336796833466));
#37130=CARTESIAN_POINT('Ctrl Pts',(-0.00296776744903848,-0.0261994210259704,
-0.012614912524563));
#37131=CARTESIAN_POINT('Ctrl Pts',(-0.00296471149164684,-0.0262004852954412,
-0.0126350943706082));
#37132=CARTESIAN_POINT('Ctrl Pts',(-0.00295956235644654,-0.0262021827739815,
-0.0126669033729147));
#37133=CARTESIAN_POINT('Ctrl Pts',(-0.00295760598170671,-0.0262028086832761,
-0.0126785523780043));
#37134=CARTESIAN_POINT('Ctrl Pts',(-0.00295335953302141,-0.0262041293172166,
-0.0127029541729565));
#37135=CARTESIAN_POINT('Ctrl Pts',(-0.00295105556535897,-0.0262048248529811,
-0.0127157041054001));
#37136=CARTESIAN_POINT('Ctrl Pts',(-0.00294503817338269,-0.0262065897259424,
-0.0127478137273511));
#37137=CARTESIAN_POINT('Ctrl Pts',(-0.00294121641468453,-0.0262076647992908,
-0.012767152322083));
#37138=CARTESIAN_POINT('Ctrl Pts',(-0.0029248005745554,-0.0262121005598569,
-0.0128461186396004));
#37139=CARTESIAN_POINT('Ctrl Pts',(-0.00291058216053183,-0.0262155371721572,
-0.0129053905350537));
#37140=CARTESIAN_POINT('Ctrl Pts',(-0.0028644813789978,-0.026225584799816,
-0.013074661966317));
#37141=CARTESIAN_POINT('Ctrl Pts',(-0.00282809387749655,-0.0262323197133492,
-0.0131833222169843));
#37142=CARTESIAN_POINT('Ctrl Pts',(-0.00270814621452849,-0.0262513234098642,
-0.013483314142516));
#37143=CARTESIAN_POINT('Ctrl Pts',(-0.00261070565950489,-0.0262634973326678,
-0.0136684177475832));
#37144=CARTESIAN_POINT('Ctrl Pts',(-0.00246980038471531,-0.0262775004239674,
-0.0138794136081842));
#37145=CARTESIAN_POINT('Ctrl Pts',(-0.00244392541500113,-0.0262799583167868,
-0.0139163303977391));
#37146=CARTESIAN_POINT('Ctrl Pts',(-0.00240207376419642,-0.0262837628750102,
-0.0139732670575144));
#37147=CARTESIAN_POINT('Ctrl Pts',(-0.00238665675298442,-0.0262851303456879,
-0.013993688326132));
#37148=CARTESIAN_POINT('Ctrl Pts',(-0.00235748716780589,-0.0262876561247282,
-0.0140313152896178));
#37149=CARTESIAN_POINT('Ctrl Pts',(-0.00234380281635463,-0.0262888169576663,
-0.0140485714671085));
#37150=CARTESIAN_POINT('Ctrl Pts',(-0.00231280599341356,-0.0262913940876831,
-0.0140867869149724));
#37151=CARTESIAN_POINT('Ctrl Pts',(-0.00229539606198751,-0.0262928063950667,
-0.0141076648397084));
#37152=CARTESIAN_POINT('Ctrl Pts',(-0.00224219520198089,-0.0262970205281855,
-0.0141697283015315));
#37153=CARTESIAN_POINT('Ctrl Pts',(-0.00220556131244758,-0.0262997882604862,
-0.014210177905968));
#37154=CARTESIAN_POINT('Ctrl Pts',(-0.00207225391405662,-0.0263094331570109,
-0.014349533628757));
#37155=CARTESIAN_POINT('Ctrl Pts',(-0.00196986552819778,-0.026316079143308,
-0.0144427357986513));
#37156=CARTESIAN_POINT('Ctrl Pts',(-0.00172838896540962,-0.0263307112070987,
-0.0146337876498034));
#37157=CARTESIAN_POINT('Ctrl Pts',(-0.0015866932847853,-0.0263386308302992,
-0.0147275522000348));
#37158=CARTESIAN_POINT('Ctrl Pts',(-0.00138507930899339,-0.0263499624349665,
-0.0148376515208313));
#37159=CARTESIAN_POINT('Ctrl Pts',(-0.00133146224695846,-0.0263529833646708,
-0.0148648720590887));
#37160=CARTESIAN_POINT('Ctrl Pts',(-0.00125876347347922,-0.0263571353441502,
-0.0148990726469535));
#37161=CARTESIAN_POINT('Ctrl Pts',(-0.00124037374313603,-0.0263581903017766,
-0.0149074978647041));
#37162=CARTESIAN_POINT('Ctrl Pts',(-0.00121115133263792,-0.026359876184706,
-0.0149205301308951));
#37163=CARTESIAN_POINT('Ctrl Pts',(-0.00120037401867651,-0.0263604999658543,
-0.0149252606292993));
#37164=CARTESIAN_POINT('Ctrl Pts',(-0.00117763892437462,-0.0263618206533458,
-0.0149350806155248));
#37165=CARTESIAN_POINT('Ctrl Pts',(-0.00116567548548739,-0.0263625184196523,
-0.0149401560076386));
#37166=CARTESIAN_POINT('Ctrl Pts',(-0.00113532685196329,-0.0263642948901051,
-0.0149527991315181));
#37167=CARTESIAN_POINT('Ctrl Pts',(-0.00111689887680067,-0.0263653794697229,
-0.0149602620466994));
#37168=CARTESIAN_POINT('Ctrl Pts',(-0.00104031175263584,-0.0263699072150745,
-0.0149903954986541));
#37169=CARTESIAN_POINT('Ctrl Pts',(-0.000981529315005994,-0.0263734300705311,
-0.0150114300559489));
#37170=CARTESIAN_POINT('Ctrl Pts',(-0.000808601434267826,-0.0263838472663003,
-0.0150672887774806));
#37171=CARTESIAN_POINT('Ctrl Pts',(-0.000692982526473934,-0.0263908747727479,
-0.0150971558521233));
#37172=CARTESIAN_POINT('Ctrl Pts',(-0.000378079364101146,-0.0264097470162851,
-0.0151587520706844));
#37173=CARTESIAN_POINT('Ctrl Pts',(-0.000176839674301235,-0.0264214896326742,
-0.0151774158198483));
#37174=CARTESIAN_POINT('Ctrl Pts',(7.02431736514861E-5,-0.0264351319563392,
-0.0151753755308247));
#37175=CARTESIAN_POINT('Ctrl Pts',(0.000115701800131155,-0.0264376123034122,
-0.0151739662259297));
#37176=CARTESIAN_POINT('Ctrl Pts',(0.000186767158066899,-0.0264414447803659,
-0.0151701442025625));
#37177=CARTESIAN_POINT('Ctrl Pts',(0.00021240346732146,-0.0264428181529634,
-0.0151684349285025));
#37178=CARTESIAN_POINT('Ctrl Pts',(0.000259992804911569,-0.0264453512504799,
-0.0151646473269047));
#37179=CARTESIAN_POINT('Ctrl Pts',(0.000281950823223422,-0.0264465135630514,
-0.0151626558984039));
#37180=CARTESIAN_POINT('Ctrl Pts',(0.000330875203223684,-0.0264490896074626,
-0.0151576744762023));
#37181=CARTESIAN_POINT('Ctrl Pts',(0.000357827136870877,-0.026450499415262,
-0.0151545603566988));
#37182=CARTESIAN_POINT('Ctrl Pts',(0.000438449604974007,-0.0264546911888428,
-0.0151441348752801));
#37183=CARTESIAN_POINT('Ctrl Pts',(0.00049196938162317,-0.026457439718098,
-0.0151357350788764));
#37184=CARTESIAN_POINT('Ctrl Pts',(0.000750342620371381,-0.0264705865611251,
-0.0150879817748392));
#37185=CARTESIAN_POINT('Ctrl Pts',(0.000950936046794013,-0.0264803698107777,
-0.0150287873051669));
#37186=CARTESIAN_POINT('Ctrl Pts',(0.00127370367310936,-0.026496950193539,
-0.014895675239027));
#37187=CARTESIAN_POINT('Ctrl Pts',(0.0013996948785352,-0.0265036754519913,
-0.0148330322021753));
#37188=CARTESIAN_POINT('Ctrl Pts',(0.0015476722691891,-0.0265123999897581,
-0.0147460052309575));
#37189=CARTESIAN_POINT('Ctrl Pts',(0.00157427643719887,-0.0265140033424187,
-0.0147297961258277));
#37190=CARTESIAN_POINT('Ctrl Pts',(0.00161361118385055,-0.0265164336386123,
-0.0147049825426861));
#37191=CARTESIAN_POINT('Ctrl Pts',(0.00162653661688444,-0.026517242052961,
-0.0146966893504206));
#37192=CARTESIAN_POINT('Ctrl Pts',(0.00164984013887743,-0.0265187184946581,
-0.0146814835453238));
#37193=CARTESIAN_POINT('Ctrl Pts',(0.00166023960202947,-0.0265193843762967,
-0.0146746049602128));
#37194=CARTESIAN_POINT('Ctrl Pts',(0.00168394093277497,-0.0265209180085231,
-0.0146587147549854));
#37195=CARTESIAN_POINT('Ctrl Pts',(0.00169721353488977,-0.0265217884123444,
-0.0146496609449121));
#37196=CARTESIAN_POINT('Ctrl Pts',(0.00173901366532376,-0.0265245648314106,
-0.0146206525558815));
#37197=CARTESIAN_POINT('Ctrl Pts',(0.00176726602409027,-0.0265264938684584,
-0.0146003083992853));
#37198=CARTESIAN_POINT('Ctrl Pts',(0.00183468362650029,-0.0265312129742921,
-0.0145499572950523));
#37199=CARTESIAN_POINT('Ctrl Pts',(0.00187347466118594,-0.0265340257695353,
-0.0145194671895346));
#37200=CARTESIAN_POINT('Ctrl Pts',(0.00203486975796642,-0.0265460922967348,
-0.0143860409479122));
#37201=CARTESIAN_POINT('Ctrl Pts',(0.00214988197452682,-0.026555595180676,
-0.0142743364450816));
#37202=CARTESIAN_POINT('Ctrl Pts',(0.00236110692921097,-0.0265742987755129,
-0.0140335019693678));
#37203=CARTESIAN_POINT('Ctrl Pts',(0.00245696744520741,-0.0265834669232397,
-0.0139047277797845));
#37204=CARTESIAN_POINT('Ctrl Pts',(0.00256244299038546,-0.026594349622514,
-0.0137364157340204));
#37205=CARTESIAN_POINT('Ctrl Pts',(0.00258217329610803,-0.0265964278082052,
-0.0137035477862005));
#37206=CARTESIAN_POINT('Ctrl Pts',(0.00261321642752148,-0.0265997699390877,
-0.0136495137347939));
#37207=CARTESIAN_POINT('Ctrl Pts',(0.00262491432953693,-0.0266010473681421,
-0.0136285748777071));
#37208=CARTESIAN_POINT('Ctrl Pts',(0.0026470791993611,-0.0266035041173972,
-0.0135877584686789));
#37209=CARTESIAN_POINT('Ctrl Pts',(0.00265757644586538,-0.0266046844387135,
-0.0135678992634247));
#37210=CARTESIAN_POINT('Ctrl Pts',(0.00268175869663563,-0.0266074448251034,
-0.013520879361923));
#37211=CARTESIAN_POINT('Ctrl Pts',(0.0026952558125526,-0.0266090183668267,
-0.0134936245269545));
#37212=CARTESIAN_POINT('Ctrl Pts',(0.00273996377325103,-0.0266143505566001,
-0.0133997837356761));
#37213=CARTESIAN_POINT('Ctrl Pts',(0.00276914091869512,-0.0266180414194744,
-0.0133322558320741));
#37214=CARTESIAN_POINT('Ctrl Pts',(0.00283658452337156,-0.0266272156818553,
-0.0131589263758013));
#37215=CARTESIAN_POINT('Ctrl Pts',(0.00287143786491108,-0.0266326043944009,
-0.0130519189387326));
#37216=CARTESIAN_POINT('Ctrl Pts',(0.00295440815394613,-0.0266480164384357,
-0.0127383324975869));
#37217=CARTESIAN_POINT('Ctrl Pts',(0.00298674724158532,-0.0266578551249714,
-0.0125283180125818));
#37218=CARTESIAN_POINT('Ctrl Pts',(0.00299806883616562,-0.0266701414401903,
-0.0122873988315587));
#37219=CARTESIAN_POINT('Ctrl Pts',(0.00299901552943678,-0.0266716528024666,
-0.0122581022274078));
#37220=CARTESIAN_POINT('Ctrl Pts',(0.00299970122819703,-0.0266736852041671,
-0.0122192542508606));
#37221=CARTESIAN_POINT('Ctrl Pts',(0.00299982412743131,-0.0266741867732736,
-0.0122097103670345));
#37222=CARTESIAN_POINT('Ctrl Pts',(0.00299996762782709,-0.0266751217604859,
-0.0121920042481002));
#37223=CARTESIAN_POINT('Ctrl Pts',(0.0030000004394171,-0.0266755539940525,
-0.0121838521580368));
#37224=CARTESIAN_POINT('Ctrl Pts',(0.00299999999556417,-0.0266759885990988,
-0.0121756901455692));
#37225=CARTESIAN_POINT('',(-0.0030008859025812,-0.0271782456277452,-0.0121752776264524));
#37226=CARTESIAN_POINT('Ctrl Pts',(0.00299999999556417,-0.0266759885990988,
-0.0121756901455692));
#37227=CARTESIAN_POINT('Ctrl Pts',(0.00299999959124405,-0.026676384495016,
-0.0121682551020984));
#37228=CARTESIAN_POINT('Ctrl Pts',(0.00299997154769017,-0.0266767819272223,
-0.0121608202951627));
#37229=CARTESIAN_POINT('Ctrl Pts',(0.00299984500965966,-0.0266776885879081,
-0.0121439247657658));
#37230=CARTESIAN_POINT('Ctrl Pts',(0.00299972939971157,-0.0266781987292689,
-0.0121344644467317));
#37231=CARTESIAN_POINT('Ctrl Pts',(0.00299921172118187,-0.026679853116644,
-0.0121039263214186));
#37232=CARTESIAN_POINT('Ctrl Pts',(0.00299863223187566,-0.0266810065230799,
-0.0120828526144914));
#37233=CARTESIAN_POINT('Ctrl Pts',(0.00299496888804635,-0.0266863243563261,
-0.0119865742101401));
#37234=CARTESIAN_POINT('Ctrl Pts',(0.00298927770430945,-0.0266906052947664,
-0.0119115004943302));
#37235=CARTESIAN_POINT('Ctrl Pts',(0.00296196053497696,-0.0267045689040371,
-0.0116713953060827));
#37236=CARTESIAN_POINT('Ctrl Pts',(0.00292942835960164,-0.0267144745978878,
-0.0115079176724795));
#37237=CARTESIAN_POINT('Ctrl Pts',(0.00285504456101083,-0.0267302086016848,
-0.0112488363902317));
#37238=CARTESIAN_POINT('Ctrl Pts',(0.00282148375743838,-0.0267361500012816,
-0.0111512207070386));
#37239=CARTESIAN_POINT('Ctrl Pts',(0.00275705406418017,-0.0267458503987208,
-0.0109911742109662));
#37240=CARTESIAN_POINT('Ctrl Pts',(0.00272892457493658,-0.0267496846736673,
-0.0109277413684892));
#37241=CARTESIAN_POINT('Ctrl Pts',(0.00268570262590721,-0.0267550491816169,
-0.0108387385833227));
#37242=CARTESIAN_POINT('Ctrl Pts',(0.00267239291374361,-0.0267566389265011,
-0.0108123319172534));
#37243=CARTESIAN_POINT('Ctrl Pts',(0.00264844841823185,-0.0267593942448047,
-0.0107665235867418));
#37244=CARTESIAN_POINT('Ctrl Pts',(0.00263798555238983,-0.0267605656713797,
-0.0107470350729112));
#37245=CARTESIAN_POINT('Ctrl Pts',(0.0026157857455541,-0.026762985550449,
-0.010706760147235));
#37246=CARTESIAN_POINT('Ctrl Pts',(0.00260401430233,-0.0267642326766404,
-0.0106859944760083));
#37247=CARTESIAN_POINT('Ctrl Pts',(0.00257251701811284,-0.0267674786159811,
-0.0106319449566617));
#37248=CARTESIAN_POINT('Ctrl Pts',(0.00255239268973123,-0.026769463093696,
-0.0105988978428446));
#37249=CARTESIAN_POINT('Ctrl Pts',(0.00244132880068725,-0.0267799675406711,
-0.0104242132930148));
#37250=CARTESIAN_POINT('Ctrl Pts',(0.0023392251403436,-0.026788066913517,
-0.0102900213220678));
#37251=CARTESIAN_POINT('Ctrl Pts',(0.00212285019202616,-0.0268033919536706,
-0.0100504416343587));
#37252=CARTESIAN_POINT('Ctrl Pts',(0.00201060542073186,-0.0268106183249926,
-0.00994396419309953));
#37253=CARTESIAN_POINT('Ctrl Pts',(0.0018530684175075,-0.0268205491806233,
-0.00981609004527654));
#37254=CARTESIAN_POINT('Ctrl Pts',(0.00181473752270681,-0.0268229517190221,
-0.00978648674939442));
#37255=CARTESIAN_POINT('Ctrl Pts',(0.00174808341450948,-0.0268271370605342,
-0.00973753848139958));
#37256=CARTESIAN_POINT('Ctrl Pts',(0.00172011364542257,-0.0268288955279405,
-0.0097177272580704));
#37257=CARTESIAN_POINT('Ctrl Pts',(0.0016787209442918,-0.0268315105944537,
-0.00968946086469258));
#37258=CARTESIAN_POINT('Ctrl Pts',(0.00166555976050306,-0.0268323439151437,
-0.00968062545194766));
#37259=CARTESIAN_POINT('Ctrl Pts',(0.00164200961327199,-0.0268338394362079,
-0.00966508501680036));
#37260=CARTESIAN_POINT('Ctrl Pts',(0.00163164832784109,-0.0268344989835844,
-0.009658339314924));
#37261=CARTESIAN_POINT('Ctrl Pts',(0.00160837986177967,-0.0268359836978885,
-0.00964339439712793));
#37262=CARTESIAN_POINT('Ctrl Pts',(0.00159545154923154,-0.0268368109485204,
-0.00963522971340862));
#37263=CARTESIAN_POINT('Ctrl Pts',(0.00155617820362321,-0.0268393295759174,
-0.0096108451899833));
#37264=CARTESIAN_POINT('Ctrl Pts',(0.00152964485720779,-0.0268410387475932,
-0.00959493414768093));
#37265=CARTESIAN_POINT('Ctrl Pts',(0.00137893508806576,-0.0268507686562533,
-0.00950769953436586));
#37266=CARTESIAN_POINT('Ctrl Pts',(0.00125003018846361,-0.0268591644455779,
-0.00944493310314055));
#37267=CARTESIAN_POINT('Ctrl Pts',(0.000926365096198284,-0.0268796819872125,
-0.00931506570535079));
#37268=CARTESIAN_POINT('Ctrl Pts',(0.000728194922046586,-0.026891747296662,
-0.00925831835760775));
#37269=CARTESIAN_POINT('Ctrl Pts',(0.000470225348096314,-0.0269063413553884,
-0.00921239751836219));
#37270=CARTESIAN_POINT('Ctrl Pts',(0.000414419374138996,-0.026909438044452,
-0.00920407955211752));
#37271=CARTESIAN_POINT('Ctrl Pts',(0.000331026879324982,-0.0269139772527621,
-0.00919404479803303));
#37272=CARTESIAN_POINT('Ctrl Pts',(0.000303599676465059,-0.0269154561092014,
-0.00919112750983954));
#37273=CARTESIAN_POINT('Ctrl Pts',(0.000254114374587732,-0.026918099834978,
-0.00918655320820368));
#37274=CARTESIAN_POINT('Ctrl Pts',(0.000232071030441415,-0.0269192687671969,
-0.0091847611539763));
#37275=CARTESIAN_POINT('Ctrl Pts',(0.000184629413821385,-0.0269217665198699,
-0.00918143192349406));
#37276=CARTESIAN_POINT('Ctrl Pts',(0.000159227232531907,-0.0269230928346091,
-0.00917997377293681));
#37277=CARTESIAN_POINT('Ctrl Pts',(8.96775204830524E-5,-0.0269266957094395,
-0.00917686855554262));
#37278=CARTESIAN_POINT('Ctrl Pts',(4.55065501382071E-5,-0.0269289524357815,
-0.00917587314000559));
#37279=CARTESIAN_POINT('Ctrl Pts',(-0.000145392922756357,-0.026938589684486,
-0.00917578862158119));
#37280=CARTESIAN_POINT('Ctrl Pts',(-0.000291929094222405,-0.0269456791476955,
-0.00918648718843781));
#37281=CARTESIAN_POINT('Ctrl Pts',(-0.000536536556900168,-0.0269574606377949,
-0.00922251107710548));
#37282=CARTESIAN_POINT('Ctrl Pts',(-0.000635171503360813,-0.026962200415781,
-0.00924214256734746));
#37283=CARTESIAN_POINT('Ctrl Pts',(-0.000856516629671363,-0.0269731046238776,
-0.00929788535138056));
#37284=CARTESIAN_POINT('Ctrl Pts',(-0.000978268969247597,-0.0269792953198636,
-0.00933696195306479));
#37285=CARTESIAN_POINT('Ctrl Pts',(-0.00111974546700643,-0.0269870983043951,
-0.00939255316161758));
#37286=CARTESIAN_POINT('Ctrl Pts',(-0.00114223378297961,-0.0269883576823508,
-0.00940170631664954));
#37287=CARTESIAN_POINT('Ctrl Pts',(-0.00117751931476832,-0.0269903675353013,
-0.0094165699465951));
#37288=CARTESIAN_POINT('Ctrl Pts',(-0.00119039227924913,-0.0269911079519724,
-0.00942209903226777));
#37289=CARTESIAN_POINT('Ctrl Pts',(-0.00121518988955551,-0.0269925490010256,
-0.00943295625757536));
#37290=CARTESIAN_POINT('Ctrl Pts',(-0.00122711936831542,-0.026993248932969,
-0.00943827248974219));
#37291=CARTESIAN_POINT('Ctrl Pts',(-0.0012563792802428,-0.0269949814778576,
-0.00945154150303195));
#37292=CARTESIAN_POINT('Ctrl Pts',(-0.0012736691823936,-0.026996018975379,
-0.00945958187756178));
#37293=CARTESIAN_POINT('Ctrl Pts',(-0.00133879210116586,-0.0269999756208012,
-0.00949062465757286));
#37294=CARTESIAN_POINT('Ctrl Pts',(-0.00138608632814361,-0.0270029495023824,
-0.00951472924700927));
#37295=CARTESIAN_POINT('Ctrl Pts',(-0.00151279953447129,-0.027011145723247,
-0.00958360593190222));
#37296=CARTESIAN_POINT('Ctrl Pts',(-0.00159085659497257,-0.0270164450639113,
-0.0096307633751304));
#37297=CARTESIAN_POINT('Ctrl Pts',(-0.00186485706128705,-0.0270357003400356,
-0.00981383372900022));
#37298=CARTESIAN_POINT('Ctrl Pts',(-0.00204661353808642,-0.0270496586464745,
-0.00996944576964931));
#37299=CARTESIAN_POINT('Ctrl Pts',(-0.00223580051543524,-0.0270650000859256,
-0.0101751340092416));
#37300=CARTESIAN_POINT('Ctrl Pts',(-0.00226293997817949,-0.0270672268682731,
-0.0102058826149279));
#37301=CARTESIAN_POINT('Ctrl Pts',(-0.00230541556461921,-0.0270707556431898,
-0.0102560433711941));
#37302=CARTESIAN_POINT('Ctrl Pts',(-0.00232115623375781,-0.0270720735012948,
-0.0102751047961467));
#37303=CARTESIAN_POINT('Ctrl Pts',(-0.00235081546114359,-0.0270745770331205,
-0.0103119390959857));
#37304=CARTESIAN_POINT('Ctrl Pts',(-0.00236477248109318,-0.0270757641570953,
-0.0103296787034528));
#37305=CARTESIAN_POINT('Ctrl Pts',(-0.00239663477829766,-0.0270784962434833,
-0.0103711304624337));
#37306=CARTESIAN_POINT('Ctrl Pts',(-0.00241439078548372,-0.0270800354614905,
-0.0103949546516549));
#37307=CARTESIAN_POINT('Ctrl Pts',(-0.00247141546155795,-0.0270850381686923,
-0.0104738884797533));
#37308=CARTESIAN_POINT('Ctrl Pts',(-0.00250917509071342,-0.0270884461688752,
-0.0105300647869997));
#37309=CARTESIAN_POINT('Ctrl Pts',(-0.00259316013190938,-0.0270963047104576,
-0.0106646309714038));
#37310=CARTESIAN_POINT('Ctrl Pts',(-0.00263778381183813,-0.0271007055093122,
-0.0107439418955299));
#37311=CARTESIAN_POINT('Ctrl Pts',(-0.00275800636705107,-0.0271134726400279,
-0.0109823711484938));
#37312=CARTESIAN_POINT('Ctrl Pts',(-0.00282327894873937,-0.0271216561485499,
-0.0111462466035163));
#37313=CARTESIAN_POINT('Ctrl Pts',(-0.00289698863239526,-0.0271341494586836,
-0.0113922821795902));
#37314=CARTESIAN_POINT('Ctrl Pts',(-0.00291703674722833,-0.0271381577390677,
-0.0114705720971312));
#37315=CARTESIAN_POINT('Ctrl Pts',(-0.00293853432553869,-0.027143460465929,
-0.0115712800107197));
#37316=CARTESIAN_POINT('Ctrl Pts',(-0.00294292751286983,-0.027144614910176,
-0.0115930407725214));
#37317=CARTESIAN_POINT('Ctrl Pts',(-0.00294959897100789,-0.0271464908778866,
-0.0116280873230505));
#37318=CARTESIAN_POINT('Ctrl Pts',(-0.00295202997664888,-0.0271472042766585,
-0.0116413435639292));
#37319=CARTESIAN_POINT('Ctrl Pts',(-0.00295651709088547,-0.0271485810463615,
-0.0116667764898916));
#37320=CARTESIAN_POINT('Ctrl Pts',(-0.00295858742861884,-0.0271492436209307,
-0.0116789499618797));
#37321=CARTESIAN_POINT('Ctrl Pts',(-0.00296257988336301,-0.0271505782496488,
-0.0117033353077343));
#37322=CARTESIAN_POINT('Ctrl Pts',(-0.00296450169884491,-0.0271512501859289,
-0.0117155463540992));
#37323=CARTESIAN_POINT('Ctrl Pts',(-0.00296898163759094,-0.0271528903073936,
-0.011745203828794));
#37324=CARTESIAN_POINT('Ctrl Pts',(-0.00297146148759825,-0.0271538625870964,
-0.0117626614210104));
#37325=CARTESIAN_POINT('Ctrl Pts',(-0.0029912177740022,-0.0271621833190282,
-0.0119111297951135));
#37326=CARTESIAN_POINT('Ctrl Pts',(-0.00299997282133411,-0.0271699176173088,
-0.0120431172027518));
#37327=CARTESIAN_POINT('Ctrl Pts',(-0.00299999993681902,-0.0271777321248805,
-0.0121752375870697));
#37328=CARTESIAN_POINT('',(-0.00212132034355963,-0.0271787743898723,-0.0100545329429984));
#37329=CARTESIAN_POINT('Origin',(0.,-0.0271787743898623,-0.0121758532865581));
#37330=CARTESIAN_POINT('',(0.00299984018495948,-0.026803478798527,-0.0121744321482416));
#37331=CARTESIAN_POINT('Ctrl Pts',(-0.00212132034355963,-0.0271787743898623,
-0.0100545329429984));
#37332=CARTESIAN_POINT('Ctrl Pts',(-0.0017049049496698,-0.0271475243898623,
-0.00963811754910862));
#37333=CARTESIAN_POINT('Ctrl Pts',(-0.000620685517841953,-0.0270850243898623,
-0.00905869905246725));
#37334=CARTESIAN_POINT('Ctrl Pts',(0.00121551243098668,-0.0269912743898623,
-0.00923888272063218));
#37335=CARTESIAN_POINT('Ctrl Pts',(0.00264200403629968,-0.0268975243898623,
-0.0104090155171674));
#37336=CARTESIAN_POINT('Ctrl Pts',(0.00299965007763634,-0.0268350243898623,
-0.0115851731935525));
#37337=CARTESIAN_POINT('Ctrl Pts',(0.00299999947199319,-0.0268037743898623,
-0.0121740733875246));
#37338=CARTESIAN_POINT('',(0.00299996104327479,-0.0258037247414263,-0.012178123434659));
#37339=CARTESIAN_POINT('Ctrl Pts',(0.00299924423124766,-0.026802372878294,
-0.0121757744092904));
#37340=CARTESIAN_POINT('Ctrl Pts',(0.00299673535939128,-0.0267690941025886,
-0.0127901983170197));
#37341=CARTESIAN_POINT('Ctrl Pts',(0.00280417962540106,-0.0267405918373098,
-0.0134078575495431));
#37342=CARTESIAN_POINT('Ctrl Pts',(0.00245082462041977,-0.0267078460568593,
-0.0139079213177871));
#37343=CARTESIAN_POINT('Ctrl Pts',(0.00235267788581048,-0.0266987506955989,
-0.0140468174003604));
#37344=CARTESIAN_POINT('Ctrl Pts',(0.00224210112526474,-0.0266893279522048,
-0.0141768653338118));
#37345=CARTESIAN_POINT('Ctrl Pts',(0.00212149108837053,-0.026679384540145,
-0.0142973544746626));
#37346=CARTESIAN_POINT('Ctrl Pts',(0.00184406930202044,-0.0266565131506066,
-0.0145744981813672));
#37347=CARTESIAN_POINT('Ctrl Pts',(0.00151025687286574,-0.0266347599993199,
-0.0147954171162992));
#37348=CARTESIAN_POINT('Ctrl Pts',(0.00114761927794851,-0.0266145858206189,
-0.0149461376973214));
#37349=CARTESIAN_POINT('Ctrl Pts',(0.000784981683031277,-0.0265944116419178,
-0.0150968582783436));
#37350=CARTESIAN_POINT('Ctrl Pts',(0.000392670575038502,-0.0265762819668012,
-0.0151766221497208));
#37351=CARTESIAN_POINT('Ctrl Pts',(-8.02388683067743E-8,-0.026555854964913,
-0.015176884072056));
#37352=CARTESIAN_POINT('Ctrl Pts',(-3.48441082191312E-5,-0.0265540468932306,
-0.0151769072557988));
#37353=CARTESIAN_POINT('Ctrl Pts',(-6.95979448631588E-5,-0.0265522128925814,
-0.0151763233275736));
#37354=CARTESIAN_POINT('Ctrl Pts',(-0.000104324389202502,-0.0265503565989124,
-0.0151751169414781));
#37355=CARTESIAN_POINT('Ctrl Pts',(-0.000461925943243557,-0.0265312410944776,
-0.0151626939724487));
#37356=CARTESIAN_POINT('Ctrl Pts',(-0.000817299624760045,-0.0265097615922842,
-0.0150840165707924));
#37357=CARTESIAN_POINT('Ctrl Pts',(-0.0011475009811764,-0.0264898884970649,
-0.0149464508263995));
#37358=CARTESIAN_POINT('Ctrl Pts',(-0.00150976796732726,-0.0264680855390495,
-0.0147955261658843));
#37359=CARTESIAN_POINT('Ctrl Pts',(-0.0018427597207118,-0.0264480613803005,
-0.014573950245931));
#37360=CARTESIAN_POINT('Ctrl Pts',(-0.0021212251561902,-0.0264288151819772,
-0.0142971007571688));
#37361=CARTESIAN_POINT('Ctrl Pts',(-0.0022604578739294,-0.0264191920828156,
-0.0141586760127877));
#37362=CARTESIAN_POINT('Ctrl Pts',(-0.0023860677632882,-0.0264096886133638,
-0.0140064727610748));
#37363=CARTESIAN_POINT('Ctrl Pts',(-0.00249534694135949,-0.0263995873087897,
-0.0138430823230018));
#37364=CARTESIAN_POINT('Ctrl Pts',(-0.00251954374151962,-0.026397350659023,
-0.0138069041063652));
#37365=CARTESIAN_POINT('Ctrl Pts',(-0.00254295703839925,-0.0263950717229805,
-0.0137701933918611));
#37366=CARTESIAN_POINT('Ctrl Pts',(-0.00256553425346917,-0.0263927564010959,
-0.013732978367566));
#37367=CARTESIAN_POINT('Ctrl Pts',(-0.00264492173991561,-0.0263846151142205,
-0.0136021204549458));
#37368=CARTESIAN_POINT('Ctrl Pts',(-0.00271394351715795,-0.0263760239482695,
-0.0134649978038269));
#37369=CARTESIAN_POINT('Ctrl Pts',(-0.00277208227918624,-0.0263672394278163,
-0.0133240399300175));
#37370=CARTESIAN_POINT('Ctrl Pts',(-0.00284675527592791,-0.0263559566545977,
-0.0131429946775136));
#37371=CARTESIAN_POINT('Ctrl Pts',(-0.00290345548498638,-0.0263445811317006,
-0.0129555559153653));
#37372=CARTESIAN_POINT('Ctrl Pts',(-0.00294150162794113,-0.0263336547667514,
-0.0127610417049336));
#37373=CARTESIAN_POINT('Ctrl Pts',(-0.0029605246994185,-0.0263281915842769,
-0.0126637845997177));
#37374=CARTESIAN_POINT('Ctrl Pts',(-0.00297482421323234,-0.0263227359100158,
-0.01256474343909));
#37375=CARTESIAN_POINT('Ctrl Pts',(-0.00298437329047243,-0.0263174422123873,
-0.0124699000564556));
#37376=CARTESIAN_POINT('Ctrl Pts',(-0.00298914782909248,-0.0263147953635731,
-0.0124224783651384));
#37377=CARTESIAN_POINT('Ctrl Pts',(-0.00299277570460114,-0.0263122594784373,
-0.0123761082719682));
#37378=CARTESIAN_POINT('Ctrl Pts',(-0.00299518340335414,-0.0263095726021238,
-0.0123231071556954));
#37379=CARTESIAN_POINT('Ctrl Pts',(-0.00299759110210715,-0.0263068857258102,
-0.0122701060394227));
#37380=CARTESIAN_POINT('Ctrl Pts',(-0.00299862475717886,-0.0263037826870209,
-0.012210477937357));
#37381=CARTESIAN_POINT('Ctrl Pts',(-0.00299887342984987,-0.0263018678103632,
-0.0121759532348433));
#37382=CARTESIAN_POINT('Ctrl Pts',(-0.00299912210252088,-0.0262999529337055,
-0.0121414285323296));
#37383=CARTESIAN_POINT('Ctrl Pts',(-0.00299875934617465,-0.0262995268874553,
-0.0121319906728096));
#37384=CARTESIAN_POINT('Ctrl Pts',(-0.00299832085105743,-0.0262987456299934,
-0.0121154106268001));
#37385=CARTESIAN_POINT('Ctrl Pts',(-0.00299788235594021,-0.0262979643725315,
-0.0120988305807907));
#37386=CARTESIAN_POINT('Ctrl Pts',(-0.00299730472817847,-0.0262967177950422,
-0.0120751157477882));
#37387=CARTESIAN_POINT('Ctrl Pts',(-0.00299645196421981,-0.0262955090939945,
-0.0120521389971071));
#37388=CARTESIAN_POINT('Ctrl Pts',(-0.00299474643630249,-0.0262930916918991,
-0.0120061854957447));
#37389=CARTESIAN_POINT('Ctrl Pts',(-0.00299201076742324,-0.0262909485423947,
-0.0119631737263696));
#37390=CARTESIAN_POINT('Ctrl Pts',(-0.00298806880567537,-0.0262887002297303,
-0.0119175451745365));
#37391=CARTESIAN_POINT('Ctrl Pts',(-0.00298018488217962,-0.0262842036044017,
-0.0118262880708702));
#37392=CARTESIAN_POINT('Ctrl Pts',(-0.00296737558619485,-0.0262791096282125,
-0.0117245846107055));
#37393=CARTESIAN_POINT('Ctrl Pts',(-0.00294746145973241,-0.0262737381999898,
-0.0116175990496526));
#37394=CARTESIAN_POINT('Ctrl Pts',(-0.00292754733326997,-0.0262683667717672,
-0.0115106134885997));
#37395=CARTESIAN_POINT('Ctrl Pts',(-0.00290056950786379,-0.0262627942966804,
-0.011398328512074));
#37396=CARTESIAN_POINT('Ctrl Pts',(-0.00286415384468825,-0.026256749612011,
-0.0112810074516751));
#37397=CARTESIAN_POINT('Ctrl Pts',(-0.00282773818151271,-0.0262507049273417,
-0.0111636863912763));
#37398=CARTESIAN_POINT('Ctrl Pts',(-0.00278187190752082,-0.0262441700152929,
-0.0110413300661203));
#37399=CARTESIAN_POINT('Ctrl Pts',(-0.00272405415663296,-0.0262368816762903,
-0.0109162086707602));
#37400=CARTESIAN_POINT('Ctrl Pts',(-0.00271912016742034,-0.0262362597118336,
-0.0109055311953224));
#37401=CARTESIAN_POINT('Ctrl Pts',(-0.00271410137325846,-0.0262356316298146,
-0.0108948360803448));
#37402=CARTESIAN_POINT('Ctrl Pts',(-0.00270899558262347,-0.0262349976164481,
-0.0108841250848099));
#37403=CARTESIAN_POINT('Ctrl Pts',(-0.00259443944523286,-0.0262207725673808,
-0.0106438076954377));
#37404=CARTESIAN_POINT('Ctrl Pts',(-0.00243528440089842,-0.0262035616951805,
-0.0103944168682738));
#37405=CARTESIAN_POINT('Ctrl Pts',(-0.00221968972734411,-0.0261854682004667,
-0.0101584152731379));
#37406=CARTESIAN_POINT('Ctrl Pts',(-0.00199448595479028,-0.0261665682749675,
-0.0099118950383051));
#37407=CARTESIAN_POINT('Ctrl Pts',(-0.00170740007538045,-0.0261471017547109,
-0.00968017773133318));
#37408=CARTESIAN_POINT('Ctrl Pts',(-0.0013576034578573,-0.0261275404938998,
-0.00950160676104891));
#37409=CARTESIAN_POINT('Ctrl Pts',(-0.00107674666081965,-0.0261118344727944,
-0.00935822952912178));
#37410=CARTESIAN_POINT('Ctrl Pts',(-0.000754970149059731,-0.0260959488223864,
-0.00924931751844913));
#37411=CARTESIAN_POINT('Ctrl Pts',(-0.000405204452938812,-0.0260772559187937,
-0.00920190336704683));
#37412=CARTESIAN_POINT('Ctrl Pts',(-0.000319350079617993,-0.0260726675113504,
-0.00919026496939855));
#37413=CARTESIAN_POINT('Ctrl Pts',(-0.000231832572911134,-0.0260679099616966,
-0.00918236687812477));
#37414=CARTESIAN_POINT('Ctrl Pts',(-0.000142935487738069,-0.0260629444083976,
-0.00917833097991991));
#37415=CARTESIAN_POINT('Ctrl Pts',(0.00030812312370331,-0.0260377494813456,
-0.00915785306844895));
#37416=CARTESIAN_POINT('Ctrl Pts',(0.000795119160569355,-0.026009515306029,
-0.0092408291296658));
#37417=CARTESIAN_POINT('Ctrl Pts',(0.00125831408289657,-0.0259833001929126,
-0.00945421707838627));
#37418=CARTESIAN_POINT('Ctrl Pts',(0.00162458284350649,-0.025962570740737,
-0.0096229523898924));
#37419=CARTESIAN_POINT('Ctrl Pts',(0.00197702463256216,-0.0259426559133689,
-0.00987425298737038));
#37420=CARTESIAN_POINT('Ctrl Pts',(0.00226508694472562,-0.0259194666608343,
-0.0102061852982747));
#37421=CARTESIAN_POINT('Ctrl Pts',(0.00234131723585644,-0.025913330059838,
-0.0102940249622207));
#37422=CARTESIAN_POINT('Ctrl Pts',(0.00241298674888928,-0.0259069641518263,
-0.0103875021935442));
#37423=CARTESIAN_POINT('Ctrl Pts',(0.00247967811919254,-0.0259002931583302,
-0.0104860271747369));
#37424=CARTESIAN_POINT('Ctrl Pts',(0.00276181762680004,-0.0258720713537445,
-0.0109028395682197));
#37425=CARTESIAN_POINT('Ctrl Pts',(0.00294915013904871,-0.0258425202835248,
-0.0114130346997862));
#37426=CARTESIAN_POINT('Ctrl Pts',(0.00299099925998867,-0.0258142681436675,
-0.0119611698913867));
#37427=CARTESIAN_POINT('Ctrl Pts',(0.00299642302465877,-0.0258106065862782,
-0.0120322097655791));
#37428=CARTESIAN_POINT('Ctrl Pts',(0.00299936426805713,-0.0258069668468853,
-0.012103825224218));
#37429=CARTESIAN_POINT('Ctrl Pts',(0.0029996789003323,-0.0258033546468746,
-0.0121758340213435));
#37430=CARTESIAN_POINT('',(0.00299998751882004,-0.0248036932032793,-0.0121758293984721));
#37431=CARTESIAN_POINT('Ctrl Pts',(0.00299999889294253,-0.0258037743898623,
-0.0121784305610133));
#37432=CARTESIAN_POINT('Ctrl Pts',(0.00299952054911593,-0.0257742293029132,
-0.0127352323200688));
#37433=CARTESIAN_POINT('Ctrl Pts',(0.00283972856505783,-0.0257446842159642,
-0.0132920158471201));
#37434=CARTESIAN_POINT('Ctrl Pts',(0.00254499247653757,-0.0257151391290152,
-0.0137642528881594));
#37435=CARTESIAN_POINT('Ctrl Pts',(0.00242406993537792,-0.0257030175492976,
-0.013957999447391));
#37436=CARTESIAN_POINT('Ctrl Pts',(0.00228103500614737,-0.0256908959695799,
-0.014137684814758));
#37437=CARTESIAN_POINT('Ctrl Pts',(0.00211982590390775,-0.0256787743898623,
-0.0142986670176993));
#37438=CARTESIAN_POINT('Ctrl Pts',(0.00173413343228542,-0.0256497735333579,
-0.0146838166331805));
#37439=CARTESIAN_POINT('Ctrl Pts',(0.00123888032829478,-0.0256207726768534,
-0.0149623095815553));
#37440=CARTESIAN_POINT('Ctrl Pts',(0.000707343059994884,-0.025591771820349,
-0.0150912719178145));
#37441=CARTESIAN_POINT('Ctrl Pts',(0.0004751999116223,-0.0255791060101868,
-0.0151475948222394));
#37442=CARTESIAN_POINT('Ctrl Pts',(0.000236507129008994,-0.0255664402000245,
-0.0151759836724882));
#37443=CARTESIAN_POINT('Ctrl Pts',(-1.64815128970163E-6,-0.0255537743898623,
-0.0151758528338243));
#37444=CARTESIAN_POINT('Ctrl Pts',(-0.00054896799349106,-0.0255246662835434,
-0.0151755521451443));
#37445=CARTESIAN_POINT('Ctrl Pts',(-0.00109801327074517,-0.0254955581772245,
-0.0150211395577944));
#37446=CARTESIAN_POINT('Ctrl Pts',(-0.00156617253887826,-0.0254664500709055,
-0.0147345841396303));
#37447=CARTESIAN_POINT('Ctrl Pts',(-0.00176815773010942,-0.0254538915105578,
-0.0146109511051568));
#37448=CARTESIAN_POINT('Ctrl Pts',(-0.00195524218533828,-0.02544133295021,
-0.014463383215985));
#37449=CARTESIAN_POINT('Ctrl Pts',(-0.00212215710272589,-0.0254287743898623,
-0.0142963365407599));
#37450=CARTESIAN_POINT('Ctrl Pts',(-0.00250895807067001,-0.0253996717585666,
-0.0139092302432509));
#37451=CARTESIAN_POINT('Ctrl Pts',(-0.00278805096283689,-0.0253705691272708,
-0.0134119508496134));
#37452=CARTESIAN_POINT('Ctrl Pts',(-0.00291657166754198,-0.0253414664959751,
-0.0128784269183515));
#37453=CARTESIAN_POINT('Ctrl Pts',(-0.00297205595222404,-0.0253289024606041,
-0.0126480967645078));
#37454=CARTESIAN_POINT('Ctrl Pts',(-0.0030000565339502,-0.0253163384252332,
-0.0124113703361084));
#37455=CARTESIAN_POINT('Ctrl Pts',(-0.00299999991383313,-0.0253037743898623,
-0.012175134258592));
#37456=CARTESIAN_POINT('Ctrl Pts',(-0.00299986876214958,-0.0252746717585666,
-0.0116279301748924));
#37457=CARTESIAN_POINT('Ctrl Pts',(-0.00284568929645957,-0.0252455691272708,
-0.0110789342839306));
#37458=CARTESIAN_POINT('Ctrl Pts',(-0.00255937922046653,-0.0252164664959751,
-0.0106107405092017));
#37459=CARTESIAN_POINT('Ctrl Pts',(-0.00243577493584797,-0.0252039024606041,
-0.0104086143479498));
#37460=CARTESIAN_POINT('Ctrl Pts',(-0.00228820817650185,-0.0251913384252332,
-0.0102213924515308));
#37461=CARTESIAN_POINT('Ctrl Pts',(-0.0021211404011013,-0.0251787743898623,
-0.0100543530158026));
#37462=CARTESIAN_POINT('Ctrl Pts',(-0.00173408111439472,-0.0251496662835434,
-0.00966735938588312));
#37463=CARTESIAN_POINT('Ctrl Pts',(-0.00123678155629453,-0.0251205581772245,
-0.00938808525837841));
#37464=CARTESIAN_POINT('Ctrl Pts',(-0.000703183699308903,-0.0250914500709055,
-0.00925942864583339));
#37465=CARTESIAN_POINT('Ctrl Pts',(-0.000472965325947317,-0.0250788915105578,
-0.00920392033433145));
#37466=CARTESIAN_POINT('Ctrl Pts',(-0.000236348792081367,-0.02506633295021,
-0.00917586983113488));
#37467=CARTESIAN_POINT('Ctrl Pts',(-2.10095426478409E-7,-0.0250537743898623,
-0.00917585329391478));
#37468=CARTESIAN_POINT('Ctrl Pts',(0.000545093209029396,-0.0250247735333579,
-0.00917581510533792));
#37469=CARTESIAN_POINT('Ctrl Pts',(0.00109237998997015,-0.0249957726768534,
-0.00932879021741214));
#37470=CARTESIAN_POINT('Ctrl Pts',(0.0015595447804611,-0.024966771820349,
-0.00961307743257935));
#37471=CARTESIAN_POINT('Ctrl Pts',(0.00176357394594232,-0.0249541060101868,
-0.00973723679657291));
#37472=CARTESIAN_POINT('Ctrl Pts',(0.00195247687430197,-0.0249414402000245,
-0.00988576529037574));
#37473=CARTESIAN_POINT('Ctrl Pts',(0.00212084323529318,-0.0249287743898623,
-0.0100540559420148));
#37474=CARTESIAN_POINT('Ctrl Pts',(0.00251358548478697,-0.0248992293029133,
-0.0104466215869831));
#37475=CARTESIAN_POINT('Ctrl Pts',(0.00279523648864188,-0.0248696842159643,
-0.0109522392104689));
#37476=CARTESIAN_POINT('Ctrl Pts',(0.0029217167302512,-0.0248401391290152,
-0.0114949925458995));
#37477=CARTESIAN_POINT('Ctrl Pts',(0.00297360827939497,-0.0248280175492976,
-0.0117176701042286));
#37478=CARTESIAN_POINT('Ctrl Pts',(0.00299991303547187,-0.0248158959695799,
-0.0119462727392586));
#37479=CARTESIAN_POINT('Ctrl Pts',(0.00299999978369675,-0.0248037743898623,
-0.0121747140677592));
#37480=CARTESIAN_POINT('',(0.00299999984621867,-0.0238037386203311,-0.0121751721745847));
#37481=CARTESIAN_POINT('Ctrl Pts',(0.00299999999993919,-0.0248037126098014,
-0.0121758723881634));
#37482=CARTESIAN_POINT('Ctrl Pts',(0.00299999645468512,-0.0247741731508083,
-0.0127326717795756));
#37483=CARTESIAN_POINT('Ctrl Pts',(0.00284068071006489,-0.0247446336918151,
-0.0132895892039848));
#37484=CARTESIAN_POINT('Ctrl Pts',(0.00254634976491414,-0.0247150942328219,
-0.013762076119177));
#37485=CARTESIAN_POINT('Ctrl Pts',(0.00242554000872495,-0.0247029695993176,
-0.0139560109736917));
#37486=CARTESIAN_POINT('Ctrl Pts',(0.00228258638271583,-0.0246908449658133,
-0.0141358911367041));
#37487=CARTESIAN_POINT('Ctrl Pts',(0.00212142859262928,-0.024678720332309,
-0.014297065375524));
#37488=CARTESIAN_POINT('Ctrl Pts',(0.00173603113214065,-0.0246497251285438,
-0.0146825021719953));
#37489=CARTESIAN_POINT('Ctrl Pts',(0.00124099384319939,-0.0246207299247786,
-0.0149613680577734));
#37490=CARTESIAN_POINT('Ctrl Pts',(0.000709559108885839,-0.0245917347210134,
-0.0150907333648799));
#37491=CARTESIAN_POINT('Ctrl Pts',(0.000477359067389681,-0.0245790658322812,
-0.015147257012543));
#37492=CARTESIAN_POINT('Ctrl Pts',(0.000238582482541089,-0.0245663969435489,
-0.0151758274351697));
#37493=CARTESIAN_POINT('Ctrl Pts',(3.25284021884075E-7,-0.0245537280548167,
-0.0151758532689232));
#37494=CARTESIAN_POINT('Ctrl Pts',(-0.00054698931659537,-0.0245246256066227,
-0.015175912613155));
#37495=CARTESIAN_POINT('Ctrl Pts',(-0.00109613181250209,-0.0244955231584287,
-0.0150218640939648));
#37496=CARTESIAN_POINT('Ctrl Pts',(-0.0015644771952416,-0.0244664207102346,
-0.0147356210700824));
#37497=CARTESIAN_POINT('Ctrl Pts',(-0.00176663160060002,-0.0244538590659312,
-0.0146120684731881));
#37498=CARTESIAN_POINT('Ctrl Pts',(-0.0019538881738259,-0.0244412974216278,
-0.0144645503382962));
#37499=CARTESIAN_POINT('Ctrl Pts',(-0.00212096854515054,-0.0244287357773243,
-0.0142975253701945));
#37500=CARTESIAN_POINT('Ctrl Pts',(-0.00250798270998806,-0.0243996387969876,
-0.0139106395377989));
#37501=CARTESIAN_POINT('Ctrl Pts',(-0.00278735326712094,-0.0243705418166509,
-0.0134135214976788));
#37502=CARTESIAN_POINT('Ctrl Pts',(-0.00291617434900536,-0.0243414448363141,
-0.012880074250605));
#37503=CARTESIAN_POINT('Ctrl Pts',(-0.00297181273367537,-0.0243288777241534,
-0.0126496760681051));
#37504=CARTESIAN_POINT('Ctrl Pts',(-0.00299994716922196,-0.0243163106119926,
-0.0124128605335314));
#37505=CARTESIAN_POINT('Ctrl Pts',(-0.00299999992525709,-0.0243037434998319,
-0.0121765229562029));
#37506=CARTESIAN_POINT('Ctrl Pts',(-0.00300012207275585,-0.0242746465194952,
-0.0116293240649705));
#37507=CARTESIAN_POINT('Ctrl Pts',(-0.00284619954974807,-0.0242455495391585,
-0.0110802609922032));
#37508=CARTESIAN_POINT('Ctrl Pts',(-0.00256011048884314,-0.0242164525588217,
-0.0106119369573015));
#37509=CARTESIAN_POINT('Ctrl Pts',(-0.00243654738109967,-0.024203885446661,
-0.0104096657729355));
#37510=CARTESIAN_POINT('Ctrl Pts',(-0.00228899402826749,-0.0241913183345003,
-0.0102223005924817));
#37511=CARTESIAN_POINT('Ctrl Pts',(-0.00212191554668422,-0.0241787512223395,
-0.0100551283131729));
#37512=CARTESIAN_POINT('Ctrl Pts',(-0.0017350014496016,-0.0241496487741455,
-0.00966799700282649));
#37513=CARTESIAN_POINT('Ctrl Pts',(-0.00123780898872271,-0.0241205463259515,
-0.00938854213547383));
#37514=CARTESIAN_POINT('Ctrl Pts',(-0.000704262897402285,-0.0240914438777575,
-0.00925968906427182));
#37515=CARTESIAN_POINT('Ctrl Pts',(-0.000473965563859015,-0.024078882233454,
-0.00920407152869351));
#37516=CARTESIAN_POINT('Ctrl Pts',(-0.000237254351499635,-0.0240663205891505,
-0.00917593331151893));
#37517=CARTESIAN_POINT('Ctrl Pts',(-1.01405525885435E-6,-0.0240537589448471,
-0.00917585345794278));
#37518=CARTESIAN_POINT('Ctrl Pts',(0.000544283627240826,-0.0240247637410819,
-0.00917566913727139));
#37519=CARTESIAN_POINT('Ctrl Pts',(0.00109160692055374,-0.0239957685373167,
-0.00932849457792729));
#37520=CARTESIAN_POINT('Ctrl Pts',(0.00155884545293593,-0.0239667733335515,
-0.0096126519964014));
#37521=CARTESIAN_POINT('Ctrl Pts',(0.00176299621614839,-0.0239541044448192,
-0.0097368090378984));
#37522=CARTESIAN_POINT('Ctrl Pts',(0.00195201430165641,-0.023941435556087,
-0.00988536040928045));
#37523=CARTESIAN_POINT('Ctrl Pts',(0.00212048137367313,-0.0239287666673547,
-0.0100536943047885));
#37524=CARTESIAN_POINT('Ctrl Pts',(0.00251328821496056,-0.0238992272083615,
-0.0104461906246009));
#37525=CARTESIAN_POINT('Ctrl Pts',(0.00279502498094163,-0.0238696877493684,
-0.0109517571981392));
#37526=CARTESIAN_POINT('Ctrl Pts',(0.00292159872971184,-0.0238401482903752,
-0.0114944863791241));
#37527=CARTESIAN_POINT('Ctrl Pts',(0.00297355162145094,-0.0238280236568709,
-0.0117172525581882));
#37528=CARTESIAN_POINT('Ctrl Pts',(0.00299989620579271,-0.0238158990233666,
-0.0119459534947592));
#37529=CARTESIAN_POINT('Ctrl Pts',(0.00299999969243972,-0.0238037743898623,
-0.0121744948456985));
#37530=CARTESIAN_POINT('',(0.00299999948987923,-0.0228038528083122,-0.0121770162025489));
#37531=CARTESIAN_POINT('Ctrl Pts',(0.00299999999999761,-0.0238037028507998,
-0.012175849503471));
#37532=CARTESIAN_POINT('Ctrl Pts',(0.00300000070212657,-0.0237742589851738,
-0.0127326399815581));
#37533=CARTESIAN_POINT('Ctrl Pts',(0.00284069411920419,-0.0237447999402777,
-0.0132895506791278));
#37534=CARTESIAN_POINT('Ctrl Pts',(0.00254637537593904,-0.0237153253373963,
-0.0137620350052812));
#37535=CARTESIAN_POINT('Ctrl Pts',(0.00242551065442886,-0.0237032213183679,
-0.0139560650757582));
#37536=CARTESIAN_POINT('Ctrl Pts',(0.00228248050278621,-0.0236911146756247,
-0.0141360271007935));
#37537=CARTESIAN_POINT('Ctrl Pts',(0.00212123065892674,-0.0236790053829392,
-0.0142972633109591));
#37538=CARTESIAN_POINT('Ctrl Pts',(0.00173579890898887,-0.0236500608223828,
-0.0146826624725959));
#37539=CARTESIAN_POINT('Ctrl Pts',(0.001240737142082,-0.0236211011215851,
-0.014961482382444));
#37540=CARTESIAN_POINT('Ctrl Pts',(0.000709290622295351,-0.0235921273550881,
-0.0150907987085384));
#37541=CARTESIAN_POINT('Ctrl Pts',(0.000476979877153939,-0.0235794620782749,
-0.0151473266392999));
#37542=CARTESIAN_POINT('Ctrl Pts',(0.000238088999641541,-0.0235667941137618,
-0.015175875228355));
#37543=CARTESIAN_POINT('Ctrl Pts',(-2.7631354590831E-7,-0.0235541235513023,
-0.0151758532738332));
#37544=CARTESIAN_POINT('Ctrl Pts',(-0.000547620793514525,-0.0235250288716799,
-0.015175802860935));
#37545=CARTESIAN_POINT('Ctrl Pts',(-0.00109675970552012,-0.0234959204937934,
-0.0150216279019523));
#37546=CARTESIAN_POINT('Ctrl Pts',(-0.00156506467060867,-0.0234667944331137,
-0.0147352619246643));
#37547=CARTESIAN_POINT('Ctrl Pts',(-0.00176725716029671,-0.0234542191431581,
-0.0146116223004317));
#37548=CARTESIAN_POINT('Ctrl Pts',(-0.00195453684989838,-0.0234416405569279,
-0.0144640045171204));
#37549=CARTESIAN_POINT('Ctrl Pts',(-0.00212162140575758,-0.0234290583537329,
-0.0142968725251864));
#37550=CARTESIAN_POINT('Ctrl Pts',(-0.0025083439476894,-0.0233999364425086,
-0.013910040190944));
#37551=CARTESIAN_POINT('Ctrl Pts',(-0.0027874958188367,-0.0233707951549935,
-0.013413089999592));
#37552=CARTESIAN_POINT('Ctrl Pts',(-0.00291622221040971,-0.023341649313097,
-0.0128798760273223));
#37553=CARTESIAN_POINT('Ctrl Pts',(-0.00297192792673784,-0.0233290365925742,
-0.0126491302888728));
#37554=CARTESIAN_POINT('Ctrl Pts',(-0.00300004532424149,-0.0233164230191599,
-0.0124119543162287));
#37555=CARTESIAN_POINT('Ctrl Pts',(-0.00299999994485589,-0.0233038097940137,
-0.012175278078183));
#37556=CARTESIAN_POINT('Ctrl Pts',(-0.00299989497433512,-0.0232746331801249,
-0.0116278042057919));
#37557=CARTESIAN_POINT('Ctrl Pts',(-0.00284559490133652,-0.0232454584297435,
-0.011078576309219));
#37558=CARTESIAN_POINT('Ctrl Pts',(-0.00255907619185309,-0.0232162965318514,
-0.0106102450838807));
#37559=CARTESIAN_POINT('Ctrl Pts',(-0.00243550316989592,-0.0232037192594804,
-0.0104082579086059));
#37560=CARTESIAN_POINT('Ctrl Pts',(-0.00228799832177968,-0.0231911443778289,
-0.0102211626319481));
#37561=CARTESIAN_POINT('Ctrl Pts',(-0.00212101326950556,-0.0231785727684926,
-0.0100542259133888));
#37562=CARTESIAN_POINT('Ctrl Pts',(-0.00173396160267819,-0.0231494332600034,
-0.00966728627841473));
#37563=CARTESIAN_POINT('Ctrl Pts',(-0.00123668829684548,-0.0231203113322811,
-0.00938805142639478));
#37564=CARTESIAN_POINT('Ctrl Pts',(-0.000703125086075461,-0.0230912040398712,
-0.00925941451412838));
#37565=CARTESIAN_POINT('Ctrl Pts',(-0.000472761265818371,-0.0230786370807152,
-0.0092038760325809));
#37566=CARTESIAN_POINT('Ctrl Pts',(-0.000235991961798253,-0.0230660728496497,
-0.00917583020279523));
#37567=CARTESIAN_POINT('Ctrl Pts',(2.93265437673792E-7,-0.0230535111096261,
-0.0091758533008922));
#37568=CARTESIAN_POINT('Ctrl Pts',(0.000545584674455736,-0.0230245215320833,
-0.0091759066059337));
#37569=CARTESIAN_POINT('Ctrl Pts',(0.00109283646594747,-0.0229955452213105,
-0.00932896713018142));
#37570=CARTESIAN_POINT('Ctrl Pts',(0.00155994875593833,-0.0229665829718963,
-0.00961332331037315));
#37571=CARTESIAN_POINT('Ctrl Pts',(0.00176405944180797,-0.0229539275468114,
-0.00973757637802705));
#37572=CARTESIAN_POINT('Ctrl Pts',(0.00195302501859612,-0.0229412748065526,
-0.0098862205247778));
#37573=CARTESIAN_POINT('Ctrl Pts',(0.00212142802901245,-0.0229286248174143,
-0.010054640633918));
#37574=CARTESIAN_POINT('Ctrl Pts',(0.0025140637145109,-0.0228991310622576,
-0.0104473161855042));
#37575=CARTESIAN_POINT('Ctrl Pts',(0.00279557606596665,-0.0228696522622051,
-0.0109530140335188));
#37576=CARTESIAN_POINT('Ctrl Pts',(0.00292190596310267,-0.0228401881371818,
-0.0114958050950414));
#37577=CARTESIAN_POINT('Ctrl Pts',(0.00297375919097428,-0.0228280943254753,
-0.0117185985052942));
#37578=CARTESIAN_POINT('Ctrl Pts',(0.00300000056297038,-0.0228160029861661,
-0.0119473153256647));
#37579=CARTESIAN_POINT('Ctrl Pts',(0.0029999999999909,-0.0228039140998865,
-0.0121758606765069));
#37580=CARTESIAN_POINT('',(0.00299999978565727,-0.0218037310910125,-0.0121750620270919));
#37581=CARTESIAN_POINT('Ctrl Pts',(0.00299999883722565,-0.0228037743898623,
-0.0121784946204567));
#37582=CARTESIAN_POINT('Ctrl Pts',(0.00299950860341255,-0.0227742284435262,
-0.0127352969505315));
#37583=CARTESIAN_POINT('Ctrl Pts',(0.00283970441390225,-0.02274468249719,
-0.0132920775528615));
#37584=CARTESIAN_POINT('Ctrl Pts',(0.00254495771088097,-0.0227151365508539,
-0.0137643085896206));
#37585=CARTESIAN_POINT('Ctrl Pts',(0.00242404290534297,-0.0227030158305234,
-0.0139580333145911));
#37586=CARTESIAN_POINT('Ctrl Pts',(0.00228102041420593,-0.0226908951101928,
-0.0141376991714502));
#37587=CARTESIAN_POINT('Ctrl Pts',(0.00211982731969915,-0.0226787743898623,
-0.0142986656038997));
#37588=CARTESIAN_POINT('Ctrl Pts',(0.001734134198291,-0.0226497726607727,
-0.0146838163819981));
#37589=CARTESIAN_POINT('Ctrl Pts',(0.00123888007405062,-0.0226207709316831,
-0.0149623098929398));
#37590=CARTESIAN_POINT('Ctrl Pts',(0.000707341766562069,-0.0225917692025935,
-0.0150912722316287));
#37591=CARTESIAN_POINT('Ctrl Pts',(0.000475221141499959,-0.0225791042650164,
-0.0151475895623728));
#37592=CARTESIAN_POINT('Ctrl Pts',(0.000236552172571135,-0.0225664393274394,
-0.015175978293945));
#37593=CARTESIAN_POINT('Ctrl Pts',(-1.58009018492896E-6,-0.0225537743898623,
-0.0151758528704439));
#37594=CARTESIAN_POINT('Ctrl Pts',(-0.00054890114122793,-0.0225246654112391,
-0.015175564598197));
#37595=CARTESIAN_POINT('Ctrl Pts',(-0.00109795087836807,-0.0224955564326158,
-0.0150211638189013));
#37596=CARTESIAN_POINT('Ctrl Pts',(-0.00156611716280598,-0.0224664474539926,
-0.0147346180339244));
#37597=CARTESIAN_POINT('Ctrl Pts',(-0.00176808529877214,-0.0224538897659491,
-0.0146110014472874));
#37598=CARTESIAN_POINT('Ctrl Pts',(-0.00195515614604609,-0.0224413320779057,
-0.0144634543840437));
#37599=CARTESIAN_POINT('Ctrl Pts',(-0.00212206229987348,-0.0224287743898623,
-0.0142964314142053));
#37600=CARTESIAN_POINT('Ctrl Pts',(-0.00250888140021627,-0.0223996708878047,
-0.0139093415828963));
#37601=CARTESIAN_POINT('Ctrl Pts',(-0.00278799673686266,-0.0223705673857471,
-0.0134120735635768));
#37602=CARTESIAN_POINT('Ctrl Pts',(-0.0029165409691721,-0.0223414638836895,
-0.0128785543432961));
#37603=CARTESIAN_POINT('Ctrl Pts',(-0.00297202990472548,-0.0223289007190805,
-0.0126482490771728));
#37604=CARTESIAN_POINT('Ctrl Pts',(-0.0030000408079041,-0.0223163375544714,
-0.0124115475875402));
#37605=CARTESIAN_POINT('Ctrl Pts',(-0.00299999995513309,-0.0223037743898623,
-0.0121753344402846));
#37606=CARTESIAN_POINT('Ctrl Pts',(-0.00299990531666084,-0.0222746708878047,
-0.0116281291754413));
#37607=CARTESIAN_POINT('Ctrl Pts',(-0.00284576185212074,-0.0222455673857471,
-0.0110791220651115));
#37608=CARTESIAN_POINT('Ctrl Pts',(-0.00255948205582041,-0.0222164638836896,
-0.010610908685004));
#37609=CARTESIAN_POINT('Ctrl Pts',(-0.00243590310652211,-0.0222039007190805,
-0.0104087941162889));
#37610=CARTESIAN_POINT('Ctrl Pts',(-0.00228836540196688,-0.0221913375544714,
-0.0102215793127615));
#37611=CARTESIAN_POINT('Ctrl Pts',(-0.00212132867023112,-0.0221787743898623,
-0.0100545412697026));
#37612=CARTESIAN_POINT('Ctrl Pts',(-0.00173430288455623,-0.0221496654112391,
-0.00966751244567895));
#37613=CARTESIAN_POINT('Ctrl Pts',(-0.00123702698233215,-0.0221205564326158,
-0.00938819396503985));
#37614=CARTESIAN_POINT('Ctrl Pts',(-0.000703439480540827,-0.0220914474539925,
-0.00925949032951444));
#37615=CARTESIAN_POINT('Ctrl Pts',(-0.000473248463601254,-0.0220788897659491,
-0.00920396725102037));
#37616=CARTESIAN_POINT('Ctrl Pts',(-0.000236658131907783,-0.0220663320779057,
-0.00917589602513529));
#37617=CARTESIAN_POINT('Ctrl Pts',(-5.42397702818636E-7,-0.0220537743898623,
-0.00917585333559064));
#37618=CARTESIAN_POINT('Ctrl Pts',(0.000544762162621619,-0.0220247726607727,
-0.00917575474494208));
#37619=CARTESIAN_POINT('Ctrl Pts',(0.00109206689317226,-0.0219957709316831,
-0.0093286699125783));
#37620=CARTESIAN_POINT('Ctrl Pts',(0.00155926371864595,-0.0219667692025935,
-0.00961290641709037));
#37621=CARTESIAN_POINT('Ctrl Pts',(0.00176328667922693,-0.0219541042650164,
-0.00973703134687119));
#37622=CARTESIAN_POINT('Ctrl Pts',(0.00195218903299633,-0.0219414393274394,
-0.00988552230538304));
#37623=CARTESIAN_POINT('Ctrl Pts',(0.00212056146838152,-0.0219287743898623,
-0.0100537743392011));
#37624=CARTESIAN_POINT('Ctrl Pts',(0.0025133563724309,-0.0218992284435262,
-0.0104462883592574));
#37625=CARTESIAN_POINT('Ctrl Pts',(0.00279507461672607,-0.0218696824971901,
-0.010951869259183));
#37626=CARTESIAN_POINT('Ctrl Pts',(0.00292162671273439,-0.0218401365508539,
-0.0114946063772537));
#37627=CARTESIAN_POINT('Ctrl Pts',(0.00297354255071463,-0.0218280158305234,
-0.0117172550190096));
#37628=CARTESIAN_POINT('Ctrl Pts',(0.00299987747078827,-0.0218158951101928,
-0.0119458309340674));
#37629=CARTESIAN_POINT('Ctrl Pts',(0.0029999995713889,-0.0218037743898623,
-0.0121742496449468));
#37630=CARTESIAN_POINT('',(0.00299999993086331,-0.0208037504150882,-0.0121753965937047));
#37631=CARTESIAN_POINT('Ctrl Pts',(0.00299999999992564,-0.0218036877921627,
-0.012175874409237));
#37632=CARTESIAN_POINT('Ctrl Pts',(0.00299999607956417,-0.0217741497906089,
-0.01273267331044));
#37633=CARTESIAN_POINT('Ctrl Pts',(0.00284068022618476,-0.0217446117890551,
-0.013289590216266));
#37634=CARTESIAN_POINT('Ctrl Pts',(0.00254634941007706,-0.0217150737875013,
-0.0137620766887938));
#37635=CARTESIAN_POINT('Ctrl Pts',(0.00242552952729006,-0.0217029487306259,
-0.0139560277027724));
#37636=CARTESIAN_POINT('Ctrl Pts',(0.00228256206844824,-0.0216908236737505,
-0.0141359216549807));
#37637=CARTESIAN_POINT('Ctrl Pts',(0.00212138778135082,-0.0216786986168751,
-0.0142971061901826));
#37638=CARTESIAN_POINT('Ctrl Pts',(0.00173598366932797,-0.0216497048681671,
-0.0146825348077372));
#37639=CARTESIAN_POINT('Ctrl Pts',(0.0012409420320321,-0.0216207111194592,
-0.01496139097265));
#37640=CARTESIAN_POINT('Ctrl Pts',(0.000709505757877311,-0.0215917173707512,
-0.015090746351413));
#37641=CARTESIAN_POINT('Ctrl Pts',(0.000477285674087594,-0.02157904806103,
-0.015147270375752));
#37642=CARTESIAN_POINT('Ctrl Pts',(0.000238488477075509,-0.0215663787513088,
-0.0151758364513004));
#37643=CARTESIAN_POINT('Ctrl Pts',(2.11868588605447E-7,-0.0215537094415876,
-0.0151758532790767));
#37644=CARTESIAN_POINT('Ctrl Pts',(-0.000547101720137076,-0.0215246084508768,
-0.0151758919319293));
#37645=CARTESIAN_POINT('Ctrl Pts',(-0.00109623758463809,-0.0214955074601659,
-0.015021823198552));
#37646=CARTESIAN_POINT('Ctrl Pts',(-0.00156457171055949,-0.0214664064694551,
-0.0147355633018756));
#37647=CARTESIAN_POINT('Ctrl Pts',(-0.00176673819564929,-0.0214538444017367,
-0.0146119930687235));
#37648=CARTESIAN_POINT('Ctrl Pts',(-0.00195400349499016,-0.0214412823340184,
-0.0144644538808624));
#37649=CARTESIAN_POINT('Ctrl Pts',(-0.0021210881422845,-0.0214287202663,
-0.0142974058059787));
#37650=CARTESIAN_POINT('Ctrl Pts',(-0.00250807980025495,-0.0213996247420099,
-0.0139104988548804));
#37651=CARTESIAN_POINT('Ctrl Pts',(-0.00278742215409447,-0.0213705292177197,
-0.0134133659977121));
#37652=CARTESIAN_POINT('Ctrl Pts',(-0.00291621343819134,-0.0213414336934296,
-0.0128799123628523));
#37653=CARTESIAN_POINT('Ctrl Pts',(-0.00297184360465812,-0.0213288661592906,
-0.0126494921545466));
#37654=CARTESIAN_POINT('Ctrl Pts',(-0.00299996491844838,-0.0213162986251515,
-0.0124126550628953));
#37655=CARTESIAN_POINT('Ctrl Pts',(-0.00299999996701662,-0.0213037310910125,
-0.012176298146413));
#37656=CARTESIAN_POINT('Ctrl Pts',(-0.003000081109145,-0.0212746355667223,
-0.0116291002372155));
#37657=CARTESIAN_POINT('Ctrl Pts',(-0.00284611797447065,-0.0212455400424322,
-0.0110800494869966));
#37658=CARTESIAN_POINT('Ctrl Pts',(-0.00255999463096865,-0.0212164445181421,
-0.0106117473152724));
#37659=CARTESIAN_POINT('Ctrl Pts',(-0.00243640638242635,-0.021203876984003,
-0.010409468659908));
#37660=CARTESIAN_POINT('Ctrl Pts',(-0.00228882502846644,-0.021191309449864,
-0.0102221002517993));
#37661=CARTESIAN_POINT('Ctrl Pts',(-0.00212171724469397,-0.0211787419157249,
-0.0100549299184073));
#37662=CARTESIAN_POINT('Ctrl Pts',(-0.00173476766417422,-0.0211496409250141,
-0.0096678354999363));
#37663=CARTESIAN_POINT('Ctrl Pts',(-0.00123755002938891,-0.0211205399343033,
-0.00938842730832361));
#37664=CARTESIAN_POINT('Ctrl Pts',(-0.000703992790271626,-0.0210914389435924,
-0.00925962384578264));
#37665=CARTESIAN_POINT('Ctrl Pts',(-0.000473671347403565,-0.0210788768758741,
-0.00920402306452828));
#37666=CARTESIAN_POINT('Ctrl Pts',(-0.00023693751233426,-0.0210663148081557,
-0.00917590674609835));
#37667=CARTESIAN_POINT('Ctrl Pts',(-6.77851118439549E-7,-0.0210537527404374,
-0.00917585336313846));
#37668=CARTESIAN_POINT('Ctrl Pts',(0.000544618783218096,-0.0210247589917294,
-0.00917573015315749));
#37669=CARTESIAN_POINT('Ctrl Pts',(0.00109192409600206,-0.0209957652430214,
-0.00932861635859259));
#37670=CARTESIAN_POINT('Ctrl Pts',(0.00155913031831126,-0.0209667714943134,
-0.00961282526280911));
#37671=CARTESIAN_POINT('Ctrl Pts',(0.00176328399273679,-0.0209541021845922,
-0.0097370151586831));
#37672=CARTESIAN_POINT('Ctrl Pts',(0.00195229978348282,-0.020941432874871,
-0.00988560171783371));
#37673=CARTESIAN_POINT('Ctrl Pts',(0.00212075858122446,-0.0209287635651498,
-0.0100539713293883));
#37674=CARTESIAN_POINT('Ctrl Pts',(0.00251351369882283,-0.0208992255635961,
-0.0104465185128695));
#37675=CARTESIAN_POINT('Ctrl Pts',(0.0027951843313585,-0.0208696875620423,
-0.0109521213124772));
#37676=CARTESIAN_POINT('Ctrl Pts',(0.00292168736193154,-0.0208401495604885,
-0.0114948665325536));
#37677=CARTESIAN_POINT('Ctrl Pts',(0.00297361560216193,-0.0208280245036131,
-0.0117176580660399));
#37678=CARTESIAN_POINT('Ctrl Pts',(0.00299993046755241,-0.0208158994467377,
-0.0119463820244118));
#37679=CARTESIAN_POINT('Ctrl Pts',(0.00299999986172769,-0.0208037743898623,
-0.0121749424441802));
#37680=CARTESIAN_POINT('',(0.00299999945013065,-0.0198038454750366,-0.0121771205057471));
#37681=CARTESIAN_POINT('Ctrl Pts',(0.00299999999999892,-0.0208037264403141,
-0.0121758507432291));
#37682=CARTESIAN_POINT('Ctrl Pts',(0.00300000047203861,-0.0207741929253612,
-0.0127326481792972));
#37683=CARTESIAN_POINT('Ctrl Pts',(0.00284068981401535,-0.0207446594104083,
-0.013289565089164));
#37684=CARTESIAN_POINT('Ctrl Pts',(0.00254636407823635,-0.0207151258954554,
-0.013762053141894));
#37685=CARTESIAN_POINT('Ctrl Pts',(0.00242552667548471,-0.0207030007130224,
-0.0139560362775241));
#37686=CARTESIAN_POINT('Ctrl Pts',(0.00228253446287072,-0.0206908755305894,
-0.0141359580207443));
#37687=CARTESIAN_POINT('Ctrl Pts',(0.00212133014721027,-0.0206787503481565,
-0.0142971638264218));
#37688=CARTESIAN_POINT('Ctrl Pts',(0.00173591719310115,-0.0206497610350512,
-0.0146825803429162));
#37689=CARTESIAN_POINT('Ctrl Pts',(0.00124087014846921,-0.0206207717219459,
-0.0149614226384336));
#37690=CARTESIAN_POINT('Ctrl Pts',(0.000709432384186756,-0.0205917824088407,
-0.0150907642101143));
#37691=CARTESIAN_POINT('Ctrl Pts',(0.000477170333426602,-0.0205791127836004,
-0.0151472922566818));
#37692=CARTESIAN_POINT('Ctrl Pts',(0.000238329566291121,-0.0205664431583602,
-0.0151758523684426));
#37693=CARTESIAN_POINT('Ctrl Pts',(1.15571610319707E-8,-0.02055377353312,
-0.0151758532865358));
#37694=CARTESIAN_POINT('Ctrl Pts',(-0.000547299870503991,-0.0205246769881148,
-0.0151758553949913));
#37695=CARTESIAN_POINT('Ctrl Pts',(-0.00109642372481938,-0.0204955804431096,
-0.0150217511609241));
#37696=CARTESIAN_POINT('Ctrl Pts',(-0.00156473780817212,-0.0204664838981044,
-0.014735461770619));
#37697=CARTESIAN_POINT('Ctrl Pts',(-0.00176693177040435,-0.0204539215047641,
-0.0146118567195891));
#37698=CARTESIAN_POINT('Ctrl Pts',(-0.00195421772447099,-0.0204413591114238,
-0.014464275218782));
#37699=CARTESIAN_POINT('Ctrl Pts',(-0.00212131380292897,-0.0204287967180835,
-0.0142971801707283));
#37700=CARTESIAN_POINT('Ctrl Pts',(-0.00250826281589996,-0.0203997056361836,
-0.0139102335438927));
#37701=CARTESIAN_POINT('Ctrl Pts',(-0.00278755190394519,-0.0203706145542837,
-0.0134130729604044));
#37702=CARTESIAN_POINT('Ctrl Pts',(-0.00291628702624431,-0.0203415234723838,
-0.0128796074912057));
#37703=CARTESIAN_POINT('Ctrl Pts',(-0.00297190285181329,-0.0203289556159382,
-0.0126491410734002));
#37704=CARTESIAN_POINT('Ctrl Pts',(-0.00299999945292661,-0.0203163877594927,
-0.0124122583918547));
#37705=CARTESIAN_POINT('Ctrl Pts',(-0.00299999999999197,-0.0203038199030471,
-0.0121758602290658));
#37706=CARTESIAN_POINT('Ctrl Pts',(-0.00300000126629566,-0.0202747288211472,
-0.0116286644248754));
#37707=CARTESIAN_POINT('Ctrl Pts',(-0.00284595912377596,-0.0202456377392472,
-0.0110796378325426));
#37708=CARTESIAN_POINT('Ctrl Pts',(-0.00255976915460028,-0.0202165466573473,
-0.0106113783346471));
#37709=CARTESIAN_POINT('Ctrl Pts',(-0.00243613007987847,-0.0202039788009018,
-0.0104090820374839));
#37710=CARTESIAN_POINT('Ctrl Pts',(-0.00228849159223828,-0.0201914109444562,
-0.0102217047082522));
#37711=CARTESIAN_POINT('Ctrl Pts',(-0.00212132362112505,-0.0201788430880106,
-0.0100545362205689));
#37712=CARTESIAN_POINT('Ctrl Pts',(-0.00173430373304865,-0.0201497465430054,
-0.00966751513655252));
#37713=CARTESIAN_POINT('Ctrl Pts',(-0.00123703629027194,-0.0201206499980002,
-0.00938819961622383));
#37714=CARTESIAN_POINT('Ctrl Pts',(-0.000703457073080728,-0.020091553452995,
-0.00925949457296804));
#37715=CARTESIAN_POINT('Ctrl Pts',(-0.000473084978959003,-0.0200789910596548,
-0.00920392634732584));
#37716=CARTESIAN_POINT('Ctrl Pts',(-0.000236303284987885,-0.0200664286663145,
-0.00917585346991708));
#37717=CARTESIAN_POINT('Ctrl Pts',(-2.32785436811739E-9,-0.0200538662729742,
-0.009175853286559));
#37718=CARTESIAN_POINT('Ctrl Pts',(0.00054529204781636,-0.0200248769598689,
-0.00917585286343704));
#37719=CARTESIAN_POINT('Ctrl Pts',(0.00109256110731081,-0.0199958876467636,
-0.00932886108422719));
#37720=CARTESIAN_POINT('Ctrl Pts',(0.00155970233578898,-0.0199668983336584,
-0.00961317331751507));
#37721=CARTESIAN_POINT('Ctrl Pts',(0.0017638639272547,-0.0199542287084181,
-0.00973743046820657));
#37722=CARTESIAN_POINT('Ctrl Pts',(0.00195287686596327,-0.0199415590831779,
-0.00988608946770726));
#37723=CARTESIAN_POINT('Ctrl Pts',(0.00212132032904437,-0.0199288894579377,
-0.0100545329284832));
#37724=CARTESIAN_POINT('Ctrl Pts',(0.00251397054265975,-0.0198993559220794,
-0.0104471831367251));
#37725=CARTESIAN_POINT('Ctrl Pts',(0.00279550710894889,-0.0198698223862211,
-0.0109528592737185));
#37726=CARTESIAN_POINT('Ctrl Pts',(0.00292186681724648,-0.0198402888503629,
-0.011495636922249));
#37727=CARTESIAN_POINT('Ctrl Pts',(0.00297374554685843,-0.0198281634478756,
-0.011718481808858));
#37728=CARTESIAN_POINT('Ctrl Pts',(0.00300000017425403,-0.0198160380453884,
-0.011947254496424));
#37729=CARTESIAN_POINT('Ctrl Pts',(0.00299999999999913,-0.0198039126429012,
-0.0121758555733571));
#37730=CARTESIAN_POINT('',(0.0029999996678785,-0.0188037207375212,-0.0121748645262654));
#37731=CARTESIAN_POINT('Ctrl Pts',(0.00299999886819319,-0.0198037743898623,
-0.0121784592104961));
#37732=CARTESIAN_POINT('Ctrl Pts',(0.0029995152061575,-0.0197742278626064,
-0.0127352619392769));
#37733=CARTESIAN_POINT('Ctrl Pts',(0.00283971737465793,-0.0197446813353506,
-0.0132920447572879));
#37734=CARTESIAN_POINT('Ctrl Pts',(0.00254497588675829,-0.0197151348080947,
-0.0137642794686071));
#37735=CARTESIAN_POINT('Ctrl Pts',(0.00242407139288802,-0.0197030146686839,
-0.0139579926074221));
#37736=CARTESIAN_POINT('Ctrl Pts',(0.00228106202287421,-0.0196908945292731,
-0.0141376490287441));
#37737=CARTESIAN_POINT('Ctrl Pts',(0.00211988397161103,-0.0196787743898623,
-0.0142986090301392));
#37738=CARTESIAN_POINT('Ctrl Pts',(0.00173420051625722,-0.0196497720709318,
-0.0146837707132921));
#37739=CARTESIAN_POINT('Ctrl Pts',(0.00123895300934861,-0.0196207697520013,
-0.0149622775982709));
#37740=CARTESIAN_POINT('Ctrl Pts',(0.000707417383176034,-0.0195917674330708,
-0.0150912538844143));
#37741=CARTESIAN_POINT('Ctrl Pts',(0.000475313460033195,-0.0195791030853346,
-0.0151475735373825));
#37742=CARTESIAN_POINT('Ctrl Pts',(0.000236661332504474,-0.0195664387375985,
-0.0151759684499085));
#37743=CARTESIAN_POINT('Ctrl Pts',(-1.45537485542859E-6,-0.0195537743898623,
-0.0151758529335388));
#37744=CARTESIAN_POINT('Ctrl Pts',(-0.000548777249974811,-0.0195246648215881,
-0.0151755874140092));
#37745=CARTESIAN_POINT('Ctrl Pts',(-0.00109783405214176,-0.0194955552533139,
-0.0150212090217193));
#37746=CARTESIAN_POINT('Ctrl Pts',(-0.00156601259674953,-0.0194664456850397,
-0.0147346820316721));
#37747=CARTESIAN_POINT('Ctrl Pts',(-0.00176797244701259,-0.0194538885866472,
-0.0146110818610263));
#37748=CARTESIAN_POINT('Ctrl Pts',(-0.00195503796625831,-0.0194413314882548,
-0.0144635537821148));
#37749=CARTESIAN_POINT('Ctrl Pts',(-0.00212194257711093,-0.0194287743898623,
-0.014296551213997));
#37750=CARTESIAN_POINT('Ctrl Pts',(-0.00250878408897936,-0.0193996702991963,
-0.0139094826626457));
#37751=CARTESIAN_POINT('Ctrl Pts',(-0.00278792764284432,-0.0193705662085304,
-0.0134122296558984));
#37752=CARTESIAN_POINT('Ctrl Pts',(-0.00291650177595357,-0.0193414621178644,
-0.0128787169937302));
#37753=CARTESIAN_POINT('Ctrl Pts',(-0.00297199989604426,-0.0193288995418637,
-0.0126484300061464));
#37754=CARTESIAN_POINT('Ctrl Pts',(-0.00300002398420702,-0.019316336965863,
-0.0124117461089284));
#37755=CARTESIAN_POINT('Ctrl Pts',(-0.00299999998451356,-0.0193037743898623,
-0.0121755484609993));
#37756=CARTESIAN_POINT('Ctrl Pts',(-0.00299994438371526,-0.0192746702991963,
-0.0116283423975273));
#37757=CARTESIAN_POINT('Ctrl Pts',(-0.00284583965861221,-0.0192455662085304,
-0.0110793236615489));
#37758=CARTESIAN_POINT('Ctrl Pts',(-0.00255959261512691,-0.0192164621178644,
-0.0106110895201743));
#37759=CARTESIAN_POINT('Ctrl Pts',(-0.00243603609243631,-0.0192038995418637,
-0.0104089795468838));
#37760=CARTESIAN_POINT('Ctrl Pts',(-0.00228852293779553,-0.019191336965863,
-0.0102217656692403));
#37761=CARTESIAN_POINT('Ctrl Pts',(-0.00212151157134427,-0.0191787743898623,
-0.010054724188023));
#37762=CARTESIAN_POINT('Ctrl Pts',(-0.00173451858726122,-0.0191496648215881,
-0.00966766142304171));
#37763=CARTESIAN_POINT('Ctrl Pts',(-0.00123726600657303,-0.0191205552533139,
-0.00938829991716738));
#37764=CARTESIAN_POINT('Ctrl Pts',(-0.000703688884394736,-0.0190914456850397,
-0.00925955049809815));
#37765=CARTESIAN_POINT('Ctrl Pts',(-0.000473517816241132,-0.0190788885866472,
-0.0092040114015373));
#37766=CARTESIAN_POINT('Ctrl Pts',(-0.000236945933484557,-0.0190663314882548,
-0.00917591996428969));
#37767=CARTESIAN_POINT('Ctrl Pts',(-8.45723782757253E-7,-0.0190537743898623,
-0.00917585340576622));
#37768=CARTESIAN_POINT('Ctrl Pts',(0.000544459677777046,-0.0190247720709318,
-0.00917569967984446));
#37769=CARTESIAN_POINT('Ctrl Pts',(0.0010917805481729,-0.0189957697520013,
-0.00932855996767236));
#37770=CARTESIAN_POINT('Ctrl Pts',(0.00155900648058052,-0.0189667674330708,
-0.00961274993446557));
#37771=CARTESIAN_POINT('Ctrl Pts',(0.00176302850011425,-0.0189541030853346,
-0.00973684623763436));
#37772=CARTESIAN_POINT('Ctrl Pts',(0.00195193435715708,-0.0189414387375985,
-0.00988530686974216));
#37773=CARTESIAN_POINT('Ctrl Pts',(0.00212031530797329,-0.0189287743898623,
-0.0100535283833507));
#37774=CARTESIAN_POINT('Ctrl Pts',(0.00251315609664262,-0.0188992278626065,
-0.0104459971974108));
#37775=CARTESIAN_POINT('Ctrl Pts',(0.00279493305266735,-0.0188696813353506,
-0.0109515458766621));
#37776=CARTESIAN_POINT('Ctrl Pts',(0.00292154795597086,-0.0188401348080948,
-0.0114942687056274));
#37777=CARTESIAN_POINT('Ctrl Pts',(0.00297348604893989,-0.018828014668684,
-0.0117168964375275));
#37778=CARTESIAN_POINT('Ctrl Pts',(0.00299984735059131,-0.0188158945292731,
-0.0119454535977987));
#37779=CARTESIAN_POINT('Ctrl Pts',(0.00299999933581561,-0.0188037743898623,
-0.0121738570135582));
#37780=CARTESIAN_POINT('',(0.00299995600267922,-0.0178036976750793,-0.0121755209840925));
#37781=CARTESIAN_POINT('Ctrl Pts',(0.00299999999994139,-0.0188036670851801,
-0.0121758720389726));
#37782=CARTESIAN_POINT('Ctrl Pts',(0.00299999651950407,-0.0187741306257539,
-0.0127326703103992));
#37783=CARTESIAN_POINT('Ctrl Pts',(0.00284068144842702,-0.0187445941663278,
-0.0132895868137558));
#37784=CARTESIAN_POINT('Ctrl Pts',(0.00254635158034459,-0.0187150577069016,
-0.0137620732048786));
#37785=CARTESIAN_POINT('Ctrl Pts',(0.00242551900903975,-0.0187029319706895,
-0.0139560451789696));
#37786=CARTESIAN_POINT('Ctrl Pts',(0.00228253407654152,-0.0186908062344774,
-0.0141359570825797));
#37787=CARTESIAN_POINT('Ctrl Pts',(0.00212133886195709,-0.0186786804982654,
-0.0142971551115586));
#37788=CARTESIAN_POINT('Ctrl Pts',(0.00173592684308017,-0.018649688294707,
-0.0146825738595526));
#37789=CARTESIAN_POINT('Ctrl Pts',(0.0012408800814106,-0.0186206960911486,
-0.0149614183555681));
#37790=CARTESIAN_POINT('Ctrl Pts',(0.00070944204344864,-0.0185917038875902,
-0.0150907618592216));
#37791=CARTESIAN_POINT('Ctrl Pts',(0.000477196304749861,-0.0185790338955104,
-0.0151472867509421));
#37792=CARTESIAN_POINT('Ctrl Pts',(0.000238372674535684,-0.0185663639034305,
-0.0151758476355391));
#37793=CARTESIAN_POINT('Ctrl Pts',(7.11305807639468E-8,-0.0185536939113506,
-0.0151758532857148));
#37794=CARTESIAN_POINT('Ctrl Pts',(-0.000547241156960315,-0.0185245944677076,
-0.0151758662625951));
#37795=CARTESIAN_POINT('Ctrl Pts',(-0.00109636875609812,-0.0184954950240646,
-0.0150217724696189));
#37796=CARTESIAN_POINT('Ctrl Pts',(-0.00156468889345413,-0.0184663955804216,
-0.0147354916724832));
#37797=CARTESIAN_POINT('Ctrl Pts',(-0.00176687110051442,-0.0184538328284263,
-0.0146118991151982));
#37798=CARTESIAN_POINT('Ctrl Pts',(-0.00195414785241674,-0.0184412700764311,
-0.0144643331888976));
#37799=CARTESIAN_POINT('Ctrl Pts',(-0.00212123826661812,-0.0184287073244359,
-0.0142972557038837));
#37800=CARTESIAN_POINT('Ctrl Pts',(-0.00250820164891467,-0.018399613345429,
-0.0139103222641914));
#37801=CARTESIAN_POINT('Ctrl Pts',(-0.00278750859192168,-0.0183705193664222,
-0.013413170836358));
#37802=CARTESIAN_POINT('Ctrl Pts',(-0.00291626247755638,-0.0183414253874153,
-0.0128797092107334));
#37803=CARTESIAN_POINT('Ctrl Pts',(-0.00297188246430367,-0.0183288571707839,
-0.0126492607982357));
#37804=CARTESIAN_POINT('Ctrl Pts',(-0.00299998730878829,-0.0183162889541526,
-0.0124123960596514));
#37805=CARTESIAN_POINT('Ctrl Pts',(-0.0029999999956791,-0.0183037207375212,
-0.0121760143001341));
#37806=CARTESIAN_POINT('Ctrl Pts',(-0.00300002936437523,-0.0182746267585143,
-0.0116288176571484));
#37807=CARTESIAN_POINT('Ctrl Pts',(-0.00284601496634515,-0.0182455327795075,
-0.0110797824871448));
#37808=CARTESIAN_POINT('Ctrl Pts',(-0.00255984835774281,-0.0182164388005006,
-0.010611507932948));
#37809=CARTESIAN_POINT('Ctrl Pts',(-0.00243622814310224,-0.0182038705838692,
-0.0104092194787386));
#37810=CARTESIAN_POINT('Ctrl Pts',(-0.00228861112392049,-0.0181913023672379,
-0.0102218466845278));
#37811=CARTESIAN_POINT('Ctrl Pts',(-0.0021214659707898,-0.0181787341506065,
-0.0100546785802265));
#37812=CARTESIAN_POINT('Ctrl Pts',(-0.00173447145069292,-0.0181496347069635,
-0.00966763092082484));
#37813=CARTESIAN_POINT('Ctrl Pts',(-0.00123722194394823,-0.0181205352633204,
-0.00938828187359959));
#37814=CARTESIAN_POINT('Ctrl Pts',(-0.000703650603191536,-0.0180914358196774,
-0.00925954126130631));
#37815=CARTESIAN_POINT('Ctrl Pts',(-0.000473298280723861,-0.0180788730676822,
-0.0092039616287953));
#37816=CARTESIAN_POINT('Ctrl Pts',(-0.000236535431579815,-0.0180663103156869,
-0.00917587305804289));
#37817=CARTESIAN_POINT('Ctrl Pts',(-2.50896571037858E-7,-0.0180537475636917,
-0.00917585329704962));
#37818=CARTESIAN_POINT('Ctrl Pts',(0.000545044381030049,-0.0180247553601333,
-0.009175807692811));
#37819=CARTESIAN_POINT('Ctrl Pts',(0.0010923268375626,-0.017995763156575,
-0.00932877105354029));
#37820=CARTESIAN_POINT('Ctrl Pts',(0.00155949201344859,-0.0179667709530166,
-0.00961304532262673));
#37821=CARTESIAN_POINT('Ctrl Pts',(0.00176364962659962,-0.0179541009609367,
-0.00973727709171541));
#37822=CARTESIAN_POINT('Ctrl Pts',(0.00195266270700665,-0.0179414309688569,
-0.00988590854610536));
#37823=CARTESIAN_POINT('Ctrl Pts',(0.00212111114414092,-0.017928760976777,
-0.0100543237642084));
#37824=CARTESIAN_POINT('Ctrl Pts',(0.00251380045266248,-0.0178992245173508,
-0.0104469356320686));
#37825=CARTESIAN_POINT('Ctrl Pts',(0.00279538695390489,-0.0178696880579247,
-0.0109525844923845));
#37826=CARTESIAN_POINT('Ctrl Pts',(0.00292180002846733,-0.0178401515984985,
-0.0114953500950532));
#37827=CARTESIAN_POINT('Ctrl Pts',(0.0029736969594361,-0.0178280258622864,
-0.0117181741115675));
#37828=CARTESIAN_POINT('Ctrl Pts',(0.00299997401495591,-0.0178159001260744,
-0.0119469275970063));
#37829=CARTESIAN_POINT('Ctrl Pts',(0.00299999998064488,-0.0178037743898623,
-0.0121755125069922));
#37830=CARTESIAN_POINT('',(-0.00267238707576395,-0.0173796339931718,-0.0135401565297772));
#37831=CARTESIAN_POINT('Ctrl Pts',(0.00299880969160871,-0.0178016980599612,
-0.0121757419446065));
#37832=CARTESIAN_POINT('Ctrl Pts',(0.00299841265092597,-0.0177739447125569,
-0.0126975268287903));
#37833=CARTESIAN_POINT('Ctrl Pts',(0.00286181894313852,-0.01774972903045,
-0.0132226923897836));
#37834=CARTESIAN_POINT('Ctrl Pts',(0.00260148942570033,-0.0177223184482828,
-0.0136736443513037));
#37835=CARTESIAN_POINT('Ctrl Pts',(0.00252897879046934,-0.0177146836677764,
-0.0137992498282018));
#37836=CARTESIAN_POINT('Ctrl Pts',(0.00244688739981009,-0.0177068010230323,
-0.0139192469917063));
#37837=CARTESIAN_POINT('Ctrl Pts',(0.00235675099364363,-0.0176985250299721,
-0.0140330646766062));
#37838=CARTESIAN_POINT('Ctrl Pts',(0.00194300311890452,-0.0176605362229444,
-0.0145555153404158));
#37839=CARTESIAN_POINT('Ctrl Pts',(0.00134957914778,-0.0176246399761912,
-0.0149356135552591));
#37840=CARTESIAN_POINT('Ctrl Pts',(0.000701575655805405,-0.0175919594685167,
-0.0150930770227462));
#37841=CARTESIAN_POINT('Ctrl Pts',(0.00052847864049833,-0.0175832297341754,
-0.0151351392285514));
#37842=CARTESIAN_POINT('Ctrl Pts',(0.000351920136921582,-0.0175739186146666,
-0.015162498550165));
#37843=CARTESIAN_POINT('Ctrl Pts',(0.000174231884956872,-0.0175642883153518,
-0.0151731005712262));
#37844=CARTESIAN_POINT('Ctrl Pts',(-0.000313271042439478,-0.0175378667649355,
-0.0152021881234221));
#37845=CARTESIAN_POINT('Ctrl Pts',(-0.000810188572686238,-0.0175090426645311,
-0.015104128674824));
#37846=CARTESIAN_POINT('Ctrl Pts',(-0.00125381412214389,-0.0174832309972516,
-0.0149001412679313));
#37847=CARTESIAN_POINT('Ctrl Pts',(-0.00170800994607117,-0.0174568043148811,
-0.0146912934491848));
#37848=CARTESIAN_POINT('Ctrl Pts',(-0.00211381185151582,-0.0174333575875628,
-0.0143671701585034));
#37849=CARTESIAN_POINT('Ctrl Pts',(-0.00241105511171453,-0.0174070539795054,
-0.013965019431062));
#37850=CARTESIAN_POINT('Ctrl Pts',(-0.00250995731168941,-0.0173983019401744,
-0.0138312112106877));
#37851=CARTESIAN_POINT('Ctrl Pts',(-0.00259702259284883,-0.0173892336148329,
-0.0136887408954094));
#37852=CARTESIAN_POINT('Ctrl Pts',(-0.00267238707576395,-0.0173796339931718,
-0.0135401565297772));
#37853=CARTESIAN_POINT('',(-0.000927050983124835,-0.0173787743898723,-0.0150290228354436));
#37854=CARTESIAN_POINT('Origin',(0.,-0.0173787743898623,-0.0121758532865581));
#37855=CARTESIAN_POINT('',(-0.00299905564929069,-0.0191797287809082,-0.012156770087783));
#37856=CARTESIAN_POINT('Ctrl Pts',(-0.000927050983124817,-0.0173787743898723,
-0.0150290228354436));
#37857=CARTESIAN_POINT('Ctrl Pts',(-0.000918484919008519,-0.0173792522203775,
-0.0150318061183941));
#37858=CARTESIAN_POINT('Ctrl Pts',(-0.0009099159702334,-0.0173797313630426,
-0.015034547752181));
#37859=CARTESIAN_POINT('Ctrl Pts',(-0.000891568346580233,-0.0173807595853773,
-0.015040327152537));
#37860=CARTESIAN_POINT('Ctrl Pts',(-0.000881795771413628,-0.0173813086359318,
-0.0150433506027228));
#37861=CARTESIAN_POINT('Ctrl Pts',(-0.000843717427209008,-0.017383452924518,
-0.0150549182603554));
#37862=CARTESIAN_POINT('Ctrl Pts',(-0.000815302129173545,-0.0173850636494666,
-0.015063093587522));
#37863=CARTESIAN_POINT('Ctrl Pts',(-0.000658439221454871,-0.0173939988708078,
-0.0151057241640584));
#37864=CARTESIAN_POINT('Ctrl Pts',(-0.000527936836835853,-0.0174015864401309,
-0.0151320272181851));
#37865=CARTESIAN_POINT('Ctrl Pts',(-0.000260662284274568,-0.0174170165196915,
-0.0151676306870811));
#37866=CARTESIAN_POINT('Ctrl Pts',(-0.000124114522098636,-0.0174248403265584,
-0.0151763991948485));
#37867=CARTESIAN_POINT('Ctrl Pts',(8.99157383655247E-5,-0.0174368109280743,
-0.0151755031371412));
#37868=CARTESIAN_POINT('Ctrl Pts',(0.000167233758914984,-0.0174410774295902,
-0.0151721873989718));
#37869=CARTESIAN_POINT('Ctrl Pts',(0.000277013241401311,-0.0174470435289978,
-0.0151632163817411));
#37870=CARTESIAN_POINT('Ctrl Pts',(0.000309640161404375,-0.0174488052436293,
-0.0151600110686811));
#37871=CARTESIAN_POINT('Ctrl Pts',(0.000366934073234336,-0.0174518790810126,
-0.0151534326366392));
#37872=CARTESIAN_POINT('Ctrl Pts',(0.000391623516384989,-0.0174531971911412,
-0.0151502860839234));
#37873=CARTESIAN_POINT('Ctrl Pts',(0.000443388102909554,-0.0174559476592967,
-0.0151430332172639));
#37874=CARTESIAN_POINT('Ctrl Pts',(0.000470452027768219,-0.0174573781020459,
-0.0151388626857293));
#37875=CARTESIAN_POINT('Ctrl Pts',(0.000542772580701761,-0.01746118163024,
-0.0151267022518846));
#37876=CARTESIAN_POINT('Ctrl Pts',(0.000587909812379087,-0.0174635354913767,
-0.0151180419295527));
#37877=CARTESIAN_POINT('Ctrl Pts',(0.00088264247281882,-0.0174787983870967,
-0.0150544386762684));
#37878=CARTESIAN_POINT('Ctrl Pts',(0.00112453661194926,-0.0174907069809869,
-0.0149688335306828));
#37879=CARTESIAN_POINT('Ctrl Pts',(0.00145117848234948,-0.017508005925314,
-0.0148038302623325));
#37880=CARTESIAN_POINT('Ctrl Pts',(0.00154686784903474,-0.017513259869844,
-0.014748668705615));
#37881=CARTESIAN_POINT('Ctrl Pts',(0.00169003181277015,-0.0175217048364162,
-0.014655260991457));
#37882=CARTESIAN_POINT('Ctrl Pts',(0.00173975149240897,-0.0175247559550493,
-0.0146206301572248));
#37883=CARTESIAN_POINT('Ctrl Pts',(0.00180432459532359,-0.0175289228850042,
-0.0145726859583269));
#37884=CARTESIAN_POINT('Ctrl Pts',(0.00182014527386188,-0.0175299607042177,
-0.0145606940030742));
#37885=CARTESIAN_POINT('Ctrl Pts',(0.00184617982711892,-0.017531698742836,
-0.014540550050632));
#37886=CARTESIAN_POINT('Ctrl Pts',(0.00185646174728182,-0.0175323931044592,
-0.014532486586037));
#37887=CARTESIAN_POINT('Ctrl Pts',(0.0018768074825597,-0.0175337836657031,
-0.0145163149273462));
#37888=CARTESIAN_POINT('Ctrl Pts',(0.00188687188825807,-0.017534479814909,
-0.01450820863589));
#37889=CARTESIAN_POINT('Ctrl Pts',(0.00191302623527904,-0.0175363103203988,
-0.0144868627602179));
#37890=CARTESIAN_POINT('Ctrl Pts',(0.00192903078585154,-0.0175374517634064,
-0.0144735204386002));
#37891=CARTESIAN_POINT('Ctrl Pts',(0.00199935852172301,-0.0175425574631231,
-0.014413638443835));
#37892=CARTESIAN_POINT('Ctrl Pts',(0.0020521426919352,-0.0175466303085446,
-0.0143653340052529));
#37893=CARTESIAN_POINT('Ctrl Pts',(0.00223175912897695,-0.0175612048398428,
-0.0141887563597442));
#37894=CARTESIAN_POINT('Ctrl Pts',(0.00234870794347416,-0.0175720046632656,
-0.0140509800559048));
#37895=CARTESIAN_POINT('Ctrl Pts',(0.00252958870975051,-0.0175903407089791,
-0.013794205611741));
#37896=CARTESIAN_POINT('Ctrl Pts',(0.00259921253975879,-0.0175979852034743,
-0.0136798428414295));
#37897=CARTESIAN_POINT('Ctrl Pts',(0.0026803422836706,-0.0176076617832214,
-0.0135240089192594));
#37898=CARTESIAN_POINT('Ctrl Pts',(0.00269892488473315,-0.0176099439778581,
-0.0134864115983019));
#37899=CARTESIAN_POINT('Ctrl Pts',(0.00272684224164531,-0.0176134812343224,
-0.0134268135134082));
#37900=CARTESIAN_POINT('Ctrl Pts',(0.00273671233177929,-0.0176147552824252,
-0.0134050708263808));
#37901=CARTESIAN_POINT('Ctrl Pts',(0.00275473905673241,-0.0176171279366588,
-0.013364066289527));
#37902=CARTESIAN_POINT('Ctrl Pts',(0.00276295581151654,-0.0176182286280351,
-0.0133448325960253));
#37903=CARTESIAN_POINT('Ctrl Pts',(0.00278102587221311,-0.0176206942546393,
-0.0133012792212089));
#37904=CARTESIAN_POINT('Ctrl Pts',(0.00279076266919065,-0.0176220550317912,
-0.0132769128764347));
#37905=CARTESIAN_POINT('Ctrl Pts',(0.00281516304515299,-0.0176255532327253,
-0.013213446928504));
#37906=CARTESIAN_POINT('Ctrl Pts',(0.00282933243217529,-0.0176276736171813,
-0.0131741627323976));
#37907=CARTESIAN_POINT('Ctrl Pts',(0.00289604662473854,-0.0176381471346402,
-0.0129763544027179));
#37908=CARTESIAN_POINT('Ctrl Pts',(0.00293611296146069,-0.0176460798742083,
-0.0128139252942959));
#37909=CARTESIAN_POINT('Ctrl Pts',(0.00298701088980831,-0.0176612196264104,
-0.0124952424427378));
#37910=CARTESIAN_POINT('Ctrl Pts',(0.00299955892181305,-0.0176684227891603,
-0.0123398182771641));
#37911=CARTESIAN_POINT('Ctrl Pts',(0.00300018665214758,-0.017679487081178,
-0.0121123592065175));
#37912=CARTESIAN_POINT('Ctrl Pts',(0.00299780893032342,-0.0176830553993994,
-0.0120406069738473));
#37913=CARTESIAN_POINT('Ctrl Pts',(0.00299147775181801,-0.0176877884040497,
-0.0119489977157236));
#37914=CARTESIAN_POINT('Ctrl Pts',(0.00298989362807892,-0.0176888326710539,
-0.0119289957613114));
#37915=CARTESIAN_POINT('Ctrl Pts',(0.00298698161741509,-0.0176905550568207,
-0.0118963868733524));
#37916=CARTESIAN_POINT('Ctrl Pts',(0.00298577427053765,-0.0176912264214951,
-0.0118837699860754));
#37917=CARTESIAN_POINT('Ctrl Pts',(0.00298331897577259,-0.0176925157476851,
-0.0118597201809043));
#37918=CARTESIAN_POINT('Ctrl Pts',(0.00298208522555795,-0.0176931327890869,
-0.0118482865752693));
#37919=CARTESIAN_POINT('Ctrl Pts',(0.0029786681784155,-0.0176947645310459,
-0.0118182402523259));
#37920=CARTESIAN_POINT('Ctrl Pts',(0.00297637619270419,-0.0176957849567514,
-0.0117996406827138));
#37921=CARTESIAN_POINT('Ctrl Pts',(0.002967501834458,-0.0176994867668378,
-0.011732790937164));
#37922=CARTESIAN_POINT('Ctrl Pts',(0.00295991940624405,-0.0177022149922086,
-0.0116846832711209));
#37923=CARTESIAN_POINT('Ctrl Pts',(0.00291460480321268,-0.0177165460313655,
-0.0114366054381575));
#37924=CARTESIAN_POINT('Ctrl Pts',(0.00285776866025242,-0.017728711700786,
-0.0112406708531797));
#37925=CARTESIAN_POINT('Ctrl Pts',(0.00272471409561269,-0.0177494102852254,
-0.0109113607472286));
#37926=CARTESIAN_POINT('Ctrl Pts',(0.00265730059788534,-0.0177580593755,
-0.0107752206813554));
#37927=CARTESIAN_POINT('Ctrl Pts',(0.00256047818768718,-0.0177684462594944,
-0.0106120774157992));
#37928=CARTESIAN_POINT('Ctrl Pts',(0.00254046792852701,-0.0177705050518907,
-0.0105797748407188));
#37929=CARTESIAN_POINT('Ctrl Pts',(0.00250674917800025,-0.0177738363525339,
-0.0105275841115992));
#37930=CARTESIAN_POINT('Ctrl Pts',(0.00249340504967478,-0.0177751216897858,
-0.0105074666353051));
#37931=CARTESIAN_POINT('Ctrl Pts',(0.00246694636720748,-0.0177776078628876,
-0.010468604379082));
#37932=CARTESIAN_POINT('Ctrl Pts',(0.00245385739440067,-0.017778809511288,
-0.0104498442667652));
#37933=CARTESIAN_POINT('Ctrl Pts',(0.00242228106103653,-0.0177816434925442,
-0.010405671973726));
#37934=CARTESIAN_POINT('Ctrl Pts',(0.00240360630183731,-0.0177832687574654,
-0.0103803967267592));
#37935=CARTESIAN_POINT('Ctrl Pts',(0.00233991100216624,-0.0177886509606342,
-0.0102969639869986));
#37936=CARTESIAN_POINT('Ctrl Pts',(0.00229314845641496,-0.0177923427698239,
-0.0102401674479122));
#37937=CARTESIAN_POINT('Ctrl Pts',(0.00209020256090864,-0.0178074448423757,
-0.010011364431285));
#37938=CARTESIAN_POINT('Ctrl Pts',(0.00191641050047461,-0.0178181970206191,
-0.00985608512780436));
#37939=CARTESIAN_POINT('Ctrl Pts',(0.00167661075217465,-0.0178324458720628,
-0.00968734163058456));
#37940=CARTESIAN_POINT('Ctrl Pts',(0.00162571692605577,-0.0178354452406854,
-0.00965379902379728));
#37941=CARTESIAN_POINT('Ctrl Pts',(0.00153927769305174,-0.0178405569903873,
-0.00960053344546228));
#37942=CARTESIAN_POINT('Ctrl Pts',(0.00150428872153922,-0.0178426307737637,
-0.0095799404885922));
#37943=CARTESIAN_POINT('Ctrl Pts',(0.00145382074309139,-0.0178456437713906,
-0.00955160022974656));
#37944=CARTESIAN_POINT('Ctrl Pts',(0.00143867467761251,-0.0178465507506309,
-0.00954326634511958));
#37945=CARTESIAN_POINT('Ctrl Pts',(0.00141219763905639,-0.017848142451736,
-0.00952899449583122));
#37946=CARTESIAN_POINT('Ctrl Pts',(0.00140089895638865,-0.0178488236499623,
-0.00952299713868346));
#37947=CARTESIAN_POINT('Ctrl Pts',(0.00137630459106438,-0.0178503112711572,
-0.00951014335386279));
#37948=CARTESIAN_POINT('Ctrl Pts',(0.00136299562904553,-0.0178511192026931,
-0.00950331391936947));
#37949=CARTESIAN_POINT('Ctrl Pts',(0.00132473402221249,-0.0178534490412603,
-0.00948404028108089));
#37950=CARTESIAN_POINT('Ctrl Pts',(0.00129965878469903,-0.0178549845503533,
-0.00947184433286688));
#37951=CARTESIAN_POINT('Ctrl Pts',(0.00109688320724374,-0.017867449195163,
-0.0093766915954745));
#37952=CARTESIAN_POINT('Ctrl Pts',(0.000911617884956722,-0.0178790952266145,
-0.00931099659349189));
#37953=CARTESIAN_POINT('Ctrl Pts',(0.000566779390770429,-0.0178999135766266,
-0.0092255827629516));
#37954=CARTESIAN_POINT('Ctrl Pts',(0.00040946355650682,-0.0179091110500029,
-0.00919966701156135));
#37955=CARTESIAN_POINT('Ctrl Pts',(0.000198575408085529,-0.0179208578909511,
-0.00918197345430626));
#37956=CARTESIAN_POINT('Ctrl Pts',(0.000146223533100969,-0.0179237288079131,
-0.00917896026468511));
#37957=CARTESIAN_POINT('Ctrl Pts',(6.69574811337146E-5,-0.017928008601673,
-0.00917648021046679));
#37958=CARTESIAN_POINT('Ctrl Pts',(4.00870642307179E-5,-0.0179294478222835,
-0.00917600074943157));
#37959=CARTESIAN_POINT('Ctrl Pts',(-6.76178468817044E-6,-0.0179319376254472,
-0.00917579440596316));
#37960=CARTESIAN_POINT('Ctrl Pts',(-2.67374854965956E-5,-0.0179329930704657,
-0.0091759059301255));
#37961=CARTESIAN_POINT('Ctrl Pts',(-7.20073707692166E-5,-0.0179353715193671,
-0.00917661088145549));
#37962=CARTESIAN_POINT('Ctrl Pts',(-9.72983143109419E-5,-0.0179366907629061,
-0.00917732478827978));
#37963=CARTESIAN_POINT('Ctrl Pts',(-0.000165862173926824,-0.0179402430927888,
-0.00918012859687431));
#37964=CARTESIAN_POINT('Ctrl Pts',(-0.000209104473442932,-0.017942457314688,
-0.00918283604053157));
#37965=CARTESIAN_POINT('Ctrl Pts',(-0.000516292156398082,-0.017958030295056,
-0.00920875972505409));
#37966=CARTESIAN_POINT('Ctrl Pts',(-0.000776179042377204,-0.0179702501749041,
-0.00926591360868667));
#37967=CARTESIAN_POINT('Ctrl Pts',(-0.001099977292886,-0.0179867437199379,
-0.00938365285892597));
#37968=CARTESIAN_POINT('Ctrl Pts',(-0.00117365291519255,-0.01799059922073,
-0.00941381222105218));
#37969=CARTESIAN_POINT('Ctrl Pts',(-0.0012902773268246,-0.0179969924597811,
-0.00946706213416999));
#37970=CARTESIAN_POINT('Ctrl Pts',(-0.00133401628003306,-0.0179994588246775,
-0.00948833302358071));
#37971=CARTESIAN_POINT('Ctrl Pts',(-0.00139340407198984,-0.0180029281642065,
-0.00951902113233563));
#37972=CARTESIAN_POINT('Ctrl Pts',(-0.00140951462523009,-0.018003881788604,
-0.00952753297119871));
#37973=CARTESIAN_POINT('Ctrl Pts',(-0.0014367034093368,-0.018005514062931,
-0.00954221623841134));
#37974=CARTESIAN_POINT('Ctrl Pts',(-0.00144782214192675,-0.0180061881575623,
-0.00954831226309777));
#37975=CARTESIAN_POINT('Ctrl Pts',(-0.00147104787132347,-0.0180076107277387,
-0.00956123832848776));
#37976=CARTESIAN_POINT('Ctrl Pts',(-0.00148314647888632,-0.0180083600106268,
-0.00956808226029));
#37977=CARTESIAN_POINT('Ctrl Pts',(-0.00151627684546927,-0.0180104336312767,
-0.00958712855101086));
#37978=CARTESIAN_POINT('Ctrl Pts',(-0.00153720807933166,-0.0180117680844417,
-0.00959950267479505));
#37979=CARTESIAN_POINT('Ctrl Pts',(-0.00168250846336647,-0.0180211906087799,
-0.0096878023381588));
#37980=CARTESIAN_POINT('Ctrl Pts',(-0.00180134236042741,-0.0180297104872719,
-0.00977244094249443));
#37981=CARTESIAN_POINT('Ctrl Pts',(-0.00200269531583522,-0.0180450840700167,
-0.0099392016808822));
#37982=CARTESIAN_POINT('Ctrl Pts',(-0.00208749953127519,-0.0180519094353813,
-0.010018135434828));
#37983=CARTESIAN_POINT('Ctrl Pts',(-0.00222794506239104,-0.0180636805546593,
-0.010164909089136));
#37984=CARTESIAN_POINT('Ctrl Pts',(-0.00228557395368082,-0.0180686726461414,
-0.0102306568271619));
#37985=CARTESIAN_POINT('Ctrl Pts',(-0.00237898341557835,-0.0180770229545888,
-0.0103471188508274));
#37986=CARTESIAN_POINT('Ctrl Pts',(-0.00241621117623581,-0.0180804314683752,
-0.0103965961251811));
#37987=CARTESIAN_POINT('Ctrl Pts',(-0.00246824428271427,-0.0180853183753977,
-0.0104703984040806));
#37988=CARTESIAN_POINT('Ctrl Pts',(-0.00248427532931604,-0.0180868425666843,
-0.0104938359384863));
#37989=CARTESIAN_POINT('Ctrl Pts',(-0.00251213837088896,-0.0180895261514575,
-0.0105358394932248));
#37990=CARTESIAN_POINT('Ctrl Pts',(-0.00252410312446807,-0.0180906904276781,
-0.0105543145454972));
#37991=CARTESIAN_POINT('Ctrl Pts',(-0.00254896817512699,-0.0180931362891017,
-0.0105936514145953));
#37992=CARTESIAN_POINT('Ctrl Pts',(-0.00256181817710261,-0.0180944159790963,
-0.0106145431969307));
#37993=CARTESIAN_POINT('Ctrl Pts',(-0.00259579213524361,-0.0180978440542813,
-0.010671327618906));
#37994=CARTESIAN_POINT('Ctrl Pts',(-0.00261642763928695,-0.01809997493894,
-0.0107075069656226));
#37995=CARTESIAN_POINT('Ctrl Pts',(-0.00275305708827867,-0.018114456124006,
-0.0109590852973342));
#37996=CARTESIAN_POINT('Ctrl Pts',(-0.00284307444529361,-0.0181258397605986,
-0.0111875306139982));
#37997=CARTESIAN_POINT('Ctrl Pts',(-0.00292821460363338,-0.0181419929030586,
-0.0115165882016262));
#37998=CARTESIAN_POINT('Ctrl Pts',(-0.00294766632742895,-0.0181465596277272,
-0.0116098739897278));
#37999=CARTESIAN_POINT('Ctrl Pts',(-0.002968497591926,-0.0181531232725227,
-0.0117406464368854));
#38000=CARTESIAN_POINT('Ctrl Pts',(-0.00297366409534073,-0.0181549895615279,
-0.0117774758223127));
#38001=CARTESIAN_POINT('Ctrl Pts',(-0.00298153752097113,-0.0181583223382188,
-0.011842346093858));
#38002=CARTESIAN_POINT('Ctrl Pts',(-0.00298453664821187,-0.0181597757640042,
-0.0118703472753936));
#38003=CARTESIAN_POINT('Ctrl Pts',(-0.00298849917548977,-0.0181620180776826,
-0.0119130067490887));
#38004=CARTESIAN_POINT('Ctrl Pts',(-0.00298974990498657,-0.0181627921163158,
-0.0119276374287722));
#38005=CARTESIAN_POINT('Ctrl Pts',(-0.00299186212529958,-0.0181642332051021,
-0.0119546838771571));
#38006=CARTESIAN_POINT('Ctrl Pts',(-0.00299275383806924,-0.0181648986253354,
-0.0119670966584653));
#38007=CARTESIAN_POINT('Ctrl Pts',(-0.00299464040581733,-0.018166449678184,
-0.0119958610623202));
#38008=CARTESIAN_POINT('Ctrl Pts',(-0.00299557859394014,-0.018167338284819,
-0.0120122158085731));
#38009=CARTESIAN_POINT('Ctrl Pts',(-0.00299823964601961,-0.0181703002598389,
-0.012066355772898));
#38010=CARTESIAN_POINT('Ctrl Pts',(-0.00299938179577923,-0.0181724015559035,
-0.0121041645983236));
#38011=CARTESIAN_POINT('Ctrl Pts',(-0.00300194485721393,-0.0181851748148728,
-0.0123311696858455));
#38012=CARTESIAN_POINT('Ctrl Pts',(-0.00298617943132953,-0.0181964320611897,
-0.0125201253721847));
#38013=CARTESIAN_POINT('Ctrl Pts',(-0.00293174299641538,-0.0182144740442399,
-0.0128231287328789));
#38014=CARTESIAN_POINT('Ctrl Pts',(-0.00290384614350085,-0.0182213533136839,
-0.012938587749154));
#38015=CARTESIAN_POINT('Ctrl Pts',(-0.0028469503417549,-0.0182323489592065,
-0.013124887673167));
#38016=CARTESIAN_POINT('Ctrl Pts',(-0.00282195737281311,-0.0182365687132353,
-0.0131968089616204));
#38017=CARTESIAN_POINT('Ctrl Pts',(-0.00278304908522534,-0.0182423732966641,
-0.0132963824760266));
#38018=CARTESIAN_POINT('Ctrl Pts',(-0.00277140287654923,-0.0182440305509258,
-0.0133248850819308));
#38019=CARTESIAN_POINT('Ctrl Pts',(-0.00275048100433672,-0.0182468750177217,
-0.0133739190084775));
#38020=CARTESIAN_POINT('Ctrl Pts',(-0.00274140919465408,-0.0182480688692432,
-0.0133945340871935));
#38021=CARTESIAN_POINT('Ctrl Pts',(-0.00272225480458288,-0.0182505109746674,
-0.0134367646827539));
#38022=CARTESIAN_POINT('Ctrl Pts',(-0.00271214486293597,-0.0182517582015689,
-0.0134583660762039));
#38023=CARTESIAN_POINT('Ctrl Pts',(-0.00268539964238647,-0.0182549540149564,
-0.0135137802720378));
#38024=CARTESIAN_POINT('Ctrl Pts',(-0.0026683827406809,-0.0182568895438479,
-0.0135474048048597));
#38025=CARTESIAN_POINT('Ctrl Pts',(-0.00258622891749262,-0.0182658076912017,
-0.0137024167360325));
#38026=CARTESIAN_POINT('Ctrl Pts',(-0.00251341106963634,-0.0182725228024711,
-0.0138195520979423));
#38027=CARTESIAN_POINT('Ctrl Pts',(-0.00239866513169428,-0.0182819081415633,
-0.0139785756081425));
#38028=CARTESIAN_POINT('Ctrl Pts',(-0.00236316238006915,-0.0182846775256849,
-0.0140248708305322));
#38029=CARTESIAN_POINT('Ctrl Pts',(-0.00221034248989368,-0.0182961565445621,
-0.0142125493788301));
#38030=CARTESIAN_POINT('Ctrl Pts',(-0.00208152600560481,-0.0183047973022683,
-0.0143440277435928));
#38031=CARTESIAN_POINT('Ctrl Pts',(-0.00191953404008343,-0.0183156265334936,
-0.0144815463149926));
#38032=CARTESIAN_POINT('Ctrl Pts',(-0.00189728718186802,-0.0183171134459348,
-0.0144998869582831));
#38033=CARTESIAN_POINT('Ctrl Pts',(-0.00186298687060158,-0.0183194114098442,
-0.0145273439042255));
#38034=CARTESIAN_POINT('Ctrl Pts',(-0.00185112261875409,-0.0183202072290333,
-0.0145366949238486));
#38035=CARTESIAN_POINT('Ctrl Pts',(-0.00182942020530571,-0.0183216657294489,
-0.0145535358958784));
#38036=CARTESIAN_POINT('Ctrl Pts',(-0.00181960566740642,-0.0183223264004514,
-0.0145610551813913));
#38037=CARTESIAN_POINT('Ctrl Pts',(-0.00179673602647957,-0.0183238683407411,
-0.0145783531715706));
#38038=CARTESIAN_POINT('Ctrl Pts',(-0.0017836474516084,-0.0183247525469609,
-0.0145880862335798));
#38039=CARTESIAN_POINT('Ctrl Pts',(-0.00174113920935269,-0.0183276280162323,
-0.0146191615462217));
#38040=CARTESIAN_POINT('Ctrl Pts',(-0.00171141181936689,-0.0183296447157395,
-0.0146400753451428));
#38041=CARTESIAN_POINT('Ctrl Pts',(-0.00163794353273847,-0.0183346284267124,
-0.0146897910780535));
#38042=CARTESIAN_POINT('Ctrl Pts',(-0.00159381474987995,-0.018337621505514,
-0.0147179973207889));
#38043=CARTESIAN_POINT('Ctrl Pts',(-0.00139266748649034,-0.0183511898749482,
-0.014839270112602));
#38044=CARTESIAN_POINT('Ctrl Pts',(-0.00122808894718745,-0.0183620645681737,
-0.0149190470496841));
#38045=CARTESIAN_POINT('Ctrl Pts',(-0.0009305144165387,-0.0183805181620509,
-0.015031109936399));
#38046=CARTESIAN_POINT('Ctrl Pts',(-0.00080065356400895,-0.0183882094964906,
-0.0150702113621561));
#38047=CARTESIAN_POINT('Ctrl Pts',(-0.000631988362923594,-0.0183976818669959,
-0.0151087698735885));
#38048=CARTESIAN_POINT('Ctrl Pts',(-0.000595240948658097,-0.0183997158351181,
-0.015116448019551));
#38049=CARTESIAN_POINT('Ctrl Pts',(-0.00053498935202105,-0.0184030034155253,
-0.0151278614301218));
#38050=CARTESIAN_POINT('Ctrl Pts',(-0.000511568514481902,-0.0184042697793336,
-0.0151320101473221));
#38051=CARTESIAN_POINT('Ctrl Pts',(-0.000465924026948051,-0.0184067159678558,
-0.0151395367991225));
#38052=CARTESIAN_POINT('Ctrl Pts',(-0.000443706927339776,-0.0184078966405567,
-0.015142944346944));
#38053=CARTESIAN_POINT('Ctrl Pts',(-0.000391012965124657,-0.0184106742353693,
-0.0151504211754909));
#38054=CARTESIAN_POINT('Ctrl Pts',(-0.000360507431336982,-0.0184122643203087,
-0.0151542722876984));
#38055=CARTESIAN_POINT('Ctrl Pts',(-0.000254320012048163,-0.0184177416490344,
-0.0151660223210573));
#38056=CARTESIAN_POINT('Ctrl Pts',(-0.000178398508522549,-0.0184215555378976,
-0.015171510919069));
#38057=CARTESIAN_POINT('Ctrl Pts',(1.62942335709118E-5,-0.0184311480379168,
-0.0151781568144488));
#38058=CARTESIAN_POINT('Ctrl Pts',(0.000135074762959189,-0.01843681900494,
-0.0151751613586717));
#38059=CARTESIAN_POINT('Ctrl Pts',(0.000442051908924212,-0.0184514360728539,
-0.0151491422132447));
#38060=CARTESIAN_POINT('Ctrl Pts',(0.000628778946377897,-0.0184602780448767,
-0.0151153227570962));
#38061=CARTESIAN_POINT('Ctrl Pts',(0.00084387579589751,-0.0184715422153384,
-0.0150549218703496));
#38062=CARTESIAN_POINT('Ctrl Pts',(0.000876537602384341,-0.0184732836978446,
-0.015045146565961));
#38063=CARTESIAN_POINT('Ctrl Pts',(0.000926185898403631,-0.018475988275298,
-0.0150293605970681));
#38064=CARTESIAN_POINT('Ctrl Pts',(0.000943297455501972,-0.01847693096182,
-0.0150237497328701));
#38065=CARTESIAN_POINT('Ctrl Pts',(0.000972338360798834,-0.0184785504433161,
-0.0150139368043969));
#38066=CARTESIAN_POINT('Ctrl Pts',(0.000984293785566394,-0.0184792228610794,
-0.0150098126517288));
#38067=CARTESIAN_POINT('Ctrl Pts',(0.00100948320279297,-0.0184806522551055,
-0.0150009446644592));
#38068=CARTESIAN_POINT('Ctrl Pts',(0.00102271031074457,-0.0184814101595314,
-0.0149961832733967));
#38069=CARTESIAN_POINT('Ctrl Pts',(0.00105923093844334,-0.0184835221054458,
-0.0149827461720772));
#38070=CARTESIAN_POINT('Ctrl Pts',(0.00108245037191541,-0.0184848867535847,
-0.01497387383062));
#38071=CARTESIAN_POINT('Ctrl Pts',(0.00113486118805761,-0.0184880125837716,
-0.0149530972130958));
#38072=CARTESIAN_POINT('Ctrl Pts',(0.0011639803617351,-0.0184897817333343,
-0.0149410193441623));
#38073=CARTESIAN_POINT('Ctrl Pts',(0.00125967264898238,-0.0184956912102496,
-0.0148995493637679));
#38074=CARTESIAN_POINT('Ctrl Pts',(0.00132536451254645,-0.0184999026308407,
-0.014868194905075));
#38075=CARTESIAN_POINT('Ctrl Pts',(0.00158795291398626,-0.018517207635624,
-0.0147309220473911));
#38076=CARTESIAN_POINT('Ctrl Pts',(0.00177388865768702,-0.0185305055021675,
-0.0146055260507263));
#38077=CARTESIAN_POINT('Ctrl Pts',(0.00200123488529625,-0.0185473586178457,
-0.0144120717906233));
#38078=CARTESIAN_POINT('Ctrl Pts',(0.0020564635410866,-0.0185515147533242,
-0.0143613905878732));
#38079=CARTESIAN_POINT('Ctrl Pts',(0.00213196541663141,-0.0185572852832821,
-0.0142867063771941));
#38080=CARTESIAN_POINT('Ctrl Pts',(0.00215384649450964,-0.0185589690811248,
-0.0142643749375242));
#38081=CARTESIAN_POINT('Ctrl Pts',(0.00219074231952359,-0.018561829142666,
-0.0142255230393797));
#38082=CARTESIAN_POINT('Ctrl Pts',(0.00220592876916227,-0.0185630126606279,
-0.0142091698649165));
#38083=CARTESIAN_POINT('Ctrl Pts',(0.00223674179715954,-0.0185654277426806,
-0.0141752379965831));
#38084=CARTESIAN_POINT('Ctrl Pts',(0.00225234698640823,-0.0185666583781259,
-0.0141576419181095));
#38085=CARTESIAN_POINT('Ctrl Pts',(0.00229153807264962,-0.0185697696352363,
-0.0141123899465485));
#38086=CARTESIAN_POINT('Ctrl Pts',(0.00231483156736769,-0.0185716384107584,
-0.0140844852400283));
#38087=CARTESIAN_POINT('Ctrl Pts',(0.00241967713240745,-0.0185801526549903,
-0.0139541405956519));
#38088=CARTESIAN_POINT('Ctrl Pts',(0.00249497823526368,-0.0185865557142784,
-0.0138468504000259));
#38089=CARTESIAN_POINT('Ctrl Pts',(0.00262320306556077,-0.0185983866296428,
-0.0136360620766611));
#38090=CARTESIAN_POINT('Ctrl Pts',(0.0026775968038788,-0.0186038335245203,
-0.0135337485845328));
#38091=CARTESIAN_POINT('Ctrl Pts',(0.00278676418642777,-0.0186162568771403,
-0.0132961936593528));
#38092=CARTESIAN_POINT('Ctrl Pts',(0.00283786115975335,-0.0186232481531158,
-0.0131595975329385));
#38093=CARTESIAN_POINT('Ctrl Pts',(0.0028856883177898,-0.0186319709246532,
-0.0129964609092769));
#38094=CARTESIAN_POINT('Ctrl Pts',(0.00289225916303313,-0.0186332346704168,
-0.0129729924207941));
#38095=CARTESIAN_POINT('Ctrl Pts',(0.00290214124299736,-0.018635246142386,
-0.0129359657142127));
#38096=CARTESIAN_POINT('Ctrl Pts',(0.00290564515702325,-0.0186359835285071,
-0.0129224595436406));
#38097=CARTESIAN_POINT('Ctrl Pts',(0.00291215593926266,-0.0186374019374999,
-0.0128966229168957));
#38098=CARTESIAN_POINT('Ctrl Pts',(0.00291517896912859,-0.018638082072318,
-0.0128842970960091));
#38099=CARTESIAN_POINT('Ctrl Pts',(0.0029223603674028,-0.0186397511791331,
-0.0128541919052441));
#38100=CARTESIAN_POINT('Ctrl Pts',(0.00292643476657426,-0.0186407446570823,
-0.0128363931585568));
#38101=CARTESIAN_POINT('Ctrl Pts',(0.00294084312829566,-0.0186444331823331,
-0.01277069978802));
#38102=CARTESIAN_POINT('Ctrl Pts',(0.00295016532942999,-0.018647176504052,
-0.0127225933296855));
#38103=CARTESIAN_POINT('Ctrl Pts',(0.00297169507633421,-0.0186545373187582,
-0.0125948088881133));
#38104=CARTESIAN_POINT('Ctrl Pts',(0.00298187662224434,-0.0186592188106461,
-0.0125148311418218));
#38105=CARTESIAN_POINT('Ctrl Pts',(0.0030112364308428,-0.0186791542371746,
-0.012175618893272));
#38106=CARTESIAN_POINT('Ctrl Pts',(0.00299990864153989,-0.018694548752928,
-0.0119148251489048));
#38107=CARTESIAN_POINT('Ctrl Pts',(0.00294753764037032,-0.0187112975705394,
-0.0116155455238202));
#38108=CARTESIAN_POINT('Ctrl Pts',(0.00293903254977725,-0.0187136866274807,
-0.0115725201473627));
#38109=CARTESIAN_POINT('Ctrl Pts',(0.00292412827011347,-0.0187174102377501,
-0.0115049463195372));
#38110=CARTESIAN_POINT('Ctrl Pts',(0.00291835610990155,-0.0187187641205232,
-0.0114802672259961));
#38111=CARTESIAN_POINT('Ctrl Pts',(0.00290697187285675,-0.0187212789467455,
-0.0114342321352796));
#38112=CARTESIAN_POINT('Ctrl Pts',(0.00290143545285589,-0.0187224421853027,
-0.0114128593486722));
#38113=CARTESIAN_POINT('Ctrl Pts',(0.00288844917822966,-0.0187250427038151,
-0.0113649138084039));
#38114=CARTESIAN_POINT('Ctrl Pts',(0.00288086754053546,-0.0187264756892957,
-0.0113383786469758));
#38115=CARTESIAN_POINT('Ctrl Pts',(0.00285659772999105,-0.0187308177926663,
-0.0112576689825859));
#38116=CARTESIAN_POINT('Ctrl Pts',(0.00283873902202718,-0.018733689646804,
-0.0112038582843998));
#38117=CARTESIAN_POINT('Ctrl Pts',(0.00279302483538531,-0.018740368606869,
-0.0110781498884607));
#38118=CARTESIAN_POINT('Ctrl Pts',(0.00276390157584005,-0.0187441375966111,
-0.0110067555537347));
#38119=CARTESIAN_POINT('Ctrl Pts',(0.00267922964590745,-0.0187540270429248,
-0.0108200938288052));
#38120=CARTESIAN_POINT('Ctrl Pts',(0.00261900554806964,-0.0187600454289708,
-0.0107071239595497));
#38121=CARTESIAN_POINT('Ctrl Pts',(0.00247794000393196,-0.0187727852683669,
-0.0104789386038199));
#38122=CARTESIAN_POINT('Ctrl Pts',(0.00239584016960181,-0.0187795034837786,
-0.0103648731580879));
#38123=CARTESIAN_POINT('Ctrl Pts',(0.00228623916622762,-0.0187882134594537,
-0.0102331563447409));
#38124=CARTESIAN_POINT('Ctrl Pts',(0.00226604413571959,-0.0187898091581789,
-0.0102096374371148));
#38125=CARTESIAN_POINT('Ctrl Pts',(0.00223532869343492,-0.0187922298034257,
-0.0101749683862035));
#38126=CARTESIAN_POINT('Ctrl Pts',(0.00222508083600044,-0.0187930364100857,
-0.010163578453037));
#38127=CARTESIAN_POINT('Ctrl Pts',(0.00220635798974131,-0.0187945093161124,
-0.010143086926589));
#38128=CARTESIAN_POINT('Ctrl Pts',(0.0021979130327767,-0.0187951734715535,
-0.0101339588377981));
#38129=CARTESIAN_POINT('Ctrl Pts',(0.00217846153041869,-0.0187967027674732,
-0.0101131943481031));
#38130=CARTESIAN_POINT('Ctrl Pts',(0.00216741838784637,-0.0187975705464111,
-0.0101015934076861));
#38131=CARTESIAN_POINT('Ctrl Pts',(0.00213212446576222,-0.018800340932359,
-0.0100651063398975));
#38132=CARTESIAN_POINT('Ctrl Pts',(0.0021075346904506,-0.0188022666079202,
-0.0100405536034004));
#38133=CARTESIAN_POINT('Ctrl Pts',(0.00204708265341822,-0.0188069776428102,
-0.00998225417201123));
#38134=CARTESIAN_POINT('Ctrl Pts',(0.00201080556407585,-0.0188097857947129,
-0.00994895296830683));
#38135=CARTESIAN_POINT('Ctrl Pts',(0.00185370416222843,-0.0188218106573141,
-0.00981170852525162));
#38136=CARTESIAN_POINT('Ctrl Pts',(0.00172551869541643,-0.0188312773247858,
-0.00971658829210029));
#38137=CARTESIAN_POINT('Ctrl Pts',(0.00145250779188687,-0.0188500958157585,
-0.00954589848615459));
#38138=CARTESIAN_POINT('Ctrl Pts',(0.00130783607067975,-0.0188594072479526,
-0.00947103943413225));
#38139=CARTESIAN_POINT('Ctrl Pts',(0.00112237747470937,-0.0188704236631417,
-0.00939345459053829));
#38140=CARTESIAN_POINT('Ctrl Pts',(0.00108668060028056,-0.0188725052929899,
-0.00937931986860307));
#38141=CARTESIAN_POINT('Ctrl Pts',(0.00102828336085335,-0.0188758493200226,
-0.00935748369149285));
#38142=CARTESIAN_POINT('Ctrl Pts',(0.00100574551628953,-0.0188771253297842,
-0.00934936255668477));
#38143=CARTESIAN_POINT('Ctrl Pts',(0.000961960825911773,-0.018879576829045,
-0.00933417551063117));
#38144=CARTESIAN_POINT('Ctrl Pts',(0.000940727461419175,-0.0188807533529384,
-0.00932707581329203));
#38145=CARTESIAN_POINT('Ctrl Pts',(0.000890637345740944,-0.0188835008336519,
-0.00931094854172757));
#38146=CARTESIAN_POINT('Ctrl Pts',(0.000861719411946828,-0.0188850653682551,
-0.00930211811798917));
#38147=CARTESIAN_POINT('Ctrl Pts',(0.000762870334084337,-0.0188903442350807,
-0.0092735597379996));
#38148=CARTESIAN_POINT('Ctrl Pts',(0.000692355999364761,-0.018893992442587,
-0.00925593493532533));
#38149=CARTESIAN_POINT('Ctrl Pts',(0.000513155010783287,-0.0189030321890254,
-0.00921800204322305));
#38150=CARTESIAN_POINT('Ctrl Pts',(0.000403856658224679,-0.0189083326624521,
-0.00920110728498425));
#38151=CARTESIAN_POINT('Ctrl Pts',(0.0001270887854547,-0.0189215519504282,
-0.00917386488608472));
#38152=CARTESIAN_POINT('Ctrl Pts',(-4.07659455317399E-5,-0.0189293781093705,
-0.00917145355426854));
#38153=CARTESIAN_POINT('Ctrl Pts',(-0.000270584063945929,-0.0189407192226307,
-0.0091874208534722));
#38154=CARTESIAN_POINT('Ctrl Pts',(-0.000333079584316126,-0.0189438694486538,
-0.0091937397458152));
#38155=CARTESIAN_POINT('Ctrl Pts',(-0.000415685638258841,-0.0189481735699036,
-0.00920472096704819));
#38156=CARTESIAN_POINT('Ctrl Pts',(-0.000436015680736784,-0.0189492442070633,
-0.00920763629799436));
#38157=CARTESIAN_POINT('Ctrl Pts',(-0.00046801067381927,-0.0189509492867855,
-0.00921256017412424));
#38158=CARTESIAN_POINT('Ctrl Pts',(-0.000479696754563788,-0.0189515763108307,
-0.00921442946089919));
#38159=CARTESIAN_POINT('Ctrl Pts',(-0.000504139411264349,-0.0189528972621672,
-0.00921848774041169));
#38160=CARTESIAN_POINT('Ctrl Pts',(-0.000516893311202831,-0.0189535919756741,
-0.00922069021066716));
#38161=CARTESIAN_POINT('Ctrl Pts',(-0.000548935157146933,-0.0189553503885891,
-0.00922643727933196));
#38162=CARTESIAN_POINT('Ctrl Pts',(-0.000568203185416867,-0.0189564197285708,
-0.00923008858277464));
#38163=CARTESIAN_POINT('Ctrl Pts',(-0.000646208974282892,-0.0189607935692511,
-0.00924566451245364));
#38164=CARTESIAN_POINT('Ctrl Pts',(-0.000704616025598163,-0.0189641713644821,
-0.00925915864126414));
#38165=CARTESIAN_POINT('Ctrl Pts',(-0.000870190856513358,-0.0189739695716574,
-0.00930267580600117));
#38166=CARTESIAN_POINT('Ctrl Pts',(-0.000976144742771533,-0.0189805075363449,
-0.00933692383123003));
#38167=CARTESIAN_POINT('Ctrl Pts',(-0.00127914553528562,-0.0189996083383301,
-0.00945383667015244));
#38168=CARTESIAN_POINT('Ctrl Pts',(-0.00146959805965129,-0.0190120839588966,
-0.00955175462680121));
#38169=CARTESIAN_POINT('Ctrl Pts',(-0.00168543698521664,-0.0190263354624648,
-0.00969365596630042));
#38170=CARTESIAN_POINT('Ctrl Pts',(-0.00172226538993981,-0.0190287743245499,
-0.00971906603763104));
#38171=CARTESIAN_POINT('Ctrl Pts',(-0.00177919376477361,-0.019032556896985,
-0.00976025375169827));
#38172=CARTESIAN_POINT('Ctrl Pts',(-0.00179968303464,-0.0190339209860502,
-0.0097754798583545));
#38173=CARTESIAN_POINT('Ctrl Pts',(-0.00183750224205979,-0.0190364445993303,
-0.00980434078001927));
#38174=CARTESIAN_POINT('Ctrl Pts',(-0.0018548808948331,-0.0190376065826385,
-0.00981790863944317));
#38175=CARTESIAN_POINT('Ctrl Pts',(-0.00189344946752091,-0.0190401914225397,
-0.00984871018639379));
#38176=CARTESIAN_POINT('Ctrl Pts',(-0.00191455691922286,-0.0190416102010078,
-0.0098660442551721));
#38177=CARTESIAN_POINT('Ctrl Pts',(-0.0019775878686017,-0.0190458622552884,
-0.0099192648663602));
#38178=CARTESIAN_POINT('Ctrl Pts',(-0.00201876174228229,-0.0190486605388356,
-0.00995602298230598));
#38179=CARTESIAN_POINT('Ctrl Pts',(-0.00216649610805912,-0.0190588145612551,
-0.0100954255653499));
#38180=CARTESIAN_POINT('Ctrl Pts',(-0.00226644036631344,-0.0190658996174339,
-0.0102047780845042));
#38181=CARTESIAN_POINT('Ctrl Pts',(-0.0024739548282348,-0.0190818273861348,
-0.0104685820346359));
#38182=CARTESIAN_POINT('Ctrl Pts',(-0.00257588632720747,-0.0190905920918294,
-0.0106266519879419));
#38183=CARTESIAN_POINT('Ctrl Pts',(-0.0026800459744835,-0.0191019664444451,
-0.0108272155986657));
#38184=CARTESIAN_POINT('Ctrl Pts',(-0.00269706224485031,-0.0191039242798969,
-0.0108615759057136));
#38185=CARTESIAN_POINT('Ctrl Pts',(-0.00272002108258788,-0.0191067237943501,
-0.0109102604567793));
#38186=CARTESIAN_POINT('Ctrl Pts',(-0.0027265188216796,-0.0191075352134371,
-0.0109243202283929));
#38187=CARTESIAN_POINT('Ctrl Pts',(-0.00273810155966704,-0.019109017945812,
-0.0109499012349391));
#38188=CARTESIAN_POINT('Ctrl Pts',(-0.00274322351575125,-0.0191096871003701,
-0.0109614055421165));
#38189=CARTESIAN_POINT('Ctrl Pts',(-0.00275383034873737,-0.0191111021260923,
-0.0109856388059851));
#38190=CARTESIAN_POINT('Ctrl Pts',(-0.00275929963053183,-0.0191118488245443,
-0.0109983739308514));
#38191=CARTESIAN_POINT('Ctrl Pts',(-0.00277395699684311,-0.0191138962234051,
-0.0110331663131432));
#38192=CARTESIAN_POINT('Ctrl Pts',(-0.00278296994112422,-0.0191152065238506,
-0.0110552957576228));
#38193=CARTESIAN_POINT('Ctrl Pts',(-0.00283795498855828,-0.0191235216434375,
-0.0111950566839909));
#38194=CARTESIAN_POINT('Ctrl Pts',(-0.00287672125310937,-0.0191308512173997,
-0.0113153767157011));
#38195=CARTESIAN_POINT('Ctrl Pts',(-0.00296744218820184,-0.0191524718374996,
-0.0116727849040339));
#38196=CARTESIAN_POINT('Ctrl Pts',(-0.00299839357336558,-0.0191668035180019,
-0.01191420638761));
#38197=CARTESIAN_POINT('Ctrl Pts',(-0.00299993908917108,-0.019180238095247,
-0.0121567362453802));
#38198=CARTESIAN_POINT('Ctrl Pts',(-0.0029990259773704,-0.0191797116746683,
-0.012156771224441));
#38199=CARTESIAN_POINT('Ctrl Pts',(-0.00299900717703148,-0.0191799305018243,
-0.0121612117764821));
#38200=CARTESIAN_POINT('Ctrl Pts',(-0.00299898627533192,-0.0191801491278106,
-0.0121655716153771));
#38201=CARTESIAN_POINT('Ctrl Pts',(-0.00299896195254882,-0.0191803670938455,
-0.012169853924649));
#38202=CARTESIAN_POINT('',(-0.00299993908917192,-0.0191802380952497,-0.0121567362453771));
#38203=CARTESIAN_POINT('Ctrl Pts',(-0.00299999393119832,-0.0191809619683288,
-0.0121698189717546));
#38204=CARTESIAN_POINT('Ctrl Pts',(-0.00299998955652076,-0.0191808417663619,
-0.0121676440543882));
#38205=CARTESIAN_POINT('Ctrl Pts',(-0.00299998281669984,-0.0191807214956478,
-0.0121654691307674));
#38206=CARTESIAN_POINT('Ctrl Pts',(-0.00299996455983385,-0.0191804802010913,
-0.0121611081457004));
#38207=CARTESIAN_POINT('Ctrl Pts',(-0.00299995301874857,-0.0191803591796904,
-0.0121589221414168));
#38208=CARTESIAN_POINT('Ctrl Pts',(-0.00299993908917192,-0.0191802380952497,
-0.0121567362453771));
#38209=CARTESIAN_POINT('Origin',(0.,-0.0357900992552775,-0.0121758532865581));
#38210=CARTESIAN_POINT('',(-0.00249999995746914,-0.0332901205213028,-0.0121755333059438));
#38211=CARTESIAN_POINT('',(-0.00249999938712155,-0.0322901101338213,-0.0121771834348536));
#38212=CARTESIAN_POINT('Ctrl Pts',(-0.00249999991496748,-0.0332900992552675,
-0.012175201241613));
#38213=CARTESIAN_POINT('Ctrl Pts',(-0.00249987325125826,-0.0332591766194273,
-0.0116895610036931));
#38214=CARTESIAN_POINT('Ctrl Pts',(-0.00235395428532161,-0.0332282539835869,
-0.0112039832265026));
#38215=CARTESIAN_POINT('Ctrl Pts',(-0.00208658183779019,-0.0331973313477467,
-0.0107988361355378));
#38216=CARTESIAN_POINT('Ctrl Pts',(-0.00199368361807678,-0.0331865873169203,
-0.01065806828971));
#38217=CARTESIAN_POINT('Ctrl Pts',(-0.00188657164099081,-0.0331758432860939,
-0.010526864134928));
#38218=CARTESIAN_POINT('Ctrl Pts',(-0.0017675670555371,-0.0331650992552675,
-0.0104078864587641));
#38219=CARTESIAN_POINT('Ctrl Pts',(-0.00143136654560736,-0.0331347462345938,
-0.0100717619704172));
#38220=CARTESIAN_POINT('Ctrl Pts',(-0.00099492120557128,-0.0331043932139202,
-0.00983328515454348));
#38221=CARTESIAN_POINT('Ctrl Pts',(-0.000528748028399615,-0.0330740401932465,
-0.00973240786616019));
#38222=CARTESIAN_POINT('Ctrl Pts',(-0.000354988772124477,-0.0330627265472535,
-0.00969480732742718));
#38223=CARTESIAN_POINT('Ctrl Pts',(-0.000177363740756044,-0.0330514129012605,
-0.00967585943472476));
#38224=CARTESIAN_POINT('Ctrl Pts',(-8.66816036824776E-8,-0.0330400992552675,
-0.00967585328806084));
#38225=CARTESIAN_POINT('Ctrl Pts',(0.000477283201102462,-0.0330096339830744,
-0.00967583673638604));
#38226=CARTESIAN_POINT('Ctrl Pts',(0.000956188035358496,-0.0329791687108814,
-0.00981686733479447));
#38227=CARTESIAN_POINT('Ctrl Pts',(0.0013580605767814,-0.0329487034386883,
-0.0100768841420035));
#38228=CARTESIAN_POINT('Ctrl Pts',(0.0015058200596463,-0.0329375020442147,
-0.0101724864661468));
#38229=CARTESIAN_POINT('Ctrl Pts',(0.00164330762013163,-0.0329263006497411,
-0.0102836723408953));
#38230=CARTESIAN_POINT('Ctrl Pts',(0.00176744445112735,-0.0329150992552675,
-0.0104077638905775));
#38231=CARTESIAN_POINT('Ctrl Pts',(0.00210500519603208,-0.0328846397129049,
-0.0107452015036623));
#38232=CARTESIAN_POINT('Ctrl Pts',(0.00234395658822882,-0.0328541801705422,
-0.0111834403202244));
#38233=CARTESIAN_POINT('Ctrl Pts',(0.00244435914715829,-0.0328237206281795,
-0.0116513455557251));
#38234=CARTESIAN_POINT('Ctrl Pts',(0.0024813007382356,-0.0328125135038755,
-0.0118235041546403));
#38235=CARTESIAN_POINT('Ctrl Pts',(0.00249994188581591,-0.0328013063795715,
-0.0119994240830024));
#38236=CARTESIAN_POINT('Ctrl Pts',(0.00249999986374028,-0.0327900992552675,
-0.0121750278784132));
#38237=CARTESIAN_POINT('Ctrl Pts',(0.00250015744038486,-0.0327596397129048,
-0.0126522967210052));
#38238=CARTESIAN_POINT('Ctrl Pts',(0.00235932583811129,-0.0327291801705421,
-0.0131311592784346));
#38239=CARTESIAN_POINT('Ctrl Pts',(0.00209951830117244,-0.0326987206281795,
-0.0135330647303066));
#38240=CARTESIAN_POINT('Ctrl Pts',(0.00200392607831762,-0.0326875135038754,
-0.0136809397148994));
#38241=CARTESIAN_POINT('Ctrl Pts',(0.0018927299026143,-0.0326763063795715,
-0.0138185381949725));
#38242=CARTESIAN_POINT('Ctrl Pts',(0.00176861158204399,-0.0326650992552675,
-0.0139427752066949));
#38243=CARTESIAN_POINT('Ctrl Pts',(0.00143121027214934,-0.0326346339830744,
-0.014280499164769));
#38244=CARTESIAN_POINT('Ctrl Pts',(0.000992947727101739,-0.0326041687108814,
-0.0145196020115855));
#38245=CARTESIAN_POINT('Ctrl Pts',(0.000524972426846048,-0.0325737034386883,
-0.0146201126735814));
#38246=CARTESIAN_POINT('Ctrl Pts',(0.000352908448265819,-0.0325625020442147,
-0.0146570681803854));
#38247=CARTESIAN_POINT('Ctrl Pts',(0.000177082255337662,-0.0325513006497411,
-0.0146757429836459));
#38248=CARTESIAN_POINT('Ctrl Pts',(1.56413461402208E-6,-0.0325400992552675,
-0.0146758527972546));
#38249=CARTESIAN_POINT('Ctrl Pts',(-0.000474046751108256,-0.0325097462345939,
-0.0146761503650925));
#38250=CARTESIAN_POINT('Ctrl Pts',(-0.000951423590060535,-0.0324793932139203,
-0.0145364034942133));
#38251=CARTESIAN_POINT('Ctrl Pts',(-0.00135248331656414,-0.0324490401932467,
-0.0142784204979489));
#38252=CARTESIAN_POINT('Ctrl Pts',(-0.00150197248327778,-0.0324377265472536,
-0.0141822610967693));
#38253=CARTESIAN_POINT('Ctrl Pts',(-0.00164100269364965,-0.0324264129012606,
-0.0140701896281456));
#38254=CARTESIAN_POINT('Ctrl Pts',(-0.00176639923486798,-0.0324150992552675,
-0.0139449869002396));
#38255=CARTESIAN_POINT('Ctrl Pts',(-0.00210913504099933,-0.0323841766194273,
-0.0136027808277133));
#38256=CARTESIAN_POINT('Ctrl Pts',(-0.00235017420041792,-0.0323532539835871,
-0.013157143854241));
#38257=CARTESIAN_POINT('Ctrl Pts',(-0.00244840903005507,-0.0323223313477468,
-0.0126811187826538));
#38258=CARTESIAN_POINT('Ctrl Pts',(-0.00248254059772946,-0.0323115873169204,
-0.0125157244718416));
#38259=CARTESIAN_POINT('Ctrl Pts',(-0.00249984350998278,-0.0323008432860939,
-0.012346891169886));
#38260=CARTESIAN_POINT('Ctrl Pts',(-0.00249999893936607,-0.0322900992552675,
-0.0121781561475047));
#38261=CARTESIAN_POINT('',(-0.00249999997357178,-0.0312909865556403,-0.0121755454777103));
#38262=CARTESIAN_POINT('Ctrl Pts',(-0.00249999999999967,-0.0322901250241527,
-0.0121758520066069));
#38263=CARTESIAN_POINT('Ctrl Pts',(-0.00249999975397871,-0.0322616273783385,
-0.0116953239977705));
#38264=CARTESIAN_POINT('Ctrl Pts',(-0.00235838357544941,-0.0322315631162502,
-0.0112391117930363));
#38265=CARTESIAN_POINT('Ctrl Pts',(-0.00213070189368216,-0.0322030988071068,
-0.0108681417586364));
#38266=CARTESIAN_POINT('Ctrl Pts',(-0.00204892585140747,-0.0321928753296195,
-0.0107349010825299));
#38267=CARTESIAN_POINT('Ctrl Pts',(-0.00195630643732137,-0.0321828582490487,
-0.010612003978176));
#38268=CARTESIAN_POINT('Ctrl Pts',(-0.00185518017705755,-0.0321731942832527,
-0.0105000530267859));
#38269=CARTESIAN_POINT('Ctrl Pts',(-0.00184583808252193,-0.0321723015212558,
-0.0104897109418664));
#38270=CARTESIAN_POINT('Ctrl Pts',(-0.00183642818598577,-0.0321714118294668,
-0.010479467651635));
#38271=CARTESIAN_POINT('Ctrl Pts',(-0.0018269522946202,-0.0321705251244434,
-0.0104693230895847));
#38272=CARTESIAN_POINT('Ctrl Pts',(-0.0014935199541142,-0.0321393242463525,
-0.0101123619407762));
#38273=CARTESIAN_POINT('Ctrl Pts',(-0.00107750042637275,-0.0321118214492774,
-0.00987938050070426));
#38274=CARTESIAN_POINT('Ctrl Pts',(-0.000663016412915333,-0.0320843813491235,
-0.009765374239521));
#38275=CARTESIAN_POINT('Ctrl Pts',(-0.00060675889316707,-0.0320806569305062,
-0.00974990027844722));
#38276=CARTESIAN_POINT('Ctrl Pts',(-0.00055051895230167,-0.032076933666915,
-0.00973655052044115));
#38277=CARTESIAN_POINT('Ctrl Pts',(-0.000494472428651543,-0.0320732024682493,
-0.00972524172670137));
#38278=CARTESIAN_POINT('Ctrl Pts',(-0.000166245003803277,-0.032051351305146,
-0.0096590136003947));
#38279=CARTESIAN_POINT('Ctrl Pts',(0.000155346586532059,-0.0320307859803488,
-0.00966315997919557));
#38280=CARTESIAN_POINT('Ctrl Pts',(0.000446820137915882,-0.0320118112729673,
-0.00971610700607452));
#38281=CARTESIAN_POINT('Ctrl Pts',(0.000582229204164707,-0.0320029962453373,
-0.00974070446075365));
#38282=CARTESIAN_POINT('Ctrl Pts',(0.000711629629261853,-0.0319945245091002,
-0.00977576702176651));
#38283=CARTESIAN_POINT('Ctrl Pts',(0.00083393264289702,-0.031986426622681,
-0.00981904265625477));
#38284=CARTESIAN_POINT('Ctrl Pts',(0.00121949789381606,-0.0319608977046573,
-0.00995547086333002));
#38285=CARTESIAN_POINT('Ctrl Pts',(0.00152880138072454,-0.031938621727944,
-0.0101708635989568));
#38286=CARTESIAN_POINT('Ctrl Pts',(0.00176119446046587,-0.0319172141729503,
-0.0104015381870269));
#38287=CARTESIAN_POINT('Ctrl Pts',(0.0019935875402072,-0.0318958066179567,
-0.0106322127750971));
#38288=CARTESIAN_POINT('Ctrl Pts',(0.00215013969655286,-0.0318767874994582,
-0.0108768456008528));
#38289=CARTESIAN_POINT('Ctrl Pts',(0.0022561209758157,-0.0318610351411786,
-0.0110988583271992));
#38290=CARTESIAN_POINT('Ctrl Pts',(0.00227592622398728,-0.0318580914197291,
-0.0111403469483324));
#38291=CARTESIAN_POINT('Ctrl Pts',(0.00229396174659566,-0.0318552393346794,
-0.0111810688164089));
#38292=CARTESIAN_POINT('Ctrl Pts',(0.00231042100019264,-0.031852479018487,
-0.0112208900402136));
#38293=CARTESIAN_POINT('Ctrl Pts',(0.002382038035103,-0.0318404684093821,
-0.0113941590137179));
#38294=CARTESIAN_POINT('Ctrl Pts',(0.00242408001468336,-0.0318301952319051,
-0.0115499894070535));
#38295=CARTESIAN_POINT('Ctrl Pts',(0.00245053904127961,-0.031821670397811,
-0.011681021590762));
#38296=CARTESIAN_POINT('Ctrl Pts',(0.00246680900318903,-0.0318164283785896,
-0.0117615947981735));
#38297=CARTESIAN_POINT('Ctrl Pts',(0.00247711855042881,-0.0318121280969749,
-0.0118327269911542));
#38298=CARTESIAN_POINT('Ctrl Pts',(0.00248410590563771,-0.0318084305852773,
-0.0118943966299023));
#38299=CARTESIAN_POINT('Ctrl Pts',(0.0024910932608466,-0.0318047330735796,
-0.0119560662686504));
#38300=CARTESIAN_POINT('Ctrl Pts',(0.00249470831019364,-0.0318015854479095,
-0.0120082878373164));
#38301=CARTESIAN_POINT('Ctrl Pts',(0.00249677081350409,-0.0317991659468958,
-0.0120488276795565));
#38302=CARTESIAN_POINT('Ctrl Pts',(0.00249883331681454,-0.0317967464458821,
-0.0120893675217966));
#38303=CARTESIAN_POINT('Ctrl Pts',(0.00249945501450155,-0.0317950110462313,
-0.0121182150104752));
#38304=CARTESIAN_POINT('Ctrl Pts',(0.00249977959816441,-0.0317934891261923,
-0.0121426574946412));
#38305=CARTESIAN_POINT('Ctrl Pts',(0.00249994188999584,-0.0317927281661728,
-0.0121548787367242));
#38306=CARTESIAN_POINT('Ctrl Pts',(0.00249998123728428,-0.0317920411315702,
-0.0121660007433696));
#38307=CARTESIAN_POINT('Ctrl Pts',(0.00249998704855481,-0.0317919445319498,
-0.0121678061095248));
#38308=CARTESIAN_POINT('Ctrl Pts',(0.00249999285982534,-0.0317918479323293,
-0.0121696114756799));
#38309=CARTESIAN_POINT('Ctrl Pts',(0.00250001929907833,-0.0317916697812854,
-0.0121725320504109));
#38310=CARTESIAN_POINT('Ctrl Pts',(0.00249999006451306,-0.0317910018346423,
-0.0121829015016505));
#38311=CARTESIAN_POINT('Ctrl Pts',(0.00249996082994778,-0.0317903338879991,
-0.0121932709528901));
#38312=CARTESIAN_POINT('Ctrl Pts',(0.00249956436397612,-0.0317875590268506,
-0.0122386669065317));
#38313=CARTESIAN_POINT('Ctrl Pts',(0.00249780162821883,-0.0317850627778348,
-0.01228067230233));
#38314=CARTESIAN_POINT('Ctrl Pts',(0.00249603889246154,-0.0317825665288191,
-0.0123226776981282));
#38315=CARTESIAN_POINT('Ctrl Pts',(0.00249348223220822,-0.0317801299102132,
-0.0123613011644103));
#38316=CARTESIAN_POINT('Ctrl Pts',(0.00248956162025467,-0.0317773729958845,
-0.0124040701548105));
#38317=CARTESIAN_POINT('Ctrl Pts',(0.00248172039634758,-0.0317718591672271,
-0.012489608135611));
#38318=CARTESIAN_POINT('Ctrl Pts',(0.00246784924379192,-0.0317652992968616,
-0.012591678790119));
#38319=CARTESIAN_POINT('Ctrl Pts',(0.00244358882404981,-0.0317578665642037,
-0.0127039381840688));
#38320=CARTESIAN_POINT('Ctrl Pts',(0.00239506798456559,-0.0317430010988878,
-0.0129284569719683));
#38321=CARTESIAN_POINT('Ctrl Pts',(0.00230651280877661,-0.0317242331886206,
-0.0131939916838651));
#38322=CARTESIAN_POINT('Ctrl Pts',(0.00213708827204978,-0.0317033296526518,
-0.0134731018045635));
#38323=CARTESIAN_POINT('Ctrl Pts',(0.00211106753075451,-0.0317001192233237,
-0.0135159683951052));
#38324=CARTESIAN_POINT('Ctrl Pts',(0.00208311322091434,-0.0316968275939304,
-0.0135591125370878));
#38325=CARTESIAN_POINT('Ctrl Pts',(0.00205310009985602,-0.0316934583601711,
-0.0136023104292621));
#38326=CARTESIAN_POINT('Ctrl Pts',(0.00198540349248402,-0.0316858588274699,
-0.0136997461721207));
#38327=CARTESIAN_POINT('Ctrl Pts',(0.00190718091663154,-0.0316778644761325,
-0.0137975154075378));
#38328=CARTESIAN_POINT('Ctrl Pts',(0.00181730979982462,-0.0316695165681902,
-0.0138926482922188));
#38329=CARTESIAN_POINT('Ctrl Pts',(0.00168759454882717,-0.0316574676362027,
-0.0140299581026779));
#38330=CARTESIAN_POINT('Ctrl Pts',(0.001533340118632,-0.0316455973192644,
-0.0141618818978339));
#38331=CARTESIAN_POINT('Ctrl Pts',(0.00135414966748958,-0.031632707315196,
-0.0142773476781847));
#38332=CARTESIAN_POINT('Ctrl Pts',(0.00117495921634717,-0.0316198173111276,
-0.0143928134585354));
#38333=CARTESIAN_POINT('Ctrl Pts',(0.000971210794888545,-0.0316056919371159,
-0.0144920322181475));
#38334=CARTESIAN_POINT('Ctrl Pts',(0.000741339520769619,-0.0315892324856351,
-0.0145634076241482));
#38335=CARTESIAN_POINT('Ctrl Pts',(0.000626403883710157,-0.0315810027598947,
-0.0145990953271485));
#38336=CARTESIAN_POINT('Ctrl Pts',(0.000504724124808493,-0.0315725740963865,
-0.0146274233264182));
#38337=CARTESIAN_POINT('Ctrl Pts',(0.000383936331685177,-0.0315647779266216,
-0.0146461959537223));
#38338=CARTESIAN_POINT('Ctrl Pts',(0.000320100625507402,-0.0315606576923698,
-0.0146561171873982));
#38339=CARTESIAN_POINT('Ctrl Pts',(0.000256473434805746,-0.0315565689173678,
-0.01466375980847));
#38340=CARTESIAN_POINT('Ctrl Pts',(0.000182796389150301,-0.0315518446614979,
-0.0146691614263823));
#38341=CARTESIAN_POINT('Ctrl Pts',(0.000115743617557936,-0.0315475451616066,
-0.0146740773869625));
#38342=CARTESIAN_POINT('Ctrl Pts',(4.24952442558038E-5,-0.0315428561028207,
-0.0146759101548113));
#38343=CARTESIAN_POINT('Ctrl Pts',(-3.22331663466373E-6,-0.0315399279035967,
-0.0146758512086032));
#38344=CARTESIAN_POINT('Ctrl Pts',(-4.56379105660485E-5,-0.0315372113180652,
-0.0146757965222913));
#38345=CARTESIAN_POINT('Ctrl Pts',(-6.54327116774078E-5,-0.0315359428186249,
-0.0146751074190157));
#38346=CARTESIAN_POINT('Ctrl Pts',(-8.89265215644094E-5,-0.0315344368225749,
-0.0146742712007115));
#38347=CARTESIAN_POINT('Ctrl Pts',(-0.000131230291107909,-0.0315317250738147,
-0.014672765477008));
#38348=CARTESIAN_POINT('Ctrl Pts',(-0.000192002285322905,-0.0315278261260052,
-0.0146690484249402));
#38349=CARTESIAN_POINT('Ctrl Pts',(-0.000245472305589629,-0.0315243863391031,
-0.0146637727682111));
#38350=CARTESIAN_POINT('Ctrl Pts',(-0.000294773357939573,-0.031521214746624,
-0.0146589084456003));
#38351=CARTESIAN_POINT('Ctrl Pts',(-0.0003425309527002,-0.0315181352822846,
-0.0146527679862795));
#38352=CARTESIAN_POINT('Ctrl Pts',(-0.00039125743125139,-0.0315149815570885,
-0.0146450470056678));
#38353=CARTESIAN_POINT('Ctrl Pts',(-0.000522802826387516,-0.0315064675409025,
-0.0146242029086674));
#38354=CARTESIAN_POINT('Ctrl Pts',(-0.000661229924873668,-0.0314974254324378,
-0.0145912048720715));
#38355=CARTESIAN_POINT('Ctrl Pts',(-0.00079902678801783,-0.0314888161832273,
-0.0145447256326397));
#38356=CARTESIAN_POINT('Ctrl Pts',(-0.000936823651161993,-0.0314802069340167,
-0.0144982463932078));
#38357=CARTESIAN_POINT('Ctrl Pts',(-0.00107414563365613,-0.0314711370981314,
-0.0144385815328944));
#38358=CARTESIAN_POINT('Ctrl Pts',(-0.00120897499076699,-0.0314614481142302,
-0.0143640898989243));
#38359=CARTESIAN_POINT('Ctrl Pts',(-0.00134380434787785,-0.0314517591303289,
-0.0142895982649543));
#38360=CARTESIAN_POINT('Ctrl Pts',(-0.00147605971849819,-0.0314414785072542,
-0.0142002174268997));
#38361=CARTESIAN_POINT('Ctrl Pts',(-0.00160175792260515,-0.031430573368138,
-0.0140953249736042));
#38362=CARTESIAN_POINT('Ctrl Pts',(-0.00180920400811086,-0.0314125760670816,
-0.0139222156679475));
#38363=CARTESIAN_POINT('Ctrl Pts',(-0.00199855550421331,-0.031394357005186,
-0.013706509475676));
#38364=CARTESIAN_POINT('Ctrl Pts',(-0.00214932033285382,-0.0313754212399793,
-0.0134527331191113));
#38365=CARTESIAN_POINT('Ctrl Pts',(-0.00218126194725279,-0.0313714094361917,
-0.0133989670876167));
#38366=CARTESIAN_POINT('Ctrl Pts',(-0.00221148838932676,-0.031367365462256,
-0.0133434938430907));
#38367=CARTESIAN_POINT('Ctrl Pts',(-0.00223981109177484,-0.0313632846113783,
-0.0132863695057834));
#38368=CARTESIAN_POINT('Ctrl Pts',(-0.00240181625098881,-0.0313399422450423,
-0.0129596197057801));
#38369=CARTESIAN_POINT('Ctrl Pts',(-0.00250001841270888,-0.0313177033710342,
-0.0125780611358331));
#38370=CARTESIAN_POINT('Ctrl Pts',(-0.00249999999738109,-0.031291873856013,
-0.0121757388551144));
#38371=CARTESIAN_POINT('',(-0.00249999942061914,-0.0302901454774401,-0.0121744765208516));
#38372=CARTESIAN_POINT('Ctrl Pts',(-0.00249999994976247,-0.0312900992552675,
-0.0121753521003062));
#38373=CARTESIAN_POINT('Ctrl Pts',(-0.00249990259183997,-0.0312591857748376,
-0.0116897146742599));
#38374=CARTESIAN_POINT('Ctrl Pts',(-0.00235401452783209,-0.0312282722944076,
-0.0112041304353443));
#38375=CARTESIAN_POINT('Ctrl Pts',(-0.00208666920114698,-0.0311973588139777,
-0.0107989685255906));
#38376=CARTESIAN_POINT('Ctrl Pts',(-0.00199372216379006,-0.0311866112297353,
-0.010658107267126));
#38377=CARTESIAN_POINT('Ctrl Pts',(-0.00188654303827572,-0.031175863645493,
-0.0105268207704096));
#38378=CARTESIAN_POINT('Ctrl Pts',(-0.00176745734384853,-0.0311651160612506,
-0.0104077767786898));
#38379=CARTESIAN_POINT('Ctrl Pts',(-0.00143124037051339,-0.0311347721961708,
-0.0100716775454251));
#38380=CARTESIAN_POINT('Ctrl Pts',(-0.000994786137417781,-0.031104428331091,
-0.00983322878898758));
#38381=CARTESIAN_POINT('Ctrl Pts',(-0.000528612127681506,-0.0310740844660112,
-0.00973237846195523));
#38382=CARTESIAN_POINT('Ctrl Pts',(-0.000354745538862485,-0.0310627672664187,
-0.00969476481988986));
#38383=CARTESIAN_POINT('Ctrl Pts',(-0.000177009517374391,-0.0310514500668262,
-0.00967582674646241));
#38384=CARTESIAN_POINT('Ctrl Pts',(3.7444390193485E-7,-0.0310401328672337,
-0.00967585331459975));
#38385=CARTESIAN_POINT('Ctrl Pts',(0.000477738492770387,-0.0310096767640976,
-0.00967592481302339));
#38386=CARTESIAN_POINT('Ctrl Pts',(0.000956612727593189,-0.0309792206609616,
-0.00981704046168377));
#38387=CARTESIAN_POINT('Ctrl Pts',(0.00135843499603846,-0.0309487645578255,
-0.0100771264435559));
#38388=CARTESIAN_POINT('Ctrl Pts',(0.00150626753529031,-0.0309375595962893,
-0.0101728134528218));
#38389=CARTESIAN_POINT('Ctrl Pts',(0.00164381276844332,-0.0309263546347531,
-0.0102841012708437));
#38390=CARTESIAN_POINT('Ctrl Pts',(0.00176798690091599,-0.0309151496732169,
-0.010408306308911));
#38391=CARTESIAN_POINT('Ctrl Pts',(0.00210544008061321,-0.0308846992901661,
-0.010745843477044));
#38392=CARTESIAN_POINT('Ctrl Pts',(0.00234425609545278,-0.0308542489071155,
-0.0111841501902191));
#38393=CARTESIAN_POINT('Ctrl Pts',(0.00244451688867356,-0.0308237985240648,
-0.0116520812168658));
#38394=CARTESIAN_POINT('Ctrl Pts',(0.00248142912817006,-0.0308125878424432,
-0.0118243557577763));
#38395=CARTESIAN_POINT('Ctrl Pts',(0.00250001739721303,-0.0308013771608217,
-0.0120003907020759));
#38396=CARTESIAN_POINT('Ctrl Pts',(0.00249999998772879,-0.0307901664792,
-0.0121761009881092));
#38397=CARTESIAN_POINT('Ctrl Pts',(0.00249995270019697,-0.0307597160961492,
-0.012653364164095));
#38398=CARTESIAN_POINT('Ctrl Pts',(0.00235891876369913,-0.0307292657130982,
-0.0131321617656519));
#38399=CARTESIAN_POINT('Ctrl Pts',(0.00209894355269856,-0.0306988153300473,
-0.0135339534163663));
#38400=CARTESIAN_POINT('Ctrl Pts',(0.00200323049335481,-0.0306876046484259,
-0.0136818779356336));
#38401=CARTESIAN_POINT('Ctrl Pts',(0.00189189875249167,-0.0306763939668046,
-0.0138195067532682));
#38402=CARTESIAN_POINT('Ctrl Pts',(0.0017676366069028,-0.0306651832851831,
-0.0139437505759777));
#38403=CARTESIAN_POINT('Ctrl Pts',(0.00143005314411421,-0.0306347271820469,
-0.0142812842609272));
#38404=CARTESIAN_POINT('Ctrl Pts',(0.0009916643058973,-0.0306042710789107,
-0.0145201443823691));
#38405=CARTESIAN_POINT('Ctrl Pts',(0.000523638769525182,-0.0305738149757745,
-0.014620398732863));
#38406=CARTESIAN_POINT('Ctrl Pts',(0.0003514496976169,-0.0305626100142384,
-0.014657282839017));
#38407=CARTESIAN_POINT('Ctrl Pts',(0.000175503802646239,-0.0305514050527023,
-0.0146758617810041));
#38408=CARTESIAN_POINT('Ctrl Pts',(-1.20959199542376E-7,-0.0305402000911662,
-0.0146758532836319));
#38409=CARTESIAN_POINT('Ctrl Pts',(-0.000475725811651964,-0.0305098562260865,
-0.0146758302721189));
#38410=CARTESIAN_POINT('Ctrl Pts',(-0.000953003524480613,-0.0304795123610067,
-0.0145357650987292));
#38411=CARTESIAN_POINT('Ctrl Pts',(-0.00135388681630664,-0.030449168495927,
-0.0142775170295558));
#38412=CARTESIAN_POINT('Ctrl Pts',(-0.00150340225262242,-0.0304378512963344,
-0.014181199538836));
#38413=CARTESIAN_POINT('Ctrl Pts',(-0.00164243535305725,-0.0304265340967419,
-0.0140689576145839));
#38414=CARTESIAN_POINT('Ctrl Pts',(-0.0017678076733794,-0.0304152168971493,
-0.0139435795181734));
#38415=CARTESIAN_POINT('Ctrl Pts',(-0.00211026825641089,-0.0303843034167193,
-0.013601103157476));
#38416=CARTESIAN_POINT('Ctrl Pts',(-0.00235095201767094,-0.0303533899362893,
-0.0131552776793517));
#38417=CARTESIAN_POINT('Ctrl Pts',(-0.00244880888004733,-0.0303224764558593,
-0.0126791773064512));
#38418=CARTESIAN_POINT('Ctrl Pts',(-0.00248283044143243,-0.030311728871617,
-0.0125136531145984));
#38419=CARTESIAN_POINT('Ctrl Pts',(-0.00249999960942255,-0.0303009812873747,
-0.0123446989796761));
#38420=CARTESIAN_POINT('Ctrl Pts',(-0.00249999999999331,-0.0302902337031324,
-0.0121758590697104));
#38421=CARTESIAN_POINT('',(-0.00249999943912681,-0.0292900991654731,-0.0121775325936968));
#38422=CARTESIAN_POINT('Ctrl Pts',(-0.0024999991170802,-0.0302900992552675,
-0.0121737521920283));
#38423=CARTESIAN_POINT('Ctrl Pts',(-0.00249959096584859,-0.0302591749334474,
-0.0116881111586653));
#38424=CARTESIAN_POINT('Ctrl Pts',(-0.00235339003378415,-0.0302282506116274,
-0.0112026172509638));
#38425=CARTESIAN_POINT('Ctrl Pts',(-0.00199282144836561,-0.0301865839449607,
-0.0106569403810191));
#38426=CARTESIAN_POINT('Ctrl Pts',(-0.00188565876843709,-0.0301758416001141,
-0.0105258239057141));
#38427=CARTESIAN_POINT('Ctrl Pts',(-0.00143023212870617,-0.0301347445227216,
-0.0100709902258644));
#38428=CARTESIAN_POINT('Ctrl Pts',(-0.00099365647799636,-0.0301043897901757,
-0.00983274807457304));
#38429=CARTESIAN_POINT('Ctrl Pts',(-0.000353683170743005,-0.030062723123509,
-0.00969462347352273));
#38430=CARTESIAN_POINT('Ctrl Pts',(-0.000176084995757376,-0.0300514111893883,
-0.00967577159798382));
#38431=CARTESIAN_POINT('Ctrl Pts',(0.000478527791617883,-0.0300096322717532,
-0.00967607428947804));
#38432=CARTESIAN_POINT('Ctrl Pts',(0.00095736400795089,-0.029979165288239,
-0.00981734402679618));
#38433=CARTESIAN_POINT('Ctrl Pts',(0.00150678939658889,-0.0299374986215723,
-0.0101732186109999));
#38434=CARTESIAN_POINT('Ctrl Pts',(0.00164419531455132,-0.0299262989384199,
-0.0102844469810999));
#38435=CARTESIAN_POINT('Ctrl Pts',(0.00210565841324517,-0.0298846380046097,
-0.0107461624561916));
#38436=CARTESIAN_POINT('Ctrl Pts',(0.00234441033443847,-0.029854176753952,
-0.0111845119625509));
#38437=CARTESIAN_POINT('Ctrl Pts',(0.00248145420869358,-0.0298125100872853,
-0.0118246047362775));
#38438=CARTESIAN_POINT('Ctrl Pts',(0.00250001480158532,-0.0298013046712764,
-0.0120004962840195));
#38439=CARTESIAN_POINT('Ctrl Pts',(0.00249995972970253,-0.0297596380046098,
-0.0126533349660584));
#38440=CARTESIAN_POINT('Ctrl Pts',(0.00235892856150225,-0.029729176753952,
-0.0131321406088429));
#38441=CARTESIAN_POINT('Ctrl Pts',(0.00200331865873349,-0.0296875100872853,
-0.0136817438883177));
#38442=CARTESIAN_POINT('Ctrl Pts',(0.00189209125366563,-0.0296763046712764,
-0.0138192699312786));
#38443=CARTESIAN_POINT('Ctrl Pts',(0.00143042324015757,-0.0296346322717532,
-0.0142810345935773));
#38444=CARTESIAN_POINT('Ctrl Pts',(0.000992069613805846,-0.029604165288239,
-0.0145199741564081));
#38445=CARTESIAN_POINT('Ctrl Pts',(0.000352012654775048,-0.0295624986215723,
-0.014657192859098));
#38446=CARTESIAN_POINT('Ctrl Pts',(0.000176216403953808,-0.0295512989384199,
-0.0146758016426758));
#38447=CARTESIAN_POINT('Ctrl Pts',(-0.000474878817339744,-0.0295097445227216,
-0.0146759928580223));
#38448=CARTESIAN_POINT('Ctrl Pts',(-0.000952210864759681,-0.0294793897901757,
-0.0145360863615342));
#38449=CARTESIAN_POINT('Ctrl Pts',(-0.00150261225706842,-0.029437723123509,
-0.014181778794066));
#38450=CARTESIAN_POINT('Ctrl Pts',(-0.00164157878599002,-0.0294264111893883,
-0.0140696870542259));
#38451=CARTESIAN_POINT('Ctrl Pts',(-0.00210955062163189,-0.0293841749334474,
-0.0136021667831768));
#38452=CARTESIAN_POINT('Ctrl Pts',(-0.00235046036159436,-0.0293532506116274,
-0.0131564586379207));
#38453=CARTESIAN_POINT('Ctrl Pts',(-0.00248263255009951,-0.0293115839449607,
-0.012515034510425));
#38454=CARTESIAN_POINT('Ctrl Pts',(-0.00249988611653098,-0.0293008416001141,
-0.0123462323031989));
#38455=CARTESIAN_POINT('Ctrl Pts',(-0.00249999943598566,-0.0292900992552675,
-0.0121775325933754));
#38456=CARTESIAN_POINT('',(-0.00249382779728175,-0.0292787744408383,-0.0120002887186913));
#38457=CARTESIAN_POINT('Origin',(1.04421208127001E-5,-0.0292843824914073,
-0.012176220437913));
#38458=CARTESIAN_POINT('',(0.000565648716052718,-0.0292787743898723,-0.0146110209460896));
#38459=CARTESIAN_POINT('Origin',(0.,-0.0292787743898623,-0.0121758532865581));
#38460=CARTESIAN_POINT('',(-0.00249999998652498,-0.0299924495244571,-0.0121755937194362));
#38461=CARTESIAN_POINT('Ctrl Pts',(0.000565648716059988,-0.0292787743898623,
-0.0146110209460879));
#38462=CARTESIAN_POINT('Ctrl Pts',(0.0010206242086387,-0.0293085108538038,
-0.0145053377492005));
#38463=CARTESIAN_POINT('Ctrl Pts',(0.0014447229436206,-0.0293382473177453,
-0.0142688517650026));
#38464=CARTESIAN_POINT('Ctrl Pts',(0.00177366822203208,-0.0293679837816867,
-0.0139376992043822));
#38465=CARTESIAN_POINT('Ctrl Pts',(0.00210261350044357,-0.0293977202456281,
-0.0136065466437619));
#38466=CARTESIAN_POINT('Ctrl Pts',(0.00233631458587225,-0.0294274567095696,
-0.0131806244778636));
#38467=CARTESIAN_POINT('Ctrl Pts',(0.00243889607330461,-0.029457193173511,
-0.0127252037608633));
#38468=CARTESIAN_POINT('Ctrl Pts',(0.00254147756073697,-0.0294869296374525,
-0.012269783043863));
#38469=CARTESIAN_POINT('Ctrl Pts',(0.00251297505440625,-0.0295166661013939,
-0.0117848538514163));
#38470=CARTESIAN_POINT('Ctrl Pts',(0.00235775410251832,-0.0295464025653354,
-0.0113445918402862));
#38471=CARTESIAN_POINT('Ctrl Pts',(0.00220253315063038,-0.0295761390292768,
-0.0109043298291561));
#38472=CARTESIAN_POINT('Ctrl Pts',(0.00192059182778953,-0.0296058754932183,
-0.0105087453803813));
#38473=CARTESIAN_POINT('Ctrl Pts',(0.00155507400256916,-0.0296356119571598,
-0.0102183689707758));
#38474=CARTESIAN_POINT('Ctrl Pts',(0.00118955617734879,-0.0296653484211012,
-0.0099279925611704));
#38475=CARTESIAN_POINT('Ctrl Pts',(0.000740457719301776,-0.0296950848850426,
-0.0097428209094049));
#38476=CARTESIAN_POINT('Ctrl Pts',(0.000276498140069873,-0.029724821348984,
-0.00969119057734828));
#38477=CARTESIAN_POINT('Ctrl Pts',(-0.000187461439162031,-0.0297545578129255,
-0.00963956024529165));
#38478=CARTESIAN_POINT('Ctrl Pts',(-0.000666272462951498,-0.029784294276867,
-0.00972146700967555));
#38479=CARTESIAN_POINT('Ctrl Pts',(-0.00108669381979509,-0.0298140307408084,
-0.00992438786554468));
#38480=CARTESIAN_POINT('Ctrl Pts',(-0.00150711517663868,-0.0298437672047499,
-0.0101273087214138));
#38481=CARTESIAN_POINT('Ctrl Pts',(-0.00186914848155188,-0.0298735036686913,
-0.0104512805949887));
#38482=CARTESIAN_POINT('Ctrl Pts',(-0.00211732733988455,-0.0299032401326328,
-0.0108465959992817));
#38483=CARTESIAN_POINT('Ctrl Pts',(-0.00236550619821721,-0.0299329765965742,
-0.0112419114035747));
#38484=CARTESIAN_POINT('Ctrl Pts',(-0.00249995149020126,-0.0299627130605157,
-0.0117085052539399));
#38485=CARTESIAN_POINT('Ctrl Pts',(-0.00249999998652498,-0.0299924495244571,
-0.0121755937194362));
#38486=CARTESIAN_POINT('',(-0.00249999945595836,-0.0309923794005721,-0.012177043828097));
#38487=CARTESIAN_POINT('Ctrl Pts',(-0.00249999999999978,-0.029992465890772,
-0.012175852244816));
#38488=CARTESIAN_POINT('Ctrl Pts',(-0.00250000020236312,-0.0300233774710986,
-0.0126614890819379));
#38489=CARTESIAN_POINT('Ctrl Pts',(-0.00235421003106896,-0.0300542890514251,
-0.0131471021162331));
#38490=CARTESIAN_POINT('Ctrl Pts',(-0.00208694667699899,-0.0300852006317517,
-0.0135523174406002));
#38491=CARTESIAN_POINT('Ctrl Pts',(-0.00199401628883952,-0.0300959489259515,
-0.0136932152360075));
#38492=CARTESIAN_POINT('Ctrl Pts',(-0.00188684827597316,-0.0301066972201514,
-0.0138245387021237));
#38493=CARTESIAN_POINT('Ctrl Pts',(-0.00176776854431825,-0.0301174455143512,
-0.0139436186481712));
#38494=CARTESIAN_POINT('Ctrl Pts',(-0.00143161166736268,-0.0301477874790213,
-0.0142797761303475));
#38495=CARTESIAN_POINT('Ctrl Pts',(-0.000995200662721201,-0.0301781294436916,
-0.0145183015038843));
#38496=CARTESIAN_POINT('Ctrl Pts',(-0.000529045559956314,-0.0302084714083617,
-0.0146192343038148));
#38497=CARTESIAN_POINT('Ctrl Pts',(-0.000355163394862593,-0.0302197893720153,
-0.0146568836048238));
#38498=CARTESIAN_POINT('Ctrl Pts',(-0.000177407490434834,-0.030231107335669,
-0.0146758532210078));
#38499=CARTESIAN_POINT('Ctrl Pts',(-9.23727244943536E-10,-0.0302424252993226,
-0.0146758532865579));
#38500=CARTESIAN_POINT('Ctrl Pts',(0.000477361897951327,-0.0302728794993312,
-0.0146758534629391));
#38501=CARTESIAN_POINT('Ctrl Pts',(0.000956256347303985,-0.0303033336993398,
-0.0145348104111621));
#38502=CARTESIAN_POINT('Ctrl Pts',(0.00135811717461238,-0.0303337878993484,
-0.0142747858104909));
#38503=CARTESIAN_POINT('Ctrl Pts',(0.0015059832571254,-0.0303449936276636,
-0.0141791088585576));
#38504=CARTESIAN_POINT('Ctrl Pts',(0.00164356173072387,-0.0303561993559788,
-0.0140678255018165));
#38505=CARTESIAN_POINT('Ctrl Pts',(0.00176776723797135,-0.030367405084294,
-0.0139436199545194));
#38506=CARTESIAN_POINT('Ctrl Pts',(0.00210526151255424,-0.0303978535662714,
-0.0136061255711127));
#38507=CARTESIAN_POINT('Ctrl Pts',(0.00234413180385817,-0.0304283020482487,
-0.0131678496812006));
#38508=CARTESIAN_POINT('Ctrl Pts',(0.00244445112861001,-0.0304587505302261,
-0.0126999321735945));
#38509=CARTESIAN_POINT('Ctrl Pts',(0.00248138974275191,-0.0304699619765725,
-0.0125276401021869));
#38510=CARTESIAN_POINT('Ctrl Pts',(0.00250000012159547,-0.0304811734229191,
-0.0123515843578053));
#38511=CARTESIAN_POINT('Ctrl Pts',(0.0024999999999994,-0.0304923848692655,
-0.012175851556715));
#38512=CARTESIAN_POINT('Ctrl Pts',(0.00249999966976407,-0.0305228333512428,
-0.0116985895816349));
#38513=CARTESIAN_POINT('Ctrl Pts',(0.00235901351912043,-0.03055328183322,
-0.0112197790495299));
#38514=CARTESIAN_POINT('Ctrl Pts',(0.00209907885972606,-0.0305837303151973,
-0.0108179622965846));
#38515=CARTESIAN_POINT('Ctrl Pts',(0.00200336822661217,-0.0305949417615438,
-0.01067000920749));
#38516=CARTESIAN_POINT('Ctrl Pts',(0.00189203385010139,-0.0306061532078904,
-0.0105323529268543));
#38517=CARTESIAN_POINT('Ctrl Pts',(0.00176776479160246,-0.0306173646542369,
-0.0104080841722305));
#38518=CARTESIAN_POINT('Ctrl Pts',(0.00143020667060413,-0.0306478188542455,
-0.0100705268766629));
#38519=CARTESIAN_POINT('Ctrl Pts',(0.000991836324402045,-0.0306782730542541,
-0.00983163516427871));
#38520=CARTESIAN_POINT('Ctrl Pts',(0.000523819145203904,-0.0307087272542627,
-0.00973134648494804));
#38521=CARTESIAN_POINT('Ctrl Pts',(0.000351610604002277,-0.0307199329825779,
-0.00969444491822315));
#38522=CARTESIAN_POINT('Ctrl Pts',(0.000175642919289985,-0.0307311387108931,
-0.00967585297858804));
#38523=CARTESIAN_POINT('Ctrl Pts',(-4.38341345831789E-9,-0.0307423444392083,
-0.00967585328656194));
#38524=CARTESIAN_POINT('Ctrl Pts',(-0.000475607941086921,-0.0307726864038785,
-0.00967585412046876));
#38525=CARTESIAN_POINT('Ctrl Pts',(-0.000952891164814528,-0.0308030283685486,
-0.00981589631166478));
#38526=CARTESIAN_POINT('Ctrl Pts',(-0.00135378597959753,-0.0308333703332188,
-0.0100741245882135));
#38527=CARTESIAN_POINT('Ctrl Pts',(-0.00150332517364712,-0.0308446882968725,
-0.0101704472317898));
#38528=CARTESIAN_POINT('Ctrl Pts',(-0.0016423800975229,-0.0308560062605261,
-0.0102826989053507));
#38529=CARTESIAN_POINT('Ctrl Pts',(-0.00176777099068193,-0.0308673242241798,
-0.0104080903713165));
#38530=CARTESIAN_POINT('Ctrl Pts',(-0.0021102381370025,-0.0308982358048934,
-0.010750559082085));
#38531=CARTESIAN_POINT('Ctrl Pts',(-0.002350931064765,-0.0309291473856069,
-0.0111963788623779));
#38532=CARTESIAN_POINT('Ctrl Pts',(-0.00244879805764301,-0.0309600589663204,
-0.0116724766155812));
#38533=CARTESIAN_POINT('Ctrl Pts',(-0.00248282764897228,-0.0309708073139307,
-0.0118380218264623));
#38534=CARTESIAN_POINT('Ctrl Pts',(-0.00250000047530196,-0.030981555661541,
-0.0120069982515906));
#38535=CARTESIAN_POINT('Ctrl Pts',(-0.0024999999999901,-0.0309923040091512,
-0.0121758603235419));
#38536=CARTESIAN_POINT('',(-0.00249989090829521,-0.0319922844637892,-0.0121752665328745));
#38537=CARTESIAN_POINT('Ctrl Pts',(-0.00249999894993767,-0.0309924495244571,
-0.0121781446421717));
#38538=CARTESIAN_POINT('Ctrl Pts',(-0.00249955383980213,-0.0310233727917168,
-0.0126637850485941));
#38539=CARTESIAN_POINT('Ctrl Pts',(-0.00235331629776196,-0.0310542960589767,
-0.0131492673344889));
#38540=CARTESIAN_POINT('Ctrl Pts',(-0.00208567790527778,-0.0310852193262364,
-0.0135542391815222));
#38541=CARTESIAN_POINT('Ctrl Pts',(-0.0019926946469783,-0.0310959627256433,
-0.0136949349968991));
#38542=CARTESIAN_POINT('Ctrl Pts',(-0.00188550614587116,-0.0311067061250502,
-0.0138260593105748));
#38543=CARTESIAN_POINT('Ctrl Pts',(-0.00176643472427443,-0.0311174495244571,
-0.0139449514649749));
#38544=CARTESIAN_POINT('Ctrl Pts',(-0.00143001851901507,-0.0311478031862475,
-0.0142808611810261));
#38545=CARTESIAN_POINT('Ctrl Pts',(-0.000993419834120211,-0.031178156848038,
-0.0145190586297705));
#38546=CARTESIAN_POINT('Ctrl Pts',(-0.000527181479049827,-0.0312085105098284,
-0.0146196371739235));
#38547=CARTESIAN_POINT('Ctrl Pts',(-0.000353411446926351,-0.0312198235147046,
-0.0146571234438932));
#38548=CARTESIAN_POINT('Ctrl Pts',(-0.000175788189397624,-0.0312311365195809,
-0.0146759574606499));
#38549=CARTESIAN_POINT('Ctrl Pts',(1.47533730703213E-6,-0.0312424495244571,
-0.014675852851234));
#38550=CARTESIAN_POINT('Ctrl Pts',(0.000478845873260156,-0.0312729154375606,
-0.0146755711381606));
#38551=CARTESIAN_POINT('Ctrl Pts',(0.000957663075037329,-0.0313033813506641,
-0.0145342409292666));
#38552=CARTESIAN_POINT('Ctrl Pts',(0.00135937336850242,-0.0313338472637676,
-0.0142739724550055));
#38553=CARTESIAN_POINT('Ctrl Pts',(0.00150706163852454,-0.0313450480173308,
-0.0141782850869439));
#38554=CARTESIAN_POINT('Ctrl Pts',(0.0016444698318857,-0.0313562487708939,
-0.0140670230067143));
#38555=CARTESIAN_POINT('Ctrl Pts',(0.00176852150679043,-0.0313674495244571,
-0.013942865363489));
#38556=CARTESIAN_POINT('Ctrl Pts',(0.00210587707764771,-0.0313979097065968,
-0.0136052216143116));
#38557=CARTESIAN_POINT('Ctrl Pts',(0.00234456149770483,-0.0314283698887366,
-0.0131668365917466));
#38558=CARTESIAN_POINT('Ctrl Pts',(0.00244467869100603,-0.0314588300708764,
-0.0126988696321354));
#38559=CARTESIAN_POINT('Ctrl Pts',(0.00248151240961152,-0.0314700365554033,
-0.0125267017682688));
#38560=CARTESIAN_POINT('Ctrl Pts',(0.00250004622107205,-0.0314812430399301,
-0.0123507843182147));
#38561=CARTESIAN_POINT('Ctrl Pts',(0.00249999991305973,-0.0314924495244571,
-0.0121751939677149));
#38562=CARTESIAN_POINT('Ctrl Pts',(0.00249987404392688,-0.0315229097065968,
-0.0116979243971061));
#38563=CARTESIAN_POINT('Ctrl Pts',(0.00235875767002164,-0.0315533698887364,
-0.0112191449994495));
#38564=CARTESIAN_POINT('Ctrl Pts',(0.00209871088251693,-0.0315838300708761,
-0.0108173936325363));
#38565=CARTESIAN_POINT('Ctrl Pts',(0.00200303810265292,-0.0315950365554031,
-0.0106695868841601));
#38566=CARTESIAN_POINT('Ctrl Pts',(0.00189176989217815,-0.0316062430399301,
-0.0105320643269465));
#38567=CARTESIAN_POINT('Ctrl Pts',(0.00176758924132678,-0.0316174495244571,
-0.0104079086398155));
#38568=CARTESIAN_POINT('Ctrl Pts',(0.00142999211986863,-0.0316479154375606,
-0.010070379384648));
#38569=CARTESIAN_POINT('Ctrl Pts',(0.000991590643801229,-0.0316783813506642,
-0.00983152996620587));
#38570=CARTESIAN_POINT('Ctrl Pts',(0.000523556634283034,-0.0317088472637678,
-0.00973129024775173));
#38571=CARTESIAN_POINT('Ctrl Pts',(0.00035148453580507,-0.0317200480173309,
-0.00969443724486205));
#38572=CARTESIAN_POINT('Ctrl Pts',(0.000175661390257492,-0.031731248770894,
-0.00967586429208138));
#38573=CARTESIAN_POINT('Ctrl Pts',(1.56699690761575E-7,-0.0317424495244571,
-0.00967585329146906));
#38574=CARTESIAN_POINT('Ctrl Pts',(-0.00047545505179257,-0.0317728031862475,
-0.00967582348018325));
#38575=CARTESIAN_POINT('Ctrl Pts',(-0.0009527537503948,-0.0318031568480379,
-0.00981583951346853));
#38576=CARTESIAN_POINT('Ctrl Pts',(-0.00135366848554465,-0.0318335105098283,
-0.0100740489114453));
#38577=CARTESIAN_POINT('Ctrl Pts',(-0.00150309198459525,-0.0318448235147045,
-0.0101702852139574));
#38578=CARTESIAN_POINT('Ctrl Pts',(-0.00164204916855227,-0.0318561365195809,
-0.0102824252413429));
#38579=CARTESIAN_POINT('Ctrl Pts',(-0.0017673675983348,-0.0318674495244571,
-0.0104076870691576));
#38580=CARTESIAN_POINT('Ctrl Pts',(-0.0021099163145363,-0.031898372791717,
-0.0107500810680407));
#38581=CARTESIAN_POINT('Ctrl Pts',(-0.00235071149540477,-0.0319292960589769,
-0.0111958503674165));
#38582=CARTESIAN_POINT('Ctrl Pts',(-0.00244868552940724,-0.0319602193262366,
-0.0116719295045517));
#38583=CARTESIAN_POINT('Ctrl Pts',(-0.00248272378836424,-0.0319709627256435,
-0.0118373295017941));
#38584=CARTESIAN_POINT('Ctrl Pts',(-0.00249993416323528,-0.0319817061250503,
-0.0120061587251184));
#38585=CARTESIAN_POINT('Ctrl Pts',(-0.00249999981076385,-0.0319924495244571,
-0.01217488056835));
#38586=CARTESIAN_POINT('',(-0.00249999968239255,-0.0329925058241451,-0.0121749586412689));
#38587=CARTESIAN_POINT('Ctrl Pts',(-0.00249999999995083,-0.0319925127996754,
-0.0121758689662745));
#38588=CARTESIAN_POINT('Ctrl Pts',(-0.0024999969540786,-0.0320234311161074,
-0.0126615078884318));
#38589=CARTESIAN_POINT('Ctrl Pts',(-0.0023542023509467,-0.0320543494325394,
-0.0131471216855443));
#38590=CARTESIAN_POINT('Ctrl Pts',(-0.0020869343037223,-0.0320852677489715,
-0.0135523362003449));
#38591=CARTESIAN_POINT('Ctrl Pts',(-0.00199404483670037,-0.0320960134627387,
-0.0136931691981547));
#38592=CARTESIAN_POINT('Ctrl Pts',(-0.0018869307868893,-0.0321067591765059,
-0.0138244364875498));
#38593=CARTESIAN_POINT('Ctrl Pts',(-0.00176791476587925,-0.0321175048902731,
-0.0139434724142511));
#38594=CARTESIAN_POINT('Ctrl Pts',(-0.00143178245151699,-0.0321478535912915,
-0.0142796609474821));
#38595=CARTESIAN_POINT('Ctrl Pts',(-0.000995386817022444,-0.03217820229231,
-0.0145182231418634));
#38596=CARTESIAN_POINT('Ctrl Pts',(-0.000529236055691413,-0.0322085509933284,
-0.0146191930495375));
#38597=CARTESIAN_POINT('Ctrl Pts',(-0.00035543457044395,-0.0322198663225092,
-0.0146568390674673));
#38598=CARTESIAN_POINT('Ctrl Pts',(-0.000177761363019128,-0.03223118165169,
-0.0146758224807982));
#38599=CARTESIAN_POINT('Ctrl Pts',(-4.33775247199217E-7,-0.0322424969808708,
-0.0146758532489259));
#38600=CARTESIAN_POINT('Ctrl Pts',(0.000476933345555184,-0.0322729579270768,
-0.0146759360769435));
#38601=CARTESIAN_POINT('Ctrl Pts',(0.000955855591101025,-0.0323034188732828,
-0.0145349735201245));
#38602=CARTESIAN_POINT('Ctrl Pts',(0.00135776313800081,-0.0323338798194889,
-0.0142750148480121));
#38603=CARTESIAN_POINT('Ctrl Pts',(0.0015055787696942,-0.0323450829034821,
-0.0141794059060332));
#38604=CARTESIAN_POINT('Ctrl Pts',(0.00164311873360453,-0.0323562859874753,
-0.0140682029338377));
#38605=CARTESIAN_POINT('Ctrl Pts',(0.00176730125990038,-0.0323674890714685,
-0.0139440858099426));
#38606=CARTESIAN_POINT('Ctrl Pts',(0.00210488743550194,-0.0323979442924487,
-0.0136066774286491));
#38607=CARTESIAN_POINT('Ctrl Pts',(0.00234387389339254,-0.0324283995134288,
-0.0131684605187964));
#38608=CARTESIAN_POINT('Ctrl Pts',(0.00244431520109232,-0.0324588547344089,
-0.0127005657770793));
#38609=CARTESIAN_POINT('Ctrl Pts',(0.00248128184981438,-0.0324700635436281,
-0.0125283607256711));
#38610=CARTESIAN_POINT('Ctrl Pts',(0.00249993778676581,-0.0324812723528472,
-0.0123523906424397));
#38611=CARTESIAN_POINT('Ctrl Pts',(0.00249999984398088,-0.0324924811620663,
-0.0121767365167549));
#38612=CARTESIAN_POINT('Ctrl Pts',(0.00250016845834137,-0.0325229363830465,
-0.0116994703674921));
#38613=CARTESIAN_POINT('Ctrl Pts',(0.0023593494439565,-0.0325533916040268,
-0.0112206066619966));
#38614=CARTESIAN_POINT('Ctrl Pts',(0.0020995534792578,-0.0325838468250071,
-0.0108186962625788));
#38615=CARTESIAN_POINT('Ctrl Pts',(0.00200393757792991,-0.032595055634226,
-0.0106707762395023));
#38616=CARTESIAN_POINT('Ctrl Pts',(0.00189270843726949,-0.032606264443445,
-0.0105331382635439));
#38617=CARTESIAN_POINT('Ctrl Pts',(0.00176855022373763,-0.032617473252664,
-0.0104088699515723));
#38618=CARTESIAN_POINT('Ctrl Pts',(0.00143113912238476,-0.03264793419887,
-0.0100711596478167));
#38619=CARTESIAN_POINT('Ctrl Pts',(0.000992870892482344,-0.032678395145076,
-0.00983207245885684));
#38620=CARTESIAN_POINT('Ctrl Pts',(0.000524894531450418,-0.0327088560912821,
-0.00973157717063882));
#38621=CARTESIAN_POINT('Ctrl Pts',(0.000352779770338811,-0.0327200591752753,
-0.00969461649491933));
#38622=CARTESIAN_POINT('Ctrl Pts',(0.000176901206017232,-0.0327312622592685,
-0.00967594723280333));
#38623=CARTESIAN_POINT('Ctrl Pts',(1.33268511776818E-6,-0.0327424653432617,
-0.00967585364176805));
#38624=CARTESIAN_POINT('Ctrl Pts',(-0.000474275330698369,-0.0327728140442801,
-0.0096756001074422));
#38625=CARTESIAN_POINT('Ctrl Pts',(-0.000951636949235143,-0.0328031627452987,
-0.00981538955061219));
#38626=CARTESIAN_POINT('Ctrl Pts',(-0.00135267162894355,-0.0328335114463172,
-0.0100734072196515));
#38627=CARTESIAN_POINT('Ctrl Pts',(-0.00150219497793399,-0.0328448267754979,
-0.0101696075432781));
#38628=CARTESIAN_POINT('Ctrl Pts',(-0.00164125192130111,-0.0328561421046787,
-0.010281728147083));
#38629=CARTESIAN_POINT('Ctrl Pts',(-0.0017666653529596,-0.0328674574338594,
-0.0104069854196296));
#38630=CARTESIAN_POINT('Ctrl Pts',(-0.0021093484603536,-0.0328983757502914,
-0.0107492418335746));
#38631=CARTESIAN_POINT('Ctrl Pts',(-0.00235032038741192,-0.0329292940667234,
-0.0111949134906389));
#38632=CARTESIAN_POINT('Ctrl Pts',(-0.00244848416552665,-0.0329602123831554,
-0.011670952017828));
#38633=CARTESIAN_POINT('Ctrl Pts',(-0.00248260115453699,-0.0329709580969226,
-0.011836400022301));
#38634=CARTESIAN_POINT('Ctrl Pts',(-0.00249987904565359,-0.0329817038106899,
-0.012005286551277));
#38635=CARTESIAN_POINT('Ctrl Pts',(-0.00249999936479533,-0.0329924495244571,
-0.0121740711465624));
#38636=CARTESIAN_POINT('',(-0.00249999969181303,-0.0339923940613826,-0.0121767345639794));
#38637=CARTESIAN_POINT('Ctrl Pts',(-0.00249999999998977,-0.0329925621238332,
-0.0121758461359755));
#38638=CARTESIAN_POINT('Ctrl Pts',(-0.00250000139097379,-0.0330234456018171,
-0.0126621645583693));
#38639=CARTESIAN_POINT('Ctrl Pts',(-0.00235381656149027,-0.0330543454390897,
-0.0131484007170305));
#38640=CARTESIAN_POINT('Ctrl Pts',(-0.00208584926554848,-0.0330852540039819,
-0.0135539798560033));
#38641=CARTESIAN_POINT('Ctrl Pts',(-0.00199318331240229,-0.0330959425158619,
-0.0136942334543279));
#38642=CARTESIAN_POINT('Ctrl Pts',(-0.0018863982675443,-0.0331066320714345,
-0.0138249865451629));
#38643=CARTESIAN_POINT('Ctrl Pts',(-0.0017677846850215,-0.0331173223551014,
-0.0139436025072915));
#38644=CARTESIAN_POINT('Ctrl Pts',(-0.00143207666897764,-0.0331475787038638,
-0.0142793172582532));
#38645=CARTESIAN_POINT('Ctrl Pts',(-0.000996371926244987,-0.0331778408849578,
-0.0145176499124597));
#38646=CARTESIAN_POINT('Ctrl Pts',(-0.000531036937658981,-0.0332081303637266,
-0.0146188022771925));
#38647=CARTESIAN_POINT('Ctrl Pts',(-0.000356506957828496,-0.0332194908293014,
-0.0146567407959149));
#38648=CARTESIAN_POINT('Ctrl Pts',(-0.000178075723610798,-0.0332308551349036,
-0.0146758516231808));
#38649=CARTESIAN_POINT('Ctrl Pts',(-2.33536370774718E-8,-0.033242224413066,
-0.014675853286449));
#38650=CARTESIAN_POINT('Ctrl Pts',(0.000473652017079301,-0.0332724702730293,
-0.0146758577112661));
#38651=CARTESIAN_POINT('Ctrl Pts',(0.000949299429672487,-0.0333027513251704,
-0.0145369128632183));
#38652=CARTESIAN_POINT('Ctrl Pts',(0.00134930500747653,-0.0333329893848579,
-0.0142804615628886));
#38653=CARTESIAN_POINT('Ctrl Pts',(0.00150055285081224,-0.0333444228287101,
-0.0141834936498199));
#38654=CARTESIAN_POINT('Ctrl Pts',(0.00164113036191268,-0.0333558501259118,
-0.0140702546393804));
#38655=CARTESIAN_POINT('Ctrl Pts',(0.00176775165797444,-0.0333672670498662,
-0.0139436355343841));
#38656=CARTESIAN_POINT('Ctrl Pts',(0.00212865259841615,-0.0333998080103543,
-0.0135827408390023));
#38657=CARTESIAN_POINT('Ctrl Pts',(0.00237540286991301,-0.0334322647000166,
-0.0131089574530919));
#38658=CARTESIAN_POINT('Ctrl Pts',(0.00246315794142062,-0.033465001894446,
-0.0126034663775838));
#38659=CARTESIAN_POINT('Ctrl Pts',(0.00248761842763343,-0.03347412692482,
-0.0124625678828216));
#38660=CARTESIAN_POINT('Ctrl Pts',(0.00249999885738162,-0.0334832737486432,
-0.0123193577753516));
#38661=CARTESIAN_POINT('Ctrl Pts',(0.00249999999992074,-0.0334924502655019,
-0.0121758731935598));
#38662=CARTESIAN_POINT('Ctrl Pts',(0.00250000351370605,-0.0335206718899671,
-0.0117345981383053));
#38663=CARTESIAN_POINT('Ctrl Pts',(0.00237875224282036,-0.0335491743569653,
-0.011286396448637));
#38664=CARTESIAN_POINT('Ctrl Pts',(0.0021511060277031,-0.0335776294465269,
-0.0109019840399007));
#38665=CARTESIAN_POINT('Ctrl Pts',(0.00203917054206178,-0.0335916210442673,
-0.0107129653486114));
#38666=CARTESIAN_POINT('Ctrl Pts',(0.00190236078592673,-0.0336056011872405,
-0.0105392696668422));
#38667=CARTESIAN_POINT('Ctrl Pts',(0.00174662181156177,-0.0336195308554648,
-0.0103871911475904));
#38668=CARTESIAN_POINT('Ctrl Pts',(0.00139879381563512,-0.033650641427511,
-0.0100475384255241));
#38669=CARTESIAN_POINT('Ctrl Pts',(0.000950022516408242,-0.0336815002268697,
-0.00981346098105522));
#38670=CARTESIAN_POINT('Ctrl Pts',(0.000475693111364957,-0.0337122238801269,
-0.00972152729684118));
#38671=CARTESIAN_POINT('Ctrl Pts',(0.000305720759323992,-0.0337232334687206,
-0.00968858355696019));
#38672=CARTESIAN_POINT('Ctrl Pts',(0.000132665409089458,-0.0337342257032983,
-0.0096734345216426));
#38673=CARTESIAN_POINT('Ctrl Pts',(-3.96491736052501E-5,-0.033745205950374,
-0.00967616771772501));
#38674=CARTESIAN_POINT('Ctrl Pts',(-0.000518700898371905,-0.0337757321323009,
-0.00968376627541482));
#38675=CARTESIAN_POINT('Ctrl Pts',(-0.00099485729999462,-0.0338061656633708,
-0.00983333862689195));
#38676=CARTESIAN_POINT('Ctrl Pts',(-0.0013908613543846,-0.0338364750949364,
-0.0100984740017669));
#38677=CARTESIAN_POINT('Ctrl Pts',(-0.00153480325056549,-0.0338474921464119,
-0.0101948469761874));
#38678=CARTESIAN_POINT('Ctrl Pts',(-0.00166833809419712,-0.0338584928016113,
-0.0103060091403367));
#38679=CARTESIAN_POINT('Ctrl Pts',(-0.00178867736678944,-0.0338694755502296,
-0.0104292470694802));
#38680=CARTESIAN_POINT('Ctrl Pts',(-0.00212827609129081,-0.0339004689852232,
-0.0107770258340161));
#38681=CARTESIAN_POINT('Ctrl Pts',(-0.00236269258968325,-0.0339313198167728,
-0.0112261021386227));
#38682=CARTESIAN_POINT('Ctrl Pts',(-0.00245456493483844,-0.0339620393589644,
-0.0117013946680659));
#38683=CARTESIAN_POINT('Ctrl Pts',(-0.00248481221025082,-0.0339721532017279,
-0.0118578759684531));
#38684=CARTESIAN_POINT('Ctrl Pts',(-0.00250000044750102,-0.0339822528135889,
-0.0120170244069798));
#38685=CARTESIAN_POINT('Ctrl Pts',(-0.00249999999999008,-0.0339923385983081,
-0.0121758603301622));
#38686=CARTESIAN_POINT('',(-0.00214231189934805,-0.034078774338657,-0.0134644570759021));
#38687=CARTESIAN_POINT('Ctrl Pts',(-0.00249999938363598,-0.0339924495244571,
-0.0121776087977965));
#38688=CARTESIAN_POINT('Ctrl Pts',(-0.00249968291142358,-0.0340212244625237,
-0.0126282925180976));
#38689=CARTESIAN_POINT('Ctrl Pts',(-0.00237461305321147,-0.0340499994005904,
-0.0130782549408287));
#38690=CARTESIAN_POINT('Ctrl Pts',(-0.00214231189934805,-0.034078774338657,
-0.0134644570759021));
#38691=CARTESIAN_POINT('',(-0.000601546286298526,-0.0340787743898723,-0.00974930387114525));
#38692=CARTESIAN_POINT('Origin',(0.,-0.0340787743898623,-0.0121758532865581));
#38693=CARTESIAN_POINT('Ctrl Pts',(-0.000601546286299171,-0.0340787743898619,
-0.00974930387114541));
#38694=CARTESIAN_POINT('Ctrl Pts',(-0.000126738896636988,-0.034047633898331,
-0.00963159820228718));
#38695=CARTESIAN_POINT('Ctrl Pts',(0.000383109996741683,-0.0340164934068,
-0.00965749571553324));
#38696=CARTESIAN_POINT('Ctrl Pts',(0.000843239392728706,-0.033985352915269,
-0.00982235645704026));
#38697=CARTESIAN_POINT('Ctrl Pts',(0.000868642157086713,-0.0339836337150283,
-0.00983145806759789));
#38698=CARTESIAN_POINT('Ctrl Pts',(0.000893894990357826,-0.0339819145147875,
-0.00984097008168301));
#38699=CARTESIAN_POINT('Ctrl Pts',(0.000918984538856573,-0.0339801953145468,
-0.00985088717554861));
#38700=CARTESIAN_POINT('Ctrl Pts',(0.00136814293774854,-0.0339494178285532,
-0.0100284250855098));
#38701=CARTESIAN_POINT('Ctrl Pts',(0.00176464235916692,-0.0339186403425595,
-0.0103402207080788));
#38702=CARTESIAN_POINT('Ctrl Pts',(0.00204312011347985,-0.0338878628565659,
-0.0107351381162715));
#38703=CARTESIAN_POINT('Ctrl Pts',(0.00206196011845155,-0.0338857806507877,
-0.0107618556756403));
#38704=CARTESIAN_POINT('Ctrl Pts',(0.00208027315665946,-0.0338836984450094,
-0.0107889388407447));
#38705=CARTESIAN_POINT('Ctrl Pts',(0.00209804524141437,-0.0338816162392312,
-0.0108163658224826));
#38706=CARTESIAN_POINT('Ctrl Pts',(0.00236143596159679,-0.0338507569626153,
-0.0112228466924531));
#38707=CARTESIAN_POINT('Ctrl Pts',(0.00250323127272012,-0.0338198976859994,
-0.0117083446996253));
#38708=CARTESIAN_POINT('Ctrl Pts',(0.00249994239779229,-0.0337890384093834,
-0.0121928240767732));
#38709=CARTESIAN_POINT('Ctrl Pts',(0.00249972920046646,-0.0337870379942275,
-0.0122242298644343));
#38710=CARTESIAN_POINT('Ctrl Pts',(0.0024989241470306,-0.0337850375790716,
-0.0122556273663398));
#38711=CARTESIAN_POINT('Ctrl Pts',(0.00249752833899235,-0.0337830371639157,
-0.0122869937199302));
#38712=CARTESIAN_POINT('Ctrl Pts',(0.00247600395694093,-0.0337521892973773,
-0.0127706858607799));
#38713=CARTESIAN_POINT('Ctrl Pts',(0.00230970703782302,-0.0337213414308389,
-0.0132481441899844));
#38714=CARTESIAN_POINT('Ctrl Pts',(0.00202594814670806,-0.0336904935643004,
-0.0136406174678686));
#38715=CARTESIAN_POINT('Ctrl Pts',(0.00200744205985623,-0.033688481739067,
-0.0136662136510895));
#38716=CARTESIAN_POINT('Ctrl Pts',(0.00198845339528052,-0.0336864699138336,
-0.0136914555244219));
#38717=CARTESIAN_POINT('Ctrl Pts',(0.00196899657661983,-0.0336844580886002,
-0.0137163247991994));
#38718=CARTESIAN_POINT('Ctrl Pts',(0.00167065985465431,-0.0336536102220617,
-0.0140976521911113));
#38719=CARTESIAN_POINT('Ctrl Pts',(0.00125806506077489,-0.0336227623555233,
-0.01438986140707));
#38720=CARTESIAN_POINT('Ctrl Pts',(0.000799163142138323,-0.0335919144889848,
-0.0145446796356702));
#38721=CARTESIAN_POINT('Ctrl Pts',(0.00076923463935431,-0.0335899026637514,
-0.0145547765160655));
#38722=CARTESIAN_POINT('Ctrl Pts',(0.00073911888749589,-0.033587890838518,
-0.0145643047397628));
#38723=CARTESIAN_POINT('Ctrl Pts',(0.000708838248187203,-0.0335858790132846,
-0.0145732577868264));
#38724=CARTESIAN_POINT('Ctrl Pts',(0.000244365187101707,-0.0335550197366687,
-0.0147105880833672));
#38725=CARTESIAN_POINT('Ctrl Pts',(-0.000261412390778464,-0.0335241604600528,
-0.0147089147516458));
#38726=CARTESIAN_POINT('Ctrl Pts',(-0.000725083512180734,-0.0334933011834368,
-0.0145683945924426));
#38727=CARTESIAN_POINT('Ctrl Pts',(-0.00075514042991596,-0.0334913007682809,
-0.0145592855436571));
#38728=CARTESIAN_POINT('Ctrl Pts',(-0.000785021614133495,-0.033489300353125,
-0.014549611254258));
#38729=CARTESIAN_POINT('Ctrl Pts',(-0.0008147054510334,-0.0334872999379691,
-0.014539379260195));
#38730=CARTESIAN_POINT('Ctrl Pts',(-0.00127140758694842,-0.0334565224519755,
-0.0143819544111438));
#38731=CARTESIAN_POINT('Ctrl Pts',(-0.00168135115512026,-0.0334257449659819,
-0.0140880467024281));
#38732=CARTESIAN_POINT('Ctrl Pts',(-0.00197705569024059,-0.0333949674799883,
-0.0137059679220307));
#38733=CARTESIAN_POINT('Ctrl Pts',(-0.00199706114785999,-0.0333928852742101,
-0.0136801189412384));
#38734=CARTESIAN_POINT('Ctrl Pts',(-0.00201655633294717,-0.0333908030684318,
-0.0136538817710384));
#38735=CARTESIAN_POINT('Ctrl Pts',(-0.00203552635298372,-0.0333887208626536,
-0.0136272775754236));
#38736=CARTESIAN_POINT('Ctrl Pts',(-0.00231923306173773,-0.0333575803711226,
-0.0132293977227732));
#38737=CARTESIAN_POINT('Ctrl Pts',(-0.00248283147535909,-0.0333264398795917,
-0.0127458468591014));
#38738=CARTESIAN_POINT('Ctrl Pts',(-0.00249868674944542,-0.0332952993880607,
-0.0122568750623093));
#38739=CARTESIAN_POINT('Ctrl Pts',(-0.00249956208537264,-0.0332935801878198,
-0.0122298799704049));
#38740=CARTESIAN_POINT('Ctrl Pts',(-0.00249999986943493,-0.0332918609875789,
-0.012202871934591));
#38741=CARTESIAN_POINT('Ctrl Pts',(-0.0024999999999708,-0.033290141787338,
-0.0121758653702745));
#38742=CARTESIAN_POINT('Origin',(0.,-0.0342787743898723,-0.0121758532865581));
#38743=CARTESIAN_POINT('',(-0.00299999988642399,-0.031703806066922,-0.0121752798029594));
#38744=CARTESIAN_POINT('',(-0.00299999939184732,-0.0307036990116105,-0.0121771829558748));
#38745=CARTESIAN_POINT('Ctrl Pts',(-0.00299999977291662,-0.0317037743898623,
-0.0121746860247103));
#38746=CARTESIAN_POINT('Ctrl Pts',(-0.00299978312826752,-0.0316742289770476,
-0.0116178838818835));
#38747=CARTESIAN_POINT('Ctrl Pts',(-0.00284025273261327,-0.0316446835642328,
-0.0110610251285104));
#38748=CARTESIAN_POINT('Ctrl Pts',(-0.00254573842885079,-0.0316151381514181,
-0.0105886495025807));
#38749=CARTESIAN_POINT('Ctrl Pts',(-0.00242491146118173,-0.0316030168975662,
-0.0103948534330767));
#38750=CARTESIAN_POINT('Ctrl Pts',(-0.00228196716891504,-0.0315908956437142,
-0.0102151071015685));
#38751=CARTESIAN_POINT('Ctrl Pts',(-0.00212084111800276,-0.0315787743898623,
-0.0100540538256785));
#38752=CARTESIAN_POINT('Ctrl Pts',(-0.00173533258476648,-0.0315497732024876,
-0.00966871941321266));
#38753=CARTESIAN_POINT('Ctrl Pts',(-0.00124021229841889,-0.031520772015113,
-0.00938998950206325));
#38754=CARTESIAN_POINT('Ctrl Pts',(-0.000708736353863526,-0.0314917708277383,
-0.00926077305083349));
#38755=CARTESIAN_POINT('Ctrl Pts',(-0.000476628699683858,-0.0314791053484463,
-0.00920434128250303));
#38756=CARTESIAN_POINT('Ctrl Pts',(-0.000237958547009543,-0.0314664398691543,
-0.0091758383654527));
#38757=CARTESIAN_POINT('Ctrl Pts',(1.88039627964167E-7,-0.0314537743898623,
-0.00917585329245125));
#38758=CARTESIAN_POINT('Ctrl Pts',(0.000547508419203228,-0.0314246659527796,
-0.00917588759842483));
#38759=CARTESIAN_POINT('Ctrl Pts',(0.00109662914758601,-0.0313955575156969,
-0.00933003319063454));
#38760=CARTESIAN_POINT('Ctrl Pts',(0.00156492802349207,-0.0313664490786142,
-0.00961636109448382));
#38761=CARTESIAN_POINT('Ctrl Pts',(0.00176696583063482,-0.0313538908490302,
-0.00973989131160331));
#38762=CARTESIAN_POINT('Ctrl Pts',(0.00195411565321174,-0.0313413326194463,
-0.00988736184395037));
#38763=CARTESIAN_POINT('Ctrl Pts',(0.00212110708959182,-0.0313287743898623,
-0.0100543197104667));
#38764=CARTESIAN_POINT('Ctrl Pts',(0.00250809996203972,-0.0312996714283877,
-0.0104412347867216));
#38765=CARTESIAN_POINT('Ctrl Pts',(0.00278743908090049,-0.0312705684669131,
-0.0109383763719027));
#38766=CARTESIAN_POINT('Ctrl Pts',(0.00291622376994772,-0.0312414655054385,
-0.0114718370057862));
#38767=CARTESIAN_POINT('Ctrl Pts',(0.00297181992870467,-0.0312289018002464,
-0.0117021311681698));
#38768=CARTESIAN_POINT('Ctrl Pts',(0.00299993759600436,-0.0312163380950544,
-0.0119388347240268));
#38769=CARTESIAN_POINT('Ctrl Pts',(0.00299999989567168,-0.0312037743898623,
-0.0121750621039462));
#38770=CARTESIAN_POINT('Ctrl Pts',(0.00300014420857858,-0.0311746714283877,
-0.0127222666293588));
#38771=CARTESIAN_POINT('Ctrl Pts',(0.00284624088932268,-0.0311455684669131,
-0.0132713404189909));
#38772=CARTESIAN_POINT('Ctrl Pts',(0.00256016617521376,-0.0311164655054385,
-0.0137396784543091));
#38773=CARTESIAN_POINT('Ctrl Pts',(0.00243666814653024,-0.0311039018002464,
-0.0139418592877304));
#38774=CARTESIAN_POINT('Ctrl Pts',(0.00228920193131261,-0.0310913380950544,
-0.0141291490201574));
#38775=CARTESIAN_POINT('Ctrl Pts',(0.00212222580814811,-0.0310787743898623,
-0.0142962677788756));
#38776=CARTESIAN_POINT('Ctrl Pts',(0.00173536429706138,-0.0310496659527796,
-0.0146834597576052));
#38777=CARTESIAN_POINT('Ctrl Pts',(0.00123820729474145,-0.0310205575156969,
-0.0149629884269283));
#38778=CARTESIAN_POINT('Ctrl Pts',(0.000704674944244704,-0.0309914490786142,
-0.0150919179674172));
#38779=CARTESIAN_POINT('Ctrl Pts',(0.000474493511659587,-0.0309788908490302,
-0.0151475419353071));
#38780=CARTESIAN_POINT('Ctrl Pts',(0.000237900354987811,-0.0309663326194463,
-0.0151757134156151));
#38781=CARTESIAN_POINT('Ctrl Pts',(1.77040476739121E-6,-0.0309537743898623,
-0.0151758527641692));
#38782=CARTESIAN_POINT('Ctrl Pts',(-0.000543533285161779,-0.0309247732024876,
-0.015176174566976));
#38783=CARTESIAN_POINT('Ctrl Pts',(-0.00109089993736176,-0.030895772015113,
-0.0150234838642021));
#38784=CARTESIAN_POINT('Ctrl Pts',(-0.00155821273132624,-0.0308667708277383,
-0.014739439267939));
#38785=CARTESIAN_POINT('Ctrl Pts',(-0.00176229887574436,-0.0308541053484463,
-0.0146153905210551));
#38786=CARTESIAN_POINT('Ctrl Pts',(-0.00195127257021304,-0.0308414398691543,
-0.0144669665921402));
#38787=CARTESIAN_POINT('Ctrl Pts',(-0.00211972166913044,-0.0308287743898623,
-0.0142987711006571));
#38788=CARTESIAN_POINT('Ctrl Pts',(-0.00251267151737878,-0.0307992289770476,
-0.0139064128554713));
#38789=CARTESIAN_POINT('Ctrl Pts',(-0.0027945897162608,-0.0307696835642329,
-0.0134009438838064));
#38790=CARTESIAN_POINT('Ctrl Pts',(-0.00292135667822606,-0.0307401381514181,
-0.0128582572421328));
#38791=CARTESIAN_POINT('Ctrl Pts',(-0.00297336388948608,-0.0307280168975662,
-0.012635615487657));
#38792=CARTESIAN_POINT('Ctrl Pts',(-0.00299978937163709,-0.0307158956437142,
-0.0124070355920604));
#38793=CARTESIAN_POINT('Ctrl Pts',(-0.00299999873992521,-0.0307037743898623,
-0.0121786029132924));
#38794=CARTESIAN_POINT('',(-0.00299999999999987,-0.0297037907762723,-0.0121758524173738));
#38795=CARTESIAN_POINT('Ctrl Pts',(-0.00299999999999574,-0.0307036286946763,
-0.0121758583423425));
#38796=CARTESIAN_POINT('Ctrl Pts',(-0.00300000093834573,-0.0306740944474691,
-0.0116190604763335));
#38797=CARTESIAN_POINT('Ctrl Pts',(-0.00284069050734933,-0.0306445602002618,
-0.0110621430487859));
#38798=CARTESIAN_POINT('Ctrl Pts',(-0.00254636475893709,-0.0306150259530546,
-0.0105896545239677));
#38799=CARTESIAN_POINT('Ctrl Pts',(-0.00242552546022251,-0.0306029002802589,
-0.0103956681592079));
#38800=CARTESIAN_POINT('Ctrl Pts',(-0.00228253061514852,-0.0305907746074633,
-0.010215743637405));
#38801=CARTESIAN_POINT('Ctrl Pts',(-0.00212132312544701,-0.0305786489346676,
-0.0100545357248895));
#38802=CARTESIAN_POINT('Ctrl Pts',(-0.00173590887930689,-0.0305496589228007,
-0.00966912046788729));
#38803=CARTESIAN_POINT('Ctrl Pts',(-0.00124086089003451,-0.0305206689109338,
-0.00939027980684245));
#38804=CARTESIAN_POINT('Ctrl Pts',(-0.000709422677418312,-0.0304916788990669,
-0.0092609400005812));
#38805=CARTESIAN_POINT('Ctrl Pts',(-0.000477160843076479,-0.0304790089909309,
-0.00920441282593983));
#38806=CARTESIAN_POINT('Ctrl Pts',(-0.000238320408519796,-0.0304663390827949,
-0.00917585350998904));
#38807=CARTESIAN_POINT('Ctrl Pts',(-2.81258648426431E-9,-0.0304536691746589,
-0.00917585328655942));
#38808=CARTESIAN_POINT('Ctrl Pts',(0.000547308636665276,-0.0304245719283702,
-0.00917585277343916));
#38809=CARTESIAN_POINT('Ctrl Pts',(0.0010964320589705,-0.0303954746820815,
-0.00932995861975189));
#38810=CARTESIAN_POINT('Ctrl Pts',(0.00156474531708854,-0.0303663774357928,
-0.00961624939285707));
#38811=CARTESIAN_POINT('Ctrl Pts',(0.00176693856243628,-0.0303538147620786,
-0.00973985482047163));
#38812=CARTESIAN_POINT('Ctrl Pts',(0.00195422378185452,-0.0303412520883644,
-0.00988743656966469));
#38813=CARTESIAN_POINT('Ctrl Pts',(0.00212131914785055,-0.0303286894146501,
-0.01005453174729));
#38814=CARTESIAN_POINT('Ctrl Pts',(0.00250826720070462,-0.0302995976316232,
-0.0104414793639281));
#38815=CARTESIAN_POINT('Ctrl Pts',(0.00278755503992261,-0.0302705058485962,
-0.0109386406709272));
#38816=CARTESIAN_POINT('Ctrl Pts',(0.00291628881227279,-0.0302414140655693,
-0.0114721064830751));
#38817=CARTESIAN_POINT('Ctrl Pts',(0.0029719039556564,-0.0302288459285933,
-0.011702572638857));
#38818=CARTESIAN_POINT('Ctrl Pts',(0.00299999995513255,-0.0302162777916174,
-0.0119394549660179));
#38819=CARTESIAN_POINT('Ctrl Pts',(0.00299999999999995,-0.0302037096546414,
-0.0121758527171695));
#38820=CARTESIAN_POINT('Ctrl Pts',(0.00300000010385564,-0.0301746178716145,
-0.0127230485424311));
#38821=CARTESIAN_POINT('Ctrl Pts',(0.00284595678365275,-0.0301455260885875,
-0.0132720748242642));
#38822=CARTESIAN_POINT('Ctrl Pts',(0.00255976580244818,-0.0301164343055606,
-0.0137403337231941));
#38823=CARTESIAN_POINT('Ctrl Pts',(0.00243612651056531,-0.0301038661685846,
-0.013942629401548));
#38824=CARTESIAN_POINT('Ctrl Pts',(0.00228848792214319,-0.0300912980316087,
-0.0141300061130754));
#38825=CARTESIAN_POINT('Ctrl Pts',(0.00212131995308795,-0.0300787298946327,
-0.0142971740205894));
#38826=CARTESIAN_POINT('Ctrl Pts',(0.001734299380629,-0.030049632648344,
-0.0146841944505705));
#38827=CARTESIAN_POINT('Ctrl Pts',(0.00123703143457719,-0.0300205354020554,
-0.0149635091150117));
#38828=CARTESIAN_POINT('Ctrl Pts',(0.000703451975723402,-0.0299914381557667,
-0.0150922132296808));
#38829=CARTESIAN_POINT('Ctrl Pts',(0.00047308018810817,-0.0299788754820525,
-0.0151477809553078));
#38830=CARTESIAN_POINT('Ctrl Pts',(0.000236298871225366,-0.0299663128083382,
-0.0151758534183983));
#38831=CARTESIAN_POINT('Ctrl Pts',(-1.67380927159913E-9,-0.029953750134624,
-0.0151758532865576));
#38832=CARTESIAN_POINT('Ctrl Pts',(-0.000545296072162418,-0.0299247601227571,
-0.015175852982318));
#38833=CARTESIAN_POINT('Ctrl Pts',(-0.00109256494565921,-0.0298957701108902,
-0.0150228440193565));
#38834=CARTESIAN_POINT('Ctrl Pts',(-0.00155970580473139,-0.0298667800990233,
-0.0147385311443247));
#38835=CARTESIAN_POINT('Ctrl Pts',(-0.0017638668722805,-0.0298541101908873,
-0.0146142739337699));
#38836=CARTESIAN_POINT('Ctrl Pts',(-0.00195287930718518,-0.0298414402827513,
-0.014465614980402));
#38837=CARTESIAN_POINT('Ctrl Pts',(-0.00212132232021082,-0.0298287703746153,
-0.0142971716534647));
#38838=CARTESIAN_POINT('Ctrl Pts',(-0.00251397211262461,-0.0297992361320834,
-0.0139045211293059));
#38839=CARTESIAN_POINT('Ctrl Pts',(-0.00279550818297967,-0.0297697018895515,
-0.0133988448080529));
#38840=CARTESIAN_POINT('Ctrl Pts',(-0.00292186740455529,-0.0297401676470197,
-0.0128560671280795));
#38841=CARTESIAN_POINT('Ctrl Pts',(-0.00297374563895877,-0.0297280420234372,
-0.0126332234973613));
#38842=CARTESIAN_POINT('Ctrl Pts',(-0.00300000006623164,-0.0297159163998547,
-0.0124044521585));
#38843=CARTESIAN_POINT('Ctrl Pts',(-0.00299999999999987,-0.0297037907762723,
-0.0121758524173738));
#38844=CARTESIAN_POINT('',(0.00267183091333631,-0.0292787743898623,-0.0108115514246007));
#38845=CARTESIAN_POINT('Ctrl Pts',(-0.00299999998382998,-0.0297037743898623,
-0.0121755418060137));
#38846=CARTESIAN_POINT('Ctrl Pts',(-0.00299994185979298,-0.0296740643174192,
-0.0116157247863023));
#38847=CARTESIAN_POINT('Ctrl Pts',(-0.00283892252328663,-0.0296443542449761,
-0.0110562397396311));
#38848=CARTESIAN_POINT('Ctrl Pts',(-0.00254172294431946,-0.029614644172533,
-0.0105822270837364));
#38849=CARTESIAN_POINT('Ctrl Pts',(-0.00248463801449189,-0.0296089375783095,
-0.0104911805913653));
#38850=CARTESIAN_POINT('Ctrl Pts',(-0.00242267577881712,-0.0296032309840859,
-0.0104032360322616));
#38851=CARTESIAN_POINT('Ctrl Pts',(-0.0023562110315139,-0.0295975243898623,
-0.010318901597641));
#38852=CARTESIAN_POINT('Ctrl Pts',(-0.00201476491589461,-0.0295682081807422,
-0.00988565440597122));
#38853=CARTESIAN_POINT('Ctrl Pts',(-0.0015498817289811,-0.029538891971622,
-0.00954850647314129));
#38854=CARTESIAN_POINT('Ctrl Pts',(-0.00103119238248645,-0.0295095757625019,
-0.00935864859568065));
#38855=CARTESIAN_POINT('Ctrl Pts',(-0.000923257474355454,-0.0295034753049554,
-0.0093191407617524));
#38856=CARTESIAN_POINT('Ctrl Pts',(-0.000813093493369863,-0.0294973748474088,
-0.00928585976408999));
#38857=CARTESIAN_POINT('Ctrl Pts',(-0.000701456466827434,-0.0294912743898623,
-0.00925901273124042));
#38858=CARTESIAN_POINT('Ctrl Pts',(-0.00016497631092072,-0.0294619581807422,
-0.00912999728882986));
#38859=CARTESIAN_POINT('Ctrl Pts',(0.000408862167047048,-0.029432641971622,
-0.00915297278038173));
#38860=CARTESIAN_POINT('Ctrl Pts',(0.000933680525875383,-0.0294033257625019,
-0.0093248463283763));
#38861=CARTESIAN_POINT('Ctrl Pts',(0.00104289083013255,-0.0293972253049554,
-0.00936061177399095));
#38862=CARTESIAN_POINT('Ctrl Pts',(0.00114999357473004,-0.0293911248474088,
-0.00940264375250374));
#38863=CARTESIAN_POINT('Ctrl Pts',(0.00125426789939748,-0.0293850243898623,
-0.00945063549039189));
#38864=CARTESIAN_POINT('Ctrl Pts',(0.0017620982901821,-0.0293553143174192,
-0.00968436189508353));
#38865=CARTESIAN_POINT('Ctrl Pts',(0.00220321097255991,-0.0293256042449762,
-0.0100641074196941));
#38866=CARTESIAN_POINT('Ctrl Pts',(0.00250994897180209,-0.0292958941725331,
-0.0105326380970745));
#38867=CARTESIAN_POINT('Ctrl Pts',(0.00256886600399653,-0.0292901875783095,
-0.010622631632507));
#38868=CARTESIAN_POINT('Ctrl Pts',(0.00262293094262228,-0.0292844809840859,
-0.0107157863618546));
#38869=CARTESIAN_POINT('Ctrl Pts',(0.00267183091333631,-0.0292787743898623,
-0.0108115514246007));
#38870=CARTESIAN_POINT('',(0.000927050983124848,-0.0292787743898723,-0.00932268373767264));
#38871=CARTESIAN_POINT('Origin',(0.,-0.0292787743898623,-0.0121758532865581));
#38872=CARTESIAN_POINT('',(-0.00299999932318279,-0.0295787743898623,-0.0121778684547369));
#38873=CARTESIAN_POINT('Ctrl Pts',(0.000927050983124362,-0.0292787743898627,
-0.00932268373767248));
#38874=CARTESIAN_POINT('Ctrl Pts',(0.000403615972859334,-0.029307962090938,
-0.0091526093931396));
#38875=CARTESIAN_POINT('Ctrl Pts',(-0.00016905585335949,-0.0293371497920133,
-0.00913038402760189));
#38876=CARTESIAN_POINT('Ctrl Pts',(-0.00108600803646328,-0.0293871316591116,
-0.00935191796589178));
#38877=CARTESIAN_POINT('Ctrl Pts',(-0.00144812628843063,-0.0294079258251344,
-0.009519776883436));
#38878=CARTESIAN_POINT('Ctrl Pts',(-0.00220580055780451,-0.0294579076922327,
-0.0100702541868122));
#38879=CARTESIAN_POINT('Ctrl Pts',(-0.0025605860953725,-0.0294870953933081,
-0.0105182936949274));
#38880=CARTESIAN_POINT('Ctrl Pts',(-0.00292197599480409,-0.0295370772604064,
-0.0113907378054678));
#38881=CARTESIAN_POINT('Ctrl Pts',(-0.00299999642597719,-0.0295578714264294,
-0.0117837248437925));
#38882=CARTESIAN_POINT('Ctrl Pts',(-0.00299999999987538,-0.0295786655924524,
-0.0121758259423486));
#38883=CARTESIAN_POINT('',(-0.00299999937953697,-0.0305788301727905,-0.0121743809549774));
#38884=CARTESIAN_POINT('Ctrl Pts',(-0.00299999932318279,-0.0295787743898623,
-0.0121778684547369));
#38885=CARTESIAN_POINT('Ctrl Pts',(-0.00299962530604328,-0.0296083208102491,
-0.0127346711956747));
#38886=CARTESIAN_POINT('Ctrl Pts',(-0.00283993715789012,-0.0296378672306359,
-0.0132914854094396));
#38887=CARTESIAN_POINT('Ctrl Pts',(-0.00254528873352183,-0.0296674136510226,
-0.0137637781157005));
#38888=CARTESIAN_POINT('Ctrl Pts',(-0.00242442091188463,-0.0296795338973025,
-0.0139575174533646));
#38889=CARTESIAN_POINT('Ctrl Pts',(-0.00228144489908848,-0.0296916541435824,
-0.0141372040791591));
#38890=CARTESIAN_POINT('Ctrl Pts',(-0.00212029612942546,-0.0297037743898623,
-0.0142981973499803));
#38891=CARTESIAN_POINT('Ctrl Pts',(-0.00173468758494504,-0.0297327766002826,
-0.014683433805476));
#38892=CARTESIAN_POINT('Ctrl Pts',(-0.00123949431793212,-0.0297617788107028,
-0.0149620368237008));
#38893=CARTESIAN_POINT('Ctrl Pts',(-0.000707983886383787,-0.0297907810211231,
-0.0150911163650162));
#38894=CARTESIAN_POINT('Ctrl Pts',(-0.000475888107913542,-0.0298034454773695,
-0.0151474817999126));
#38895=CARTESIAN_POINT('Ctrl Pts',(-0.000237238539839443,-0.0298161099336159,
-0.0151759230887667));
#38896=CARTESIAN_POINT('Ctrl Pts',(8.81047802455638E-7,-0.0298287743898623,
-0.0151758531571839));
#38897=CARTESIAN_POINT('Ctrl Pts',(0.00054820281424355,-0.0298578838496612,
-0.0151756924182971));
#38898=CARTESIAN_POINT('Ctrl Pts',(0.0010972890419145,-0.0298869933094601,
-0.0150214192221399));
#38899=CARTESIAN_POINT('Ctrl Pts',(0.00156552236723977,-0.029916102769259,
-0.0147349819893927));
#38900=CARTESIAN_POINT('Ctrl Pts',(0.0017675083459938,-0.0299286599761268,
-0.0146114190098294));
#38901=CARTESIAN_POINT('Ctrl Pts',(0.00195460421385389,-0.0299412171829946,
-0.0144639246845766));
#38902=CARTESIAN_POINT('Ctrl Pts',(0.00212154235467162,-0.0299537743898623,
-0.0142969515957683));
#38903=CARTESIAN_POINT('Ctrl Pts',(0.00250845679834444,-0.0299828783722448,
-0.0139099561527368));
#38904=CARTESIAN_POINT('Ctrl Pts',(0.00278769415448554,-0.0300119823546272,
-0.0134127559676335));
#38905=CARTESIAN_POINT('Ctrl Pts',(0.00291636900172886,-0.0300410863370097,
-0.0128792677061963));
#38906=CARTESIAN_POINT('Ctrl Pts',(0.00297191127975778,-0.0300536490212939,
-0.012648988409374));
#38907=CARTESIAN_POINT('Ctrl Pts',(0.00299998006402622,-0.0300662117055781,
-0.0124123068592859));
#38908=CARTESIAN_POINT('Ctrl Pts',(0.0029999999893257,-0.0300787743898623,
-0.0121761063592579));
#38909=CARTESIAN_POINT('Ctrl Pts',(0.00300004615028558,-0.0301078783722448,
-0.0116289004408389));
#38910=CARTESIAN_POINT('Ctrl Pts',(0.00284604360528892,-0.0301369823546272,
-0.011079853172088));
#38911=CARTESIAN_POINT('Ctrl Pts',(0.00255988376205479,-0.0301660863370097,
-0.010611565868988));
#38912=CARTESIAN_POINT('Ctrl Pts',(0.00243636335449944,-0.0301786490212939,
-0.0104094304544652));
#38913=CARTESIAN_POINT('Ctrl Pts',(0.00228888295904802,-0.0301912117055781,
-0.0102221870407097));
#38914=CARTESIAN_POINT('Ctrl Pts',(0.0021219001858595,-0.0302037743898623,
-0.0100551129438359));
#38915=CARTESIAN_POINT('Ctrl Pts',(0.00173497823404734,-0.0302328838496612,
-0.00966797938253934));
#38916=CARTESIAN_POINT('Ctrl Pts',(0.00123777698915588,-0.0302619933094601,
-0.00938852679820759));
#38917=CARTESIAN_POINT('Ctrl Pts',(0.000704223598844007,-0.030291102769259,
-0.00925967957382575));
#38918=CARTESIAN_POINT('Ctrl Pts',(0.000474059922038583,-0.0303036599761268,
-0.00920409759937224));
#38919=CARTESIAN_POINT('Ctrl Pts',(0.000237490241918617,-0.0303162171829945,
-0.00917596278079916));
#38920=CARTESIAN_POINT('Ctrl Pts',(1.38719316590359E-6,-0.0303287743898623,
-0.0091758536072756));
#38921=CARTESIAN_POINT('Ctrl Pts',(-0.000543918014664728,-0.0303577766002826,
-0.00917560145936276));
#38922=CARTESIAN_POINT('Ctrl Pts',(-0.00109126634046794,-0.0303867788107028,
-0.00932836287458711));
#38923=CARTESIAN_POINT('Ctrl Pts',(-0.00155854349046879,-0.0304157810211231,
-0.00961246837821574));
#38924=CARTESIAN_POINT('Ctrl Pts',(-0.00176259038673546,-0.0304284454773695,
-0.00973652932625824));
#38925=CARTESIAN_POINT('Ctrl Pts',(-0.00195152515402665,-0.0304411099336159,
-0.00988495792512666));
#38926=CARTESIAN_POINT('Ctrl Pts',(-0.00211993802768848,-0.0304537743898623,
-0.0100531515272993));
#38927=CARTESIAN_POINT('Ctrl Pts',(-0.00251284850619159,-0.030483320810249,
-0.0104455504411943));
#38928=CARTESIAN_POINT('Ctrl Pts',(-0.00279471530702616,-0.0305128672306358,
-0.0109510489415062));
#38929=CARTESIAN_POINT('Ctrl Pts',(-0.00292142670497378,-0.0305424136510226,
-0.011493749183458));
#38930=CARTESIAN_POINT('Ctrl Pts',(-0.002973405026865,-0.0305545338973025,
-0.011716370418197));
#38931=CARTESIAN_POINT('Ctrl Pts',(-0.00299980697922492,-0.0305666541435824,
-0.011944925777034));
#38932=CARTESIAN_POINT('Ctrl Pts',(-0.00299999894049624,-0.0305787743898623,
-0.0121733319731243));
#38933=CARTESIAN_POINT('',(-0.00299999999999953,-0.0315788060372049,-0.0121758516139528));
#38934=CARTESIAN_POINT('Ctrl Pts',(-0.00299999999998308,-0.0305789090044302,
-0.0121758633611915));
#38935=CARTESIAN_POINT('Ctrl Pts',(-0.002999998130136,-0.0306084450666598,
-0.0127326619098351));
#38936=CARTESIAN_POINT('Ctrl Pts',(-0.00284068451932866,-0.0306379811288893,
-0.0132895791065831));
#38937=CARTESIAN_POINT('Ctrl Pts',(-0.00254635576498619,-0.0306675171911189,
-0.0137620664872728));
#38938=CARTESIAN_POINT('Ctrl Pts',(-0.00242552940725285,-0.0306796421866157,
-0.0139560296269302));
#38939=CARTESIAN_POINT('Ctrl Pts',(-0.00228255274909621,-0.0306917671821125,
-0.0141359340922567));
#38940=CARTESIAN_POINT('Ctrl Pts',(-0.00212136726850902,-0.0307038921776093,
-0.0142971267041303));
#38941=CARTESIAN_POINT('Ctrl Pts',(-0.00173595997884731,-0.0307328840051272,
-0.0146825510452645));
#38942=CARTESIAN_POINT('Ctrl Pts',(-0.0012409163762974,-0.0307618758326452,
-0.0149614022816779));
#38943=CARTESIAN_POINT('Ctrl Pts',(-0.000709479533810012,-0.0307908676601631,
-0.015090752734413));
#38944=CARTESIAN_POINT('Ctrl Pts',(-0.0004772452707397,-0.0308035368903715,
-0.0151472779969976));
#38945=CARTESIAN_POINT('Ctrl Pts',(-0.000238433368114515,-0.0308162061205799,
-0.0151758419405363));
#38946=CARTESIAN_POINT('Ctrl Pts',(-1.42799900971172E-7,-0.0308288753507883,
-0.0151758532831595));
#38947=CARTESIAN_POINT('Ctrl Pts',(0.000547170060450925,-0.0308579744153287,
-0.0151758793352336));
#38948=CARTESIAN_POINT('Ctrl Pts',(0.00109630179715439,-0.0308870734798691,
-0.0150217983519956));
#38949=CARTESIAN_POINT('Ctrl Pts',(0.00156462901955293,-0.0309161725444094,
-0.0147355282720148));
#38950=CARTESIAN_POINT('Ctrl Pts',(0.00176680470696733,-0.0309287345375954,
-0.0146119461964099));
#38951=CARTESIAN_POINT('Ctrl Pts',(0.00195407689624954,-0.0309412965307813,
-0.0144643926465557));
#38952=CARTESIAN_POINT('Ctrl Pts',(0.00212116531380692,-0.0309538585239673,
-0.0142973286485414));
#38953=CARTESIAN_POINT('Ctrl Pts',(0.00250814239611413,-0.0309829521232851,
-0.0139104081219411));
#38954=CARTESIAN_POINT('Ctrl Pts',(0.00278746653687675,-0.0310120457226029,
-0.0134132657730967));
#38955=CARTESIAN_POINT('Ctrl Pts',(0.00291623861273731,-0.0310411393219208,
-0.0128798080816835));
#38956=CARTESIAN_POINT('Ctrl Pts',(0.00297186382740656,-0.0310537067803293,
-0.0126493722639526));
#38957=CARTESIAN_POINT('Ctrl Pts',(0.00299997668915932,-0.0310662742387378,
-0.0124125197856121));
#38958=CARTESIAN_POINT('Ctrl Pts',(0.00299999998542944,-0.0310788416971463,
-0.0121761489609931));
#38959=CARTESIAN_POINT('Ctrl Pts',(0.00300005391617075,-0.0311079352964641,
-0.0116289517602262));
#38960=CARTESIAN_POINT('Ctrl Pts',(0.00284606386147954,-0.031137028895782,
-0.0110799092327468));
#38961=CARTESIAN_POINT('Ctrl Pts',(0.00255991781383716,-0.0311661224950998,
-0.0106116215945127));
#38962=CARTESIAN_POINT('Ctrl Pts',(0.00243631232545395,-0.0311786899535083,
-0.0104093370523894));
#38963=CARTESIAN_POINT('Ctrl Pts',(0.00228871161240723,-0.0311912574119168,
-0.0102219657098566));
#38964=CARTESIAN_POINT('Ctrl Pts',(0.00212158344994877,-0.0312038248703253,
-0.0100547960820246));
#38965=CARTESIAN_POINT('Ctrl Pts',(0.00173460996431537,-0.0312329239348657,
-0.00966772658624013));
#38966=CARTESIAN_POINT('Ctrl Pts',(0.00123737539096422,-0.0312620229994061,
-0.00938834989393673));
#38967=CARTESIAN_POINT('Ctrl Pts',(0.000703810673627834,-0.0312911220639464,
-0.00925957988790571));
#38968=CARTESIAN_POINT('Ctrl Pts',(0.000473472123254697,-0.0313036840571324,
-0.00920399019923815));
#38969=CARTESIAN_POINT('Ctrl Pts',(0.000236722135829542,-0.0313162460503184,
-0.00917588864684906));
#38970=CARTESIAN_POINT('Ctrl Pts',(4.48548968202519E-7,-0.0313288080435043,
-0.0091758533200908));
#38971=CARTESIAN_POINT('Ctrl Pts',(-0.000544847326927436,-0.0313577998710222,
-0.00917577178945572));
#38972=CARTESIAN_POINT('Ctrl Pts',(-0.00109214034091453,-0.0313867916985402,
-0.00932869941596481));
#38973=CARTESIAN_POINT('Ctrl Pts',(-0.00155932450626538,-0.0314157835260581,
-0.00961294340047934));
#38974=CARTESIAN_POINT('Ctrl Pts',(-0.00176348078916547,-0.0314284527562665,
-0.00973715607637691));
#38975=CARTESIAN_POINT('Ctrl Pts',(-0.00195249554526538,-0.0314411219864749,
-0.00988576715654636));
#38976=CARTESIAN_POINT('Ctrl Pts',(-0.00212094908975225,-0.0314537912166833,
-0.0100541617541531));
#38977=CARTESIAN_POINT('Ctrl Pts',(-0.00251366863868406,-0.0314833272789129,
-0.0104467438788933));
#38978=CARTESIAN_POINT('Ctrl Pts',(-0.00279529381109297,-0.0315128633411424,
-0.0109523715539673));
#38979=CARTESIAN_POINT('Ctrl Pts',(-0.00292174824045499,-0.031542399403372,
-0.0114951277769743));
#38980=CARTESIAN_POINT('Ctrl Pts',(-0.00297365967586053,-0.0315545243988687,
-0.0117179373278435));
#38981=CARTESIAN_POINT('Ctrl Pts',(-0.00299995411642938,-0.0315666493943655,
-0.0119466777319896));
#38982=CARTESIAN_POINT('Ctrl Pts',(-0.00299999993971496,-0.0315787743898623,
-0.0121752518630578));
#38983=CARTESIAN_POINT('',(-0.00299999948627239,-0.0325786872255947,-0.0121769732930159));
#38984=CARTESIAN_POINT('Ctrl Pts',(-0.00299999999999953,-0.0315788060372049,
-0.0121758516139528));
#38985=CARTESIAN_POINT('Ctrl Pts',(-0.00300000031042998,-0.0316082332034078,
-0.0127326424646223));
#38986=CARTESIAN_POINT('Ctrl Pts',(-0.0028406931286498,-0.031637678669113,
-0.0132895533835456));
#38987=CARTESIAN_POINT('Ctrl Pts',(-0.00254637369723003,-0.0316671428820116,
-0.013762037700192));
#38988=CARTESIAN_POINT('Ctrl Pts',(-0.00242550781667549,-0.031679242722038,
-0.0139560691737654));
#38989=CARTESIAN_POINT('Ctrl Pts',(-0.00228247616791868,-0.0316913457236565,
-0.0141360323583952));
#38990=CARTESIAN_POINT('Ctrl Pts',(-0.00212122458616147,-0.0317034519178721,
-0.0142972693831936));
#38991=CARTESIAN_POINT('Ctrl Pts',(-0.00173579172354728,-0.0317323888438919,
-0.0146826674509222));
#38992=CARTESIAN_POINT('Ctrl Pts',(-0.0012407291534123,-0.0317613440102813,
-0.0149614859389926));
#38993=CARTESIAN_POINT('Ctrl Pts',(-0.000709282271278857,-0.0317903161467925,
-0.0150908007405698));
#38994=CARTESIAN_POINT('Ctrl Pts',(-0.000476972294568734,-0.0318029806605651,
-0.0151473277794003));
#38995=CARTESIAN_POINT('Ctrl Pts',(-0.000238082320351396,-0.0318156484169943,
-0.0151758756826124));
#38996=CARTESIAN_POINT('Ctrl Pts',(2.82038538772012E-7,-0.0318283193099807,
-0.0151758532733005));
#38997=CARTESIAN_POINT('Ctrl Pts',(0.000547626181592029,-0.0318574148471478,
-0.0151758018159195));
#38998=CARTESIAN_POINT('Ctrl Pts',(0.00109676449279499,-0.0318865269226405,
-0.0150216259929139));
#38999=CARTESIAN_POINT('Ctrl Pts',(0.00156506872148099,-0.0319156602466803,
-0.0147352594475732));
#39000=CARTESIAN_POINT('Ctrl Pts',(0.0017672604829583,-0.0319282386470971,
-0.014611619828958));
#39001=CARTESIAN_POINT('Ctrl Pts',(0.00195453948115426,-0.0319408210084698,
-0.01446400220402));
#39002=CARTESIAN_POINT('Ctrl Pts',(0.00212162342931928,-0.0319534077098926,
-0.0142968705010482));
#39003=CARTESIAN_POINT('Ctrl Pts',(0.00250834747015757,-0.03198254025128,
-0.0139100359293539));
#39004=CARTESIAN_POINT('Ctrl Pts',(0.00278749957941142,-0.0320116960429182,
-0.0134130827230974));
#39005=CARTESIAN_POINT('Ctrl Pts',(0.00291622471053343,-0.0320408575633779,
-0.012879865671161));
#39006=CARTESIAN_POINT('Ctrl Pts',(0.00297192875716824,-0.032053476814036,
-0.012649123256928));
#39007=CARTESIAN_POINT('Ctrl Pts',(0.00300004532358358,-0.0320660971374776,
-0.0124119508547963));
#39008=CARTESIAN_POINT('Ctrl Pts',(0.00299999994485587,-0.0320787171138616,
-0.0121752780781099));
#39009=CARTESIAN_POINT('Ctrl Pts',(0.00299989497489855,-0.0321079096110824,
-0.0116278072140276));
#39010=CARTESIAN_POINT('Ctrl Pts',(0.00284559654022781,-0.0321371002512389,
-0.0110785818195714));
#39011=CARTESIAN_POINT('Ctrl Pts',(0.00255908040558366,-0.0321662753031713,
-0.0106102519714853));
#39012=CARTESIAN_POINT('Ctrl Pts',(0.002435506461596,-0.0321788584557321,
-0.0104082620678904));
#39013=CARTESIAN_POINT('Ctrl Pts',(0.00228800007691206,-0.032191438708598,
-0.0102211643532271));
#39014=CARTESIAN_POINT('Ctrl Pts',(0.00212101305761234,-0.0322040149601267,
-0.0100542257015569));
#39015=CARTESIAN_POINT('Ctrl Pts',(0.0017339610656569,-0.0322331649097809,
-0.00966728581883857));
#39016=CARTESIAN_POINT('Ctrl Pts',(0.00123668732942299,-0.0322622933624106,
-0.00938805092606279));
#39017=CARTESIAN_POINT('Ctrl Pts',(0.000703123706334418,-0.0322914039985368,
-0.00925941418148655));
#39018=CARTESIAN_POINT('Ctrl Pts',(0.000472760129879772,-0.0323039723783152,
-0.00920387587403498));
#39019=CARTESIAN_POINT('Ctrl Pts',(0.000235991095858931,-0.0323165374370263,
-0.00917583015568731));
#39020=CARTESIAN_POINT('Ctrl Pts',(-2.93864620455047E-7,-0.0323290994708749,
-0.00917585330095084));
#39021=CARTESIAN_POINT('Ctrl Pts',(-0.000545585330011292,-0.0323580897622235,
-0.0091759067149076));
#39022=CARTESIAN_POINT('Ctrl Pts',(-0.00109283713400837,-0.0323870639437451,
-0.00932896737902686));
#39023=CARTESIAN_POINT('Ctrl Pts',(-0.00155994938770585,-0.0324160210225555,
-0.00961332369496386));
#39024=CARTESIAN_POINT('Ctrl Pts',(-0.0017640600889872,-0.0324286741902176,
-0.00973757684096947));
#39025=CARTESIAN_POINT('Ctrl Pts',(-0.00195302566753906,-0.0324413240923474,
-0.00988622107287341));
#39026=CARTESIAN_POINT('Ctrl Pts',(-0.00212142866450282,-0.0324539706461063,
-0.0100546412694731));
#39027=CARTESIAN_POINT('Ctrl Pts',(-0.0025140641651425,-0.0324834563800662,
-0.0104473168714637));
#39028=CARTESIAN_POINT('Ctrl Pts',(-0.00279557634430618,-0.0325129239122803,
-0.0109530147086656));
#39029=CARTESIAN_POINT('Ctrl Pts',(-0.00292190610715409,-0.0325423735927181,
-0.0114958057139754));
#39030=CARTESIAN_POINT('Ctrl Pts',(-0.00297375926539034,-0.0325544614721324,
-0.011718599038787));
#39031=CARTESIAN_POINT('Ctrl Pts',(-0.00300000058860966,-0.0325665463439438,
-0.0119473157627861));
#39032=CARTESIAN_POINT('Ctrl Pts',(-0.00299999999999005,-0.0325786282323535,
-0.0121758610130754));
#39033=CARTESIAN_POINT('',(-0.00299999999995998,-0.0335788169750034,-0.0121758687814435));
#39034=CARTESIAN_POINT('Ctrl Pts',(-0.00299999872723928,-0.0325787743898623,
-0.012178616719692));
#39035=CARTESIAN_POINT('Ctrl Pts',(-0.0029994858324129,-0.0326083191993918,
-0.0127354182603145));
#39036=CARTESIAN_POINT('Ctrl Pts',(-0.0028396594007697,-0.0326378640089213,
-0.0132921917133723));
#39037=CARTESIAN_POINT('Ctrl Pts',(-0.0025448941804952,-0.0326674088184508,
-0.0137644103708587));
#39038=CARTESIAN_POINT('Ctrl Pts',(-0.0024239557840027,-0.032679530675588,
-0.0139581556409997));
#39039=CARTESIAN_POINT('Ctrl Pts',(-0.00228090445082536,-0.0326916525327251,
-0.01413783744446));
#39040=CARTESIAN_POINT('Ctrl Pts',(-0.00211967908184265,-0.0327037743898623,
-0.0142988136229748));
#39041=CARTESIAN_POINT('Ctrl Pts',(-0.00173396026633068,-0.0327327749646866,
-0.0146839362701995));
#39042=CARTESIAN_POINT('Ctrl Pts',(-0.00123868829186396,-0.0327617755395109,
-0.0149623948905047));
#39043=CARTESIAN_POINT('Ctrl Pts',(-0.000707142468841261,-0.0327907761143351,
-0.0150913205782218));
#39044=CARTESIAN_POINT('Ctrl Pts',(-0.000474988166602747,-0.0328034422061775,
-0.0151476292759412));
#39045=CARTESIAN_POINT('Ctrl Pts',(-0.000236285739616681,-0.0328161082980199,
-0.0151760017068329));
#39046=CARTESIAN_POINT('Ctrl Pts',(1.87696153578847E-6,-0.0328287743898623,
-0.0151758526993939));
#39047=CARTESIAN_POINT('Ctrl Pts',(0.000549196391118819,-0.0328578822145917,
-0.0151755102668212));
#39048=CARTESIAN_POINT('Ctrl Pts',(0.00109822958083191,-0.0328869900393211,
-0.0150210560134721));
#39049=CARTESIAN_POINT('Ctrl Pts',(0.00156636682566337,-0.0329160978640505,
-0.01473446520857));
#39050=CARTESIAN_POINT('Ctrl Pts',(0.00176834899772359,-0.0329286567059878,
-0.0146108129379897));
#39051=CARTESIAN_POINT('Ctrl Pts',(0.00195542767052654,-0.032941215547925,
-0.0144632254267738));
#39052=CARTESIAN_POINT('Ctrl Pts',(0.00212233389845239,-0.0329537743898623,
-0.0142961595907226));
#39053=CARTESIAN_POINT('Ctrl Pts',(0.00250910232189599,-0.0329828767400665,
-0.013909021310601));
#39054=CARTESIAN_POINT('Ctrl Pts',(0.00278815368193294,-0.0330119790902707,
-0.0134117190045828));
#39055=CARTESIAN_POINT('Ctrl Pts',(0.00291663000649855,-0.0330410814404749,
-0.0128781846935109));
#39056=CARTESIAN_POINT('Ctrl Pts',(0.00297209690825918,-0.0330536457569373,
-0.0126478426805509));
#39057=CARTESIAN_POINT('Ctrl Pts',(0.00300007783540791,-0.0330662100733998,
-0.0124111062716708));
#39058=CARTESIAN_POINT('Ctrl Pts',(0.00299999983648833,-0.0330787743898623,
-0.0121748627967843));
#39059=CARTESIAN_POINT('Ctrl Pts',(0.00299981916992521,-0.0331078767400665,
-0.0116276591060678));
#39060=CARTESIAN_POINT('Ctrl Pts',(0.00284559023185504,-0.0331369790902707,
-0.0110786774696764));
#39061=CARTESIAN_POINT('Ctrl Pts',(0.00255923810211162,-0.0331660814404748,
-0.0106105097662086));
#39062=CARTESIAN_POINT('Ctrl Pts',(0.00243561170243732,-0.0331786457569373,
-0.0104083883862302));
#39063=CARTESIAN_POINT('Ctrl Pts',(0.00228802265505789,-0.0331912100733998,
-0.0102211743760228));
#39064=CARTESIAN_POINT('Ctrl Pts',(0.00212093334135249,-0.0332037743898623,
-0.010054146011381));
#39065=CARTESIAN_POINT('Ctrl Pts',(0.00173383656040047,-0.0332328822145917,
-0.00966719043147765));
#39066=CARTESIAN_POINT('Ctrl Pts',(0.0012365101137741,-0.0332619900393211,
-0.00938796491070863));
#39067=CARTESIAN_POINT('Ctrl Pts',(0.000702900046714844,-0.0332910978640505,
-0.00925936026850915));
#39068=CARTESIAN_POINT('Ctrl Pts',(0.000472669016033597,-0.0333036567059878,
-0.00920387259848232));
#39069=CARTESIAN_POINT('Ctrl Pts',(0.000236042090910841,-0.033316215547925,
-0.00917584510055194));
#39070=CARTESIAN_POINT('Ctrl Pts',(-1.04017925362034E-7,-0.0333287743898623,
-0.00917585328836139));
#39071=CARTESIAN_POINT('Ctrl Pts',(-0.000545406915514975,-0.0333577749646866,
-0.00917587219545343));
#39072=CARTESIAN_POINT('Ctrl Pts',(-0.00109267735081907,-0.0333867755395109,
-0.00932890439108765));
#39073=CARTESIAN_POINT('Ctrl Pts',(-0.00155981219574908,-0.0334157761143351,
-0.00961324018388489));
#39074=CARTESIAN_POINT('Ctrl Pts',(-0.0017638348016634,-0.0334284422061775,
-0.00973742473151781));
#39075=CARTESIAN_POINT('Ctrl Pts',(-0.00195272767242404,-0.0334411082980199,
-0.00988597836688022));
#39076=CARTESIAN_POINT('Ctrl Pts',(-0.00212108046664552,-0.0334537743898623,
-0.0100542930932063));
#39077=CARTESIAN_POINT('Ctrl Pts',(-0.00251377864860435,-0.0334833191993918,
-0.010446902478342));
#39078=CARTESIAN_POINT('Ctrl Pts',(-0.00279537308278998,-0.0335128640089212,
-0.0109525513711848));
#39079=CARTESIAN_POINT('Ctrl Pts',(-0.00292179270627805,-0.0335424088184507,
-0.0114953186573581));
#39080=CARTESIAN_POINT('Ctrl Pts',(-0.00297366105945631,-0.0335545306755879,
-0.0117180091267337));
#39081=CARTESIAN_POINT('Ctrl Pts',(-0.00299994031444842,-0.0335666525327251,
-0.0119466221991571));
#39082=CARTESIAN_POINT('Ctrl Pts',(-0.00299999989796097,-0.0335787743898623,
-0.0121750708326259));
#39083=CARTESIAN_POINT('',(0.00299999097150563,-0.0340787743898654,-0.0121736669288307));
#39084=CARTESIAN_POINT('Ctrl Pts',(-0.00299999999995998,-0.0335788169750034,
-0.0121758687814435));
#39085=CARTESIAN_POINT('Ctrl Pts',(-0.00299999712337882,-0.0336083693720943,
-0.0127328102029425));
#39086=CARTESIAN_POINT('Ctrl Pts',(-0.00284060331293545,-0.0336379217691852,
-0.013289857790904));
#39087=CARTESIAN_POINT('Ctrl Pts',(-0.00254613224254524,-0.0336674741662761,
-0.0137624252526131));
#39088=CARTESIAN_POINT('Ctrl Pts',(-0.00242545651832797,-0.0336795848870901,
-0.013956085772839));
#39089=CARTESIAN_POINT('Ctrl Pts',(-0.00228269685520116,-0.0336916956079041,
-0.014135728072455));
#39090=CARTESIAN_POINT('Ctrl Pts',(-0.00212177464786208,-0.0337038063287181,
-0.0142967192285002));
#39091=CARTESIAN_POINT('Ctrl Pts',(-0.0017363337691742,-0.033732813927789,
-0.0146823252531321));
#39092=CARTESIAN_POINT('Ctrl Pts',(-0.00124119544968554,-0.0337618215268599,
-0.0149613032246193));
#39093=CARTESIAN_POINT('Ctrl Pts',(-0.000709640673447739,-0.0337908291259308,
-0.0150907135086937));
#39094=CARTESIAN_POINT('Ctrl Pts',(-0.000477732425352501,-0.0338034846447648,
-0.0151471729999951));
#39095=CARTESIAN_POINT('Ctrl Pts',(-0.000239263314320967,-0.0338161401635988,
-0.015175749839925));
#39096=CARTESIAN_POINT('Ctrl Pts',(-1.30059909074996E-6,-0.0338287956824328,
-0.0151758530046318));
#39097=CARTESIAN_POINT('Ctrl Pts',(0.000544131565940404,-0.0338578032815037,
-0.0151760894675133));
#39098=CARTESIAN_POINT('Ctrl Pts',(0.00109159196088156,-0.0338868108805747,
-0.0150232433455221));
#39099=CARTESIAN_POINT('Ctrl Pts',(0.00155893455235758,-0.0339158184796456,
-0.0147390003875778));
#39100=CARTESIAN_POINT('Ctrl Pts',(0.00176282812362129,-0.0339284739984796,
-0.0146149900515654));
#39101=CARTESIAN_POINT('Ctrl Pts',(0.00195162785719649,-0.0339411295173136,
-0.0144666455862975));
#39102=CARTESIAN_POINT('Ctrl Pts',(0.00211993491957889,-0.0339537850361476,
-0.0142985581498752));
#39103=CARTESIAN_POINT('Ctrl Pts',(0.00251295532482384,-0.0339833374332385,
-0.013906050601801));
#39104=CARTESIAN_POINT('Ctrl Pts',(0.00279485478800578,-0.0340128898303293,
-0.0134003999633648));
#39105=CARTESIAN_POINT('Ctrl Pts',(0.00292152123044294,-0.0340424422274202,
-0.0128575524137918));
#39106=CARTESIAN_POINT('Ctrl Pts',(0.00297342977498999,-0.0340545529482342,
-0.012635090760436));
#39107=CARTESIAN_POINT('Ctrl Pts',(0.00299979978310408,-0.0340666636690483,
-0.0124067072854433));
#39108=CARTESIAN_POINT('Ctrl Pts',(0.00299999885881957,-0.0340787743898623,
-0.0121784699793747));
#39109=CARTESIAN_POINT('',(0.00212132034355965,-0.0340787743898723,-0.0142971736301177));
#39110=CARTESIAN_POINT('Origin',(0.,-0.0340787743898623,-0.0121758532865581));
#39111=CARTESIAN_POINT('',(-0.00299989950608398,-0.0337035851790747,-0.0121776595950485));
#39112=CARTESIAN_POINT('Ctrl Pts',(0.00212132034355965,-0.0340787743898623,
-0.0142971736301177));
#39113=CARTESIAN_POINT('Ctrl Pts',(0.0017049242015075,-0.0340475243898623,
-0.0147135697721699));
#39114=CARTESIAN_POINT('Ctrl Pts',(0.000620767042151375,-0.0339850243898623,
-0.0152929740109833));
#39115=CARTESIAN_POINT('Ctrl Pts',(-0.00121534600412802,-0.0338912743898623,
-0.0151128743279742));
#39116=CARTESIAN_POINT('Ctrl Pts',(-0.00264184561203855,-0.0337975243898623,
-0.0139428974550539));
#39117=CARTESIAN_POINT('Ctrl Pts',(-0.00299958575104565,-0.0337350243898623,
-0.012766832826268));
#39118=CARTESIAN_POINT('Ctrl Pts',(-0.00299999926036318,-0.0337037743898623,
-0.0121779599000421));
#39119=CARTESIAN_POINT('',(-0.00299999923775439,-0.0327037743898623,-0.0121737147185652));
#39120=CARTESIAN_POINT('Ctrl Pts',(-0.00299932366121755,-0.0337024929345961,
-0.0121759260444648));
#39121=CARTESIAN_POINT('Ctrl Pts',(-0.00299712296400654,-0.0336720038405544,
-0.0116201236474055));
#39122=CARTESIAN_POINT('Ctrl Pts',(-0.00284134996265265,-0.0336450671877836,
-0.0110636879727134));
#39123=CARTESIAN_POINT('Ctrl Pts',(-0.00254831752635056,-0.0336169910244305,
-0.0105910159029857));
#39124=CARTESIAN_POINT('Ctrl Pts',(-0.00250350847321846,-0.0336126977580901,
-0.0105187372564517));
#39125=CARTESIAN_POINT('Ctrl Pts',(-0.00245567366869795,-0.0336082649481663,
-0.0104483703245496));
#39126=CARTESIAN_POINT('Ctrl Pts',(-0.00240484794115916,-0.033603720390553,
-0.0103802875159579));
#39127=CARTESIAN_POINT('Ctrl Pts',(-0.00231856073827001,-0.0335960050624345,
-0.0102647028425515));
#39128=CARTESIAN_POINT('Ctrl Pts',(-0.00222364272152698,-0.0335879676540423,
-0.0101557057813394));
#39129=CARTESIAN_POINT('Ctrl Pts',(-0.00212163897555336,-0.033579744174801,
-0.0100541729698885));
#39130=CARTESIAN_POINT('Ctrl Pts',(-0.00173486111027858,-0.0335485623812726,
-0.00966918079441987));
#39131=CARTESIAN_POINT('Ctrl Pts',(-0.00123883616658502,-0.0335185292847313,
-0.00939260545203301));
#39132=CARTESIAN_POINT('Ctrl Pts',(-0.000707074316813727,-0.0334910935177513,
-0.00926138600833388));
#39133=CARTESIAN_POINT('Ctrl Pts',(-0.000475778990634066,-0.0334791600466394,
-0.00920431075172313));
#39134=CARTESIAN_POINT('Ctrl Pts',(-0.000237646442315334,-0.033467829772317,
-0.00917515682429721));
#39135=CARTESIAN_POINT('Ctrl Pts',(7.38310283306005E-8,-0.0334557455696987,
-0.00917485485860858));
#39136=CARTESIAN_POINT('Ctrl Pts',(6.96966992447012E-5,-0.033452206381246,
-0.00917476641971757));
#39137=CARTESIAN_POINT('Ctrl Pts',(0.000139279753693056,-0.0334485633437618,
-0.00917707797200307));
#39138=CARTESIAN_POINT('Ctrl Pts',(0.000208683016430185,-0.0334448399147507,
-0.00918190242644719));
#39139=CARTESIAN_POINT('Ctrl Pts',(0.000689586586317118,-0.0334190398264973,
-0.00921533165258783));
#39140=CARTESIAN_POINT('Ctrl Pts',(0.00116359922847722,-0.0333893799231094,
-0.00937025399267345));
#39141=CARTESIAN_POINT('Ctrl Pts',(0.00157475316846205,-0.0333636641845656,
-0.00962402027786571));
#39142=CARTESIAN_POINT('Ctrl Pts',(0.00177265356168317,-0.0333512864489418,
-0.00974616539856592));
#39143=CARTESIAN_POINT('Ctrl Pts',(0.00195640797895683,-0.0333396246142925,
-0.00989103223327693));
#39144=CARTESIAN_POINT('Ctrl Pts',(0.00212100455005177,-0.033328264314852,
-0.0100547923352072));
#39145=CARTESIAN_POINT('Ctrl Pts',(0.00232121948316958,-0.0333144456698003,
-0.0102539897889405));
#39146=CARTESIAN_POINT('Ctrl Pts',(0.00249575585499712,-0.0333000788700998,
-0.0104821170588777));
#39147=CARTESIAN_POINT('Ctrl Pts',(0.00263223344424879,-0.0332850382196607,
-0.010731087603101));
#39148=CARTESIAN_POINT('Ctrl Pts',(0.002746503265138,-0.0332724449987432,
-0.0109395454140213));
#39149=CARTESIAN_POINT('Ctrl Pts',(0.00283411747476242,-0.0332593793841039,
-0.011162518444991));
#39150=CARTESIAN_POINT('Ctrl Pts',(0.00289549840934342,-0.033245767596808,
-0.0113913522361136));
#39151=CARTESIAN_POINT('Ctrl Pts',(0.0029643578013657,-0.0332304973927303,
-0.0116480664070271));
#39152=CARTESIAN_POINT('Ctrl Pts',(0.00299871148338599,-0.0332155634345403,
-0.0119129046483332));
#39153=CARTESIAN_POINT('Ctrl Pts',(0.00299877890744598,-0.0332016648463028,
-0.0121757419432914));
#39154=CARTESIAN_POINT('Ctrl Pts',(0.00299890693696643,-0.0331752732349504,
-0.0126748357806571));
#39155=CARTESIAN_POINT('Ctrl Pts',(0.0028748961594508,-0.033152653571698,
-0.013172493157235));
#39156=CARTESIAN_POINT('Ctrl Pts',(0.00263826635774537,-0.033126523774227,
-0.0136074814841024));
#39157=CARTESIAN_POINT('Ctrl Pts',(0.00258279739963268,-0.0331203986258689,
-0.0137094481388036));
#39158=CARTESIAN_POINT('Ctrl Pts',(0.00252110363446337,-0.0331140805985485,
-0.0138080698342926));
#39159=CARTESIAN_POINT('Ctrl Pts',(0.00245391928001071,-0.0331074758934644,
-0.0139030936547182));
#39160=CARTESIAN_POINT('Ctrl Pts',(0.00236154049408779,-0.0330983943946241,
-0.0140337518300656));
#39161=CARTESIAN_POINT('Ctrl Pts',(0.00225854225119812,-0.0330891010895125,
-0.0141570197667402));
#39162=CARTESIAN_POINT('Ctrl Pts',(0.00214609493720693,-0.0330800644838706,
-0.0142713277699323));
#39163=CARTESIAN_POINT('Ctrl Pts',(0.00176980594943767,-0.0330498247647598,
-0.0146538432902091));
#39164=CARTESIAN_POINT('Ctrl Pts',(0.00128664527240643,-0.0330218468616416,
-0.0149389591782877));
#39165=CARTESIAN_POINT('Ctrl Pts',(0.000761545417184402,-0.0329953331669265,
-0.0150781148955854));
#39166=CARTESIAN_POINT('Ctrl Pts',(0.000585478026924089,-0.0329864430539542,
-0.0151247741809399));
#39167=CARTESIAN_POINT('Ctrl Pts',(0.000404957692717902,-0.0329773611900798,
-0.0151554473731775));
#39168=CARTESIAN_POINT('Ctrl Pts',(0.000223331473602049,-0.0329676888854435,
-0.0151689182329267));
#39169=CARTESIAN_POINT('Ctrl Pts',(0.000164832159414799,-0.032964573568775,
-0.0151732570121));
#39170=CARTESIAN_POINT('Ctrl Pts',(0.000106214754925876,-0.0329613970000329,
-0.0151758161624007));
#39171=CARTESIAN_POINT('Ctrl Pts',(4.75877733928088E-5,-0.032958145857755,
-0.01517667014769));
#39172=CARTESIAN_POINT('Ctrl Pts',(-0.000493648198624367,-0.0329281317737125,
-0.0151845540186668));
#39173=CARTESIAN_POINT('Ctrl Pts',(-0.00103971989257228,-0.0328963193462496,
-0.0150392486864561));
#39174=CARTESIAN_POINT('Ctrl Pts',(-0.00151253595850431,-0.0328681306236198,
-0.0147650753466467));
#39175=CARTESIAN_POINT('Ctrl Pts',(-0.00172418321353248,-0.0328555124699714,
-0.0146423467869516));
#39176=CARTESIAN_POINT('Ctrl Pts',(-0.00192091540781267,-0.0328438008855719,
-0.0144933772495667));
#39177=CARTESIAN_POINT('Ctrl Pts',(-0.00209642903093382,-0.0328317779866714,
-0.0143227737760233));
#39178=CARTESIAN_POINT('Ctrl Pts',(-0.00220478715253754,-0.032824355322163,
-0.0142174470691643));
#39179=CARTESIAN_POINT('Ctrl Pts',(-0.00230563731691904,-0.0328164509163901,
-0.0141041753377086));
#39180=CARTESIAN_POINT('Ctrl Pts',(-0.00239698774693834,-0.0328082565659287,
-0.013983366227865));
#39181=CARTESIAN_POINT('Ctrl Pts',(-0.00263994304948872,-0.0327864628984535,
-0.0136620627175618));
#39182=CARTESIAN_POINT('Ctrl Pts',(-0.00281552462457732,-0.0327626183203804,
-0.0132865952314827));
#39183=CARTESIAN_POINT('Ctrl Pts',(-0.00291196287183983,-0.0327403310118172,
-0.0128924370499046));
#39184=CARTESIAN_POINT('Ctrl Pts',(-0.00296920402740611,-0.0327271023257634,
-0.0126584835052284));
#39185=CARTESIAN_POINT('Ctrl Pts',(-0.00299873369263853,-0.0327144851464306,
-0.0124173715237727));
#39186=CARTESIAN_POINT('Ctrl Pts',(-0.00299918122624294,-0.0327024705208686,
-0.0121759162920882));
#39187=CARTESIAN_POINT('Ctrl Pts',(-0.00299999923775439,-0.0327037743898623,
-0.0121737147185652));
#39188=CARTESIAN_POINT('Ctrl Pts',(-0.002999602319356,-0.0326742337072068,
-0.0116169146090542));
#39189=CARTESIAN_POINT('Ctrl Pts',(-0.002839892690886,-0.0326446930245512,
-0.0110601091576252));
#39190=CARTESIAN_POINT('Ctrl Pts',(-0.00254522722774817,-0.0326151523418957,
-0.0105878298739066));
#39191=CARTESIAN_POINT('Ctrl Pts',(-0.00242429803692082,-0.0326030289976395,
-0.0103940088844481));
#39192=CARTESIAN_POINT('Ctrl Pts',(-0.00228124142308449,-0.0325909056533834,
-0.0102142540931621));
#39193=CARTESIAN_POINT('Ctrl Pts',(-0.0021199985543597,-0.0325787823091272,
-0.0100532119768892));
#39194=CARTESIAN_POINT('Ctrl Pts',(-0.00173434008204576,-0.032549785861333,
-0.00966803366152436));
#39195=CARTESIAN_POINT('Ctrl Pts',(-0.00123911318528987,-0.0325207894135388,
-0.00938950111789259));
#39196=CARTESIAN_POINT('Ctrl Pts',(-0.000707589724350954,-0.0324917929657446,
-0.00926049451241161));
#39197=CARTESIAN_POINT('Ctrl Pts',(-0.000475384885260714,-0.0324791253866271,
-0.00920413583726607));
#39198=CARTESIAN_POINT('Ctrl Pts',(-0.00023662427972223,-0.0324664578075097,
-0.0091757267513867));
#39199=CARTESIAN_POINT('Ctrl Pts',(1.59885239224121E-6,-0.0324537902283922,
-0.00917585371261296));
#39200=CARTESIAN_POINT('Ctrl Pts',(0.000548915156033654,-0.0324246865367518,
-0.00917614540531485));
#39201=CARTESIAN_POINT('Ctrl Pts',(0.00109796015032326,-0.0323955828451114,
-0.00933054705960091));
#39202=CARTESIAN_POINT('Ctrl Pts',(0.00156612260844863,-0.032366479153471,
-0.00961709187225897));
#39203=CARTESIAN_POINT('Ctrl Pts',(0.00176816836635975,-0.0323539188181997,
-0.0097407565592585));
#39204=CARTESIAN_POINT('Ctrl Pts',(0.00195530521981268,-0.0323413584829284,
-0.00988837024876112));
#39205=CARTESIAN_POINT('Ctrl Pts',(0.00212225987648144,-0.0323287981476571,
-0.0100554728922239));
#39206=CARTESIAN_POINT('Ctrl Pts',(0.00250903964605414,-0.0322996999261464,
-0.0104425954991826));
#39207=CARTESIAN_POINT('Ctrl Pts',(0.00278810780862761,-0.0322706017046357,
-0.0109398851664139));
#39208=CARTESIAN_POINT('Ctrl Pts',(0.00291660361119665,-0.032241503483125,
-0.0114734122746897));
#39209=CARTESIAN_POINT('Ctrl Pts',(0.0029720933685116,-0.032228937677724,
-0.0117038111606243));
#39210=CARTESIAN_POINT('Ctrl Pts',(0.00300008323900718,-0.032216371872323,
-0.011940608760253));
#39211=CARTESIAN_POINT('Ctrl Pts',(0.00299999981303822,-0.032203806066922,
-0.0121769124232979));
#39212=CARTESIAN_POINT('Ctrl Pts',(0.00299980662627087,-0.0321747078454113,
-0.0127241130293597));
#39213=CARTESIAN_POINT('Ctrl Pts',(0.00284556678595463,-0.0321456096239006,
-0.0132730886889762));
#39214=CARTESIAN_POINT('Ctrl Pts',(0.00255920646923548,-0.0321165114023899,
-0.0137412485234945));
#39215=CARTESIAN_POINT('Ctrl Pts',(0.00243554434049904,-0.032103945596989,
-0.0139434191398311));
#39216=CARTESIAN_POINT('Ctrl Pts',(0.00228790753192101,-0.032091379791588,
-0.0141306742213337));
#39217=CARTESIAN_POINT('Ctrl Pts',(0.00212076216568075,-0.032078813986187,
-0.0142977316611633));
#39218=CARTESIAN_POINT('Ctrl Pts',(0.00173363638719356,-0.0320497102945466,
-0.0146846537930824));
#39219=CARTESIAN_POINT('Ctrl Pts',(0.00123629038411274,-0.0320206066029062,
-0.0149638386139045));
#39220=CARTESIAN_POINT('Ctrl Pts',(0.000702672738198018,-0.0319915029112658,
-0.0150924010785535));
#39221=CARTESIAN_POINT('Ctrl Pts',(0.00047237836103825,-0.0319789425759945,
-0.0151478850246882));
#39222=CARTESIAN_POINT('Ctrl Pts',(0.000235686941747564,-0.0319663822407232,
-0.0151758941384449));
#39223=CARTESIAN_POINT('Ctrl Pts',(-5.19421053127542E-7,-0.0319538219054519,
-0.0151758532415917));
#39224=CARTESIAN_POINT('Ctrl Pts',(-0.00054581899464477,-0.0319248254576577,
-0.0151757588282307));
#39225=CARTESIAN_POINT('Ctrl Pts',(-0.00109306558886062,-0.0318958290098635,
-0.0150226526353755));
#39226=CARTESIAN_POINT('Ctrl Pts',(-0.00156015962044416,-0.0318668325620693,
-0.0147382548863733));
#39227=CARTESIAN_POINT('Ctrl Pts',(-0.00176421739477506,-0.0318541649829518,
-0.0146140110130586));
#39228=CARTESIAN_POINT('Ctrl Pts',(-0.00195313436141152,-0.0318414974038343,
-0.0144653876112966));
#39229=CARTESIAN_POINT('Ctrl Pts',(-0.00212149680405239,-0.0318288298247168,
-0.014296997154945));
#39230=CARTESIAN_POINT('Ctrl Pts',(-0.00251411653376062,-0.0317992891420613,
-0.0139043120975107));
#39231=CARTESIAN_POINT('Ctrl Pts',(-0.00279561145356866,-0.0317697484594058,
-0.0133986097351527));
#39232=CARTESIAN_POINT('Ctrl Pts',(-0.00292192511681729,-0.0317402077767503,
-0.0128558191766675));
#39233=CARTESIAN_POINT('Ctrl Pts',(-0.00297376359467769,-0.0317280844324941,
-0.0126330607226316));
#39234=CARTESIAN_POINT('Ctrl Pts',(-0.00299999845410164,-0.031715961088238,
-0.0124043815409992));
#39235=CARTESIAN_POINT('Ctrl Pts',(-0.00299999999993135,-0.0317038377439818,
-0.0121758735812085));
#39236=CARTESIAN_POINT('Origin',(0.,-0.0341787743898723,-0.0121758532865581));
#39237=CARTESIAN_POINT('',(0.000999999999999998,-0.0340787743898723,-0.0121758532865581));
#39238=CARTESIAN_POINT('Origin',(0.,-0.0340787743898623,-0.0121758532865581));
#39239=CARTESIAN_POINT('',(0.001200000000005,-0.0342787743898773,-0.0121758532865581));
#39240=CARTESIAN_POINT('',(0.0011,-0.0341787743898723,-0.0121758532865581));
#39241=CARTESIAN_POINT('Origin',(0.,-0.0342787743898723,-0.0121758532865581));
#39242=CARTESIAN_POINT('Origin',(0.,-0.0121787743898723,-0.0121758532865581));
#39243=CARTESIAN_POINT('',(0.001,-0.0181787743898623,-0.0121758532865581));
#39244=CARTESIAN_POINT('Origin',(0.,-0.0181787743898623,-0.0121758532865581));
#39245=CARTESIAN_POINT('',(0.001,-0.0121787743898723,-0.0121758532865581));
#39246=CARTESIAN_POINT('Origin',(0.,-0.0342787743898723,-0.0121758532865581));
#39247=CARTESIAN_POINT('',(-0.002800000000005,-0.0342787743898673,-0.0121758532865581));
#39248=CARTESIAN_POINT('Origin',(0.,-0.0342787743898723,-0.0121758532865581));
#39249=CARTESIAN_POINT('Origin',(0.,-0.0122787743898723,-0.0121758532865581));
#39250=CARTESIAN_POINT('',(0.00210000000001,-0.0123787743898623,-0.0121758532865581));
#39251=CARTESIAN_POINT('Origin',(0.,-0.0123787743898623,-0.0121758532865581));
#39252=CARTESIAN_POINT('',(0.00230000000001,-0.0121787743898623,-0.0121758532865581));
#39253=CARTESIAN_POINT('',(0.0022,-0.0122787743898723,-0.0121758532865581));
#39254=CARTESIAN_POINT('Origin',(0.,-0.0121787743898623,-0.0121758532865581));
#39255=CARTESIAN_POINT('Origin',(0.,-0.0121787743898723,-0.0121758532865581));
#39256=CARTESIAN_POINT('',(0.00255,-0.0121787743898723,-0.0121758532865581));
#39257=CARTESIAN_POINT('Origin',(0.,-0.0121787743898623,-0.0121758532865581));
#39258=CARTESIAN_POINT('Origin',(0.,-0.0121787743898723,-0.0121758532865581));
#39259=CARTESIAN_POINT('',(0.0021,-0.0171787743898623,-0.0121758532865581));
#39260=CARTESIAN_POINT('',(0.0021,-0.0121787743898723,-0.0121758532865581));
#39261=CARTESIAN_POINT('Origin',(0.,-0.0171787743898623,-0.0121758532865581));
#39262=CARTESIAN_POINT('Origin',(0.,-0.0176787743898723,-0.0121758532865581));
#39263=CARTESIAN_POINT('',(0.00155,-0.0176787743898723,-0.0121758532865581));
#39264=CARTESIAN_POINT('Origin',(0.,-0.0122787743898723,-0.0121758532865581));
#39265=CARTESIAN_POINT('',(0.00275,-0.0123787743898723,-0.0121758532865581));
#39266=CARTESIAN_POINT('Origin',(0.,-0.0123787743898623,-0.0121758532865581));
#39267=CARTESIAN_POINT('',(0.00265,-0.0122787743898723,-0.0121758532865581));
#39268=CARTESIAN_POINT('Origin',(0.,-0.0171787743898723,-0.0121758532865581));
#39269=CARTESIAN_POINT('',(0.00275,-0.0171787743898623,-0.0121758532865581));
#39270=CARTESIAN_POINT('',(0.00275,-0.0171787743898723,-0.0121758532865581));
#39271=CARTESIAN_POINT('Origin',(0.,-0.0171787743898623,-0.0121758532865581));
#39272=CARTESIAN_POINT('Origin',(-3.47714923605922E-19,-0.0173787743898723,
-0.0121758532865581));
#39273=CARTESIAN_POINT('',(-0.00268069430974081,-0.0173787743898623,-0.0135226561740599));
#39274=CARTESIAN_POINT('',(0.00300000000001,-0.0173787743898623,-0.0121758532865581));
#39275=CARTESIAN_POINT('Origin',(0.,-0.0173787743898623,-0.0121758532865581));
#39276=CARTESIAN_POINT('Ctrl Pts',(-0.0026806943097408,-0.017378774389871,
-0.0135226561740599));
#39277=CARTESIAN_POINT('Ctrl Pts',(-0.00271392633795641,-0.0173787741749263,
-0.0134352550519111));
#39278=CARTESIAN_POINT('Ctrl Pts',(-0.00274298533440864,-0.0173787743898643,
-0.0133463390881159));
#39279=CARTESIAN_POINT('Ctrl Pts',(-0.00276788023433509,-0.0173787743898644,
-0.0132562475799165));
#39280=CARTESIAN_POINT('Ctrl Pts',(-0.00282788362768599,-0.0173787743898647,
-0.0130391028546903));
#39281=CARTESIAN_POINT('Ctrl Pts',(-0.00286378472390475,-0.0173787743898649,
-0.0128151065976874));
#39282=CARTESIAN_POINT('Ctrl Pts',(-0.00287475302218889,-0.0173787743898652,
-0.0125890170413387));
#39283=CARTESIAN_POINT('Ctrl Pts',(-0.00287554103043115,-0.0173787743898652,
-0.0125727738257299));
#39284=CARTESIAN_POINT('Ctrl Pts',(-0.00287619933294147,-0.0173787743898653,
-0.0125565288873291));
#39285=CARTESIAN_POINT('Ctrl Pts',(-0.00287672773145678,-0.0173787743898653,
-0.0125402876026397));
#39286=CARTESIAN_POINT('Ctrl Pts',(-0.00287991617497516,-0.0173787743898654,
-0.0124422850205016));
#39287=CARTESIAN_POINT('Ctrl Pts',(-0.00287838091164588,-0.0173787743898657,
-0.0123443722698902));
#39288=CARTESIAN_POINT('Ctrl Pts',(-0.00287208727180318,-0.0173787743898654,
-0.0122469392994813));
#39289=CARTESIAN_POINT('Ctrl Pts',(-0.00285958163282609,-0.0173787743898649,
-0.0120533372531536));
#39290=CARTESIAN_POINT('Ctrl Pts',(-0.00282833650432931,-0.0173787743898647,
-0.0118615973081069));
#39291=CARTESIAN_POINT('Ctrl Pts',(-0.00277748993655705,-0.0173787743898645,
-0.0116750173394792));
#39292=CARTESIAN_POINT('Ctrl Pts',(-0.00277235536708658,-0.0173787743898644,
-0.0116561761894727));
#39293=CARTESIAN_POINT('Ctrl Pts',(-0.0027670189588198,-0.0173787743898644,
-0.0116373840454527));
#39294=CARTESIAN_POINT('Ctrl Pts',(-0.00276148764352656,-0.0173787743898644,
-0.0116186713947204));
#39295=CARTESIAN_POINT('Ctrl Pts',(-0.00272061920221593,-0.0173787743898642,
-0.0114804118980766));
#39296=CARTESIAN_POINT('Ctrl Pts',(-0.00266906423161114,-0.0173787743898641,
-0.0113462105835281));
#39297=CARTESIAN_POINT('Ctrl Pts',(-0.00260657226363377,-0.017378774389864,
-0.0112173959288558));
#39298=CARTESIAN_POINT('Ctrl Pts',(-0.00252329114560864,-0.0173787743898639,
-0.0110457286121373));
#39299=CARTESIAN_POINT('Ctrl Pts',(-0.00242059060388749,-0.0173787743898637,
-0.0108835928969429));
#39300=CARTESIAN_POINT('Ctrl Pts',(-0.00230096382390033,-0.0173787743898637,
-0.0107331618622516));
#39301=CARTESIAN_POINT('Ctrl Pts',(-0.00228846353348929,-0.0173787743898637,
-0.0107174427095612));
#39302=CARTESIAN_POINT('Ctrl Pts',(-0.00227577417957042,-0.0173787743898637,
-0.0107018475972849));
#39303=CARTESIAN_POINT('Ctrl Pts',(-0.00226291969158275,-0.0173787743898637,
-0.0106864045911225));
#39304=CARTESIAN_POINT('Ctrl Pts',(-0.0020869743162019,-0.0173787743898636,
-0.0104750289596036));
#39305=CARTESIAN_POINT('Ctrl Pts',(-0.0018796914814688,-0.0173787743898636,
-0.0102910931413629));
#39306=CARTESIAN_POINT('Ctrl Pts',(-0.00164888534756171,-0.0173787743898638,
-0.0101410525216628));
#39307=CARTESIAN_POINT('Ctrl Pts',(-0.00160588295044858,-0.0173787743898638,
-0.010113097864643));
#39308=CARTESIAN_POINT('Ctrl Pts',(-0.00156205963042595,-0.0173787743898638,
-0.010086330500961));
#39309=CARTESIAN_POINT('Ctrl Pts',(-0.00151746195886052,-0.0173787743898638,
-0.0100608079878154));
#39310=CARTESIAN_POINT('Ctrl Pts',(-0.00150248206522892,-0.0173787743898638,
-0.0100522352413308));
#39311=CARTESIAN_POINT('Ctrl Pts',(-0.00148741201804428,-0.0173787743898639,
-0.0100438015756368));
#39312=CARTESIAN_POINT('Ctrl Pts',(-0.00147227556935763,-0.0173787743898639,
-0.0100355210027254));
#39313=CARTESIAN_POINT('Ctrl Pts',(-0.00119042933630068,-0.0173787743898641,
-0.00988133369426643));
#39314=CARTESIAN_POINT('Ctrl Pts',(-0.000884129244039172,-0.0173787743898644,
-0.009778575357405));
#39315=CARTESIAN_POINT('Ctrl Pts',(-0.000565648716062966,-0.0173787743898649,
-0.0097406856270151));
#39316=CARTESIAN_POINT('Ctrl Pts',(0.00249547098945156,-0.017378774389874,
-0.0123517024776432));
#39317=CARTESIAN_POINT('Ctrl Pts',(0.0025025789150578,-0.0173787743898744,
-0.0125930835426984));
#39318=CARTESIAN_POINT('Ctrl Pts',(0.0024739241321343,-0.0173787743898748,
-0.0128349355184667));
#39319=CARTESIAN_POINT('Ctrl Pts',(0.00241344648103719,-0.0173787743898751,
-0.0130700286939032));
#39320=CARTESIAN_POINT('Ctrl Pts',(0.00240775502746633,-0.0173787743898751,
-0.0130921529310148));
#39321=CARTESIAN_POINT('Ctrl Pts',(0.00240177958578699,-0.0173787743898751,
-0.0131142177455514));
#39322=CARTESIAN_POINT('Ctrl Pts',(0.00239552211903118,-0.0173787743898751,
-0.0131362172550705));
#39323=CARTESIAN_POINT('Ctrl Pts',(0.0023872874601568,-0.0173787743898752,
-0.0131651680211493));
#39324=CARTESIAN_POINT('Ctrl Pts',(0.00237856046135632,-0.0173787743898752,
-0.0131940169394221));
#39325=CARTESIAN_POINT('Ctrl Pts',(0.00236936612861886,-0.0173787743898752,
-0.0132226879746876));
#39326=CARTESIAN_POINT('Ctrl Pts',(0.00228485698784404,-0.0173787743898755,
-0.0134862160223009));
#39327=CARTESIAN_POINT('Ctrl Pts',(0.00216102083655063,-0.0173787743898758,
-0.013735547013867));
#39328=CARTESIAN_POINT('Ctrl Pts',(0.00200195343303136,-0.0173787743898758,
-0.0139605028246134));
#39329=CARTESIAN_POINT('Ctrl Pts',(0.00199374263882198,-0.0173787743898758,
-0.01397211466857));
#39330=CARTESIAN_POINT('Ctrl Pts',(0.00198544255492749,-0.0173787743898758,
-0.0139836535663112));
#39331=CARTESIAN_POINT('Ctrl Pts',(0.00197705447952352,-0.0173787743898758,
-0.0139951174266605));
#39332=CARTESIAN_POINT('Ctrl Pts',(0.00189574251367433,-0.0173787743898759,
-0.0141062453047889));
#39333=CARTESIAN_POINT('Ctrl Pts',(0.00180616371909361,-0.0173787743898759,
-0.0142103508031204));
#39334=CARTESIAN_POINT('Ctrl Pts',(0.00170885054614273,-0.0173787743898759,
-0.0143062456970463));
#39335=CARTESIAN_POINT('Ctrl Pts',(0.00157900085243143,-0.0173787743898759,
-0.014434202912161));
#39336=CARTESIAN_POINT('Ctrl Pts',(0.00143540122347535,-0.0173787743898759,
-0.01454757649909));
#39337=CARTESIAN_POINT('Ctrl Pts',(0.00128084268067104,-0.0173787743898758,
-0.014646071767013));
#39338=CARTESIAN_POINT('Ctrl Pts',(0.0012664895905635,-0.0173787743898758,
-0.0146552185370977));
#39339=CARTESIAN_POINT('Ctrl Pts',(0.00125204156802668,-0.0173787743898758,
-0.0146642365899005));
#39340=CARTESIAN_POINT('Ctrl Pts',(0.00123750060782707,-0.0173787743898757,
-0.0146731254295959));
#39341=CARTESIAN_POINT('Ctrl Pts',(0.0012250706672739,-0.0173787743898757,
-0.014680723810135));
#39342=CARTESIAN_POINT('Ctrl Pts',(0.00121258012573586,-0.0173787743898757,
-0.0146882232766687));
#39343=CARTESIAN_POINT('Ctrl Pts',(0.00120003402569006,-0.0173787743898757,
-0.0146956217909455));
#39344=CARTESIAN_POINT('Ctrl Pts',(0.000904617897650414,-0.0173787743898755,
-0.0148698305437002));
#39345=CARTESIAN_POINT('Ctrl Pts',(0.000578281544735326,-0.0173787743898752,
-0.0149889800424757));
#39346=CARTESIAN_POINT('Ctrl Pts',(0.000238503122206503,-0.0173787743898748,
-0.0150506991599622));
#39347=CARTESIAN_POINT('Ctrl Pts',(0.000218843683908667,-0.0173787743898748,
-0.0150542702024463));
#39348=CARTESIAN_POINT('Ctrl Pts',(0.000199132992020951,-0.0173787743898748,
-0.0150576477208599));
#39349=CARTESIAN_POINT('Ctrl Pts',(0.000179404432188849,-0.0173787743898747,
-0.0150608259170612));
#39350=CARTESIAN_POINT('Ctrl Pts',(8.08486648710589E-5,-0.0173787743898746,
-0.0150767028775679));
#39351=CARTESIAN_POINT('Ctrl Pts',(-1.82764467995728E-5,-0.0173787743898737,
-0.0150876344329206));
#39352=CARTESIAN_POINT('Ctrl Pts',(-0.00011755903599944,-0.0173787743898738,
-0.0150935879009351));
#39353=CARTESIAN_POINT('Ctrl Pts',(-0.000314661884901832,-0.0173787743898741,
-0.015105407148559));
#39354=CARTESIAN_POINT('Ctrl Pts',(-0.000512377756271194,-0.0173787743898745,
-0.0150976565743765));
#39355=CARTESIAN_POINT('Ctrl Pts',(-0.000707721724771412,-0.0173787743898747,
-0.0150695266038167));
#39356=CARTESIAN_POINT('Ctrl Pts',(-0.000781218199492438,-0.0173787743898748,
-0.0150589429462509));
#39357=CARTESIAN_POINT('Ctrl Pts',(-0.000854380568763212,-0.0173787743898749,
-0.0150454663912922));
#39358=CARTESIAN_POINT('Ctrl Pts',(-0.00092705098312487,-0.0173787743898723,
-0.0150290228354436));
#39359=CARTESIAN_POINT('Origin',(0.,-0.0173787743898623,-0.0121758532865581));
#39360=CARTESIAN_POINT('Ctrl Pts',(-0.00176576417784588,-0.0274694134009467,
-0.0104108140867378));
#39361=CARTESIAN_POINT('Ctrl Pts',(-0.00118292095981484,-0.0274168573249058,
-0.0098277128924115));
#39362=CARTESIAN_POINT('Ctrl Pts',(0.00059527173215891,-0.0273117560658722,
-0.00929359972128072));
#39363=CARTESIAN_POINT('Ctrl Pts',(0.00274092821966559,-0.0271541096238461,
-0.011096746535157));
#39364=CARTESIAN_POINT('Ctrl Pts',(0.00240319207333727,-0.0269964740748679,
-0.0138747749556991));
#39365=CARTESIAN_POINT('Ctrl Pts',(-0.000101975422128609,-0.02683883852589,
-0.015117915947344));
#39366=CARTESIAN_POINT('Ctrl Pts',(-0.0025168541262501,-0.0266812029769119,
-0.0137033259019318));
#39367=CARTESIAN_POINT('Ctrl Pts',(-0.00265711008968434,-0.0265235674279339,
-0.0109088159045253));
#39368=CARTESIAN_POINT('Ctrl Pts',(-0.000397484020939204,-0.0263659318789558,
-0.00925893793215084));
#39369=CARTESIAN_POINT('Ctrl Pts',(0.00222147717336516,-0.0262082963299777,
-0.0102441291704481));
#39370=CARTESIAN_POINT('Ctrl Pts',(0.00283347043813024,-0.0260506607809997,
-0.0129744031307677));
#39371=CARTESIAN_POINT('Ctrl Pts',(0.000885836877589451,-0.0258930252320217,
-0.014983281882999));
#39372=CARTESIAN_POINT('Ctrl Pts',(-0.00186207862087175,-0.0257353896830436,
-0.0144559914602417));
#39373=CARTESIAN_POINT('Ctrl Pts',(-0.00292781373092146,-0.0255777541340656,
-0.0118688726936714));
#39374=CARTESIAN_POINT('Ctrl Pts',(-0.00134863475409321,-0.0254201185850875,
-0.00955907392664864));
#39375=CARTESIAN_POINT('Ctrl Pts',(0.00144887683555256,-0.0252624830361095,
-0.00961321703853231));
#39376=CARTESIAN_POINT('Ctrl Pts',(0.00293750170311061,-0.0251048474871315,
-0.0119823905855329));
#39377=CARTESIAN_POINT('Ctrl Pts',(0.00177245222274447,-0.0249472119381534,
-0.0145263341168514));
#39378=CARTESIAN_POINT('Ctrl Pts',(-0.000993793093215091,-0.0247895763891753,
-0.0149469039637085));
#39379=CARTESIAN_POINT('Ctrl Pts',(-0.00286226678504763,-0.0246319408401973,
-0.0128641663544265));
#39380=CARTESIAN_POINT('Ctrl Pts',(-0.00214503055983681,-0.0244743052912193,
-0.0101596215653044));
#39381=CARTESIAN_POINT('Ctrl Pts',(0.000509980129524932,-0.0243166697422412,
-0.00927649704326958));
#39382=CARTESIAN_POINT('Ctrl Pts',(0.00270428571248687,-0.0241590341932632,
-0.0110125884483945));
#39383=CARTESIAN_POINT('Ctrl Pts',(0.00245559790913657,-0.0240013986442851,
-0.0137995482294608));
#39384=CARTESIAN_POINT('Ctrl Pts',(-1.14241210114808E-5,-0.0238437630953071,
-0.0151196970035421));
#39385=CARTESIAN_POINT('Ctrl Pts',(-0.00246812583927738,-0.0236861275463291,
-0.0137804408273949));
#39386=CARTESIAN_POINT('Ctrl Pts',(-0.00269517588644093,-0.023528491997351,
-0.0109916348590015));
#39387=CARTESIAN_POINT('Ctrl Pts',(-0.000487462138964281,-0.023370856448373,
-0.00927262628838117));
#39388=CARTESIAN_POINT('Ctrl Pts',(0.00216061439503312,-0.0232132208993949,
-0.0101763303996177));
#39389=CARTESIAN_POINT('Ctrl Pts',(0.00285683846403066,-0.0230555853504169,
-0.0128863603807944));
#39390=CARTESIAN_POINT('Ctrl Pts',(0.000972256252628799,-0.0228979498014388,
-0.0149545335702968));
#39391=CARTESIAN_POINT('Ctrl Pts',(-0.00179064129716749,-0.0227403142524608,
-0.0145125068947971));
#39392=CARTESIAN_POINT('Ctrl Pts',(-0.00293591210216717,-0.0225826787034828,
-0.0119595977236454));
#39393=CARTESIAN_POINT('Ctrl Pts',(-0.00142894320700064,-0.0224250431545047,
-0.00960204916595687));
#39394=CARTESIAN_POINT('Ctrl Pts',(0.0013689021759258,-0.0222674076055267,
-0.0095696197642336));
#39395=CARTESIAN_POINT('Ctrl Pts',(0.00293011084416917,-0.0221097720565486,
-0.0118916055409205));
#39396=CARTESIAN_POINT('Ctrl Pts',(0.00184432054372579,-0.0219521365075706,
-0.014470374603087));
#39397=CARTESIAN_POINT('Ctrl Pts',(-0.000907589175775288,-0.0217945009585925,
-0.0149763225737564));
#39398=CARTESIAN_POINT('Ctrl Pts',(-0.00283960239971302,-0.0216368654096145,
-0.0129523869632051));
#39399=CARTESIAN_POINT('Ctrl Pts',(-0.00220638003274556,-0.0214792298606364,
-0.010226947570273));
#39400=CARTESIAN_POINT('Ctrl Pts',(0.000420038490802218,-0.0213215943116584,
-0.00926210758570121));
#39401=CARTESIAN_POINT('Ctrl Pts',(0.00266700329593708,-0.0211639587626804,
-0.0109294826538095));
#39402=CARTESIAN_POINT('Ctrl Pts',(0.00250465482140347,-0.0210063232137023,
-0.0137228020789193));
#39403=CARTESIAN_POINT('Ctrl Pts',(7.96551729982372E-5,-0.0208486876647243,
-0.0151186413204434));
#39404=CARTESIAN_POINT('Ctrl Pts',(-0.00241730323367411,-0.0206910521157462,
-0.0138560292817851));
#39405=CARTESIAN_POINT('Ctrl Pts',(-0.00273052202674609,-0.0205334165667682,
-0.0110755824928619));
#39406=CARTESIAN_POINT('Ctrl Pts',(-0.000577046057097934,-0.0203757810177901,
-0.00928909657626689));
#39407=CARTESIAN_POINT('Ctrl Pts',(0.00209772082487443,-0.0202181454688121,
-0.0101104445209445));
#39408=CARTESIAN_POINT('Ctrl Pts',(0.00287745204370962,-0.020060509919834,
-0.0127976380592968));
#39409=CARTESIAN_POINT('Ctrl Pts',(0.0010577549130369,-0.019902874370856,
-0.0149231249439365));
#39410=CARTESIAN_POINT('Ctrl Pts',(-0.00171749480653482,-0.019745238821878,
-0.0145667852517114));
#39411=CARTESIAN_POINT('Ctrl Pts',(-0.00294119750658452,-0.0195876032728999,
-0.0120505302976156));
#39412=CARTESIAN_POINT('Ctrl Pts',(-0.00150788431839104,-0.0194299677239219,
-0.0096474872527832));
#39413=CARTESIAN_POINT('Ctrl Pts',(0.00128761623108036,-0.0192723321749438,
-0.00952851976604358));
#39414=CARTESIAN_POINT('Ctrl Pts',(0.00291991747238735,-0.0191146966259658,
-0.0118010882457072));
#39415=CARTESIAN_POINT('Ctrl Pts',(0.00191441775473846,-0.0189570610769877,
-0.0144122269043048));
#39416=CARTESIAN_POINT('Ctrl Pts',(-0.000820505555265474,-0.0187994255280097,
-0.0150030439789635));
#39417=CARTESIAN_POINT('Ctrl Pts',(-0.00281424058814684,-0.0186417899790317,
-0.0130398954178051));
#39418=CARTESIAN_POINT('Ctrl Pts',(-0.00226557676094723,-0.0184841544300536,
-0.0102960791852537));
#39419=CARTESIAN_POINT('Ctrl Pts',(0.000329616729494906,-0.0183265188810756,
-0.00925062328400989));
#39420=CARTESIAN_POINT('Ctrl Pts',(0.00262731783985433,-0.0181688833320975,
-0.0108473472640193));
#39421=CARTESIAN_POINT('Ctrl Pts',(0.00255102483355773,-0.0180112477831195,
-0.0136450040566565));
#39422=CARTESIAN_POINT('Ctrl Pts',(0.000171215685035621,-0.0178536122341414,
-0.0151139397673183));
#39423=CARTESIAN_POINT('Ctrl Pts',(-0.00236524911441394,-0.0176959766851634,
-0.0139316310381663));
#39424=CARTESIAN_POINT('Ctrl Pts',(-0.00276110049454826,-0.0175383326154246,
-0.0111570598155219));
#39425=CARTESIAN_POINT('Ctrl Pts',(-0.00136756358585242,-0.0174332337286785,
-0.00993024457820385));
#39426=CARTESIAN_POINT('Ctrl Pts',(-0.000564501289899483,-0.017380680024925,
-0.00974385311997074));
#39427=CARTESIAN_POINT('Ctrl Pts',(-0.00188620817627642,-0.0273710914741913,
-0.0102904195395609));
#39428=CARTESIAN_POINT('Ctrl Pts',(-0.00126360881837204,-0.0273185353981504,
-0.00966754460861935));
#39429=CARTESIAN_POINT('Ctrl Pts',(0.000635875629595165,-0.0272134341391169,
-0.00909699920788931));
#39430=CARTESIAN_POINT('Ctrl Pts',(0.00292788883327953,-0.0270557876970907,
-0.01102313991571));
#39431=CARTESIAN_POINT('Ctrl Pts',(0.00256711547032362,-0.0268981521481127,
-0.013990659580282));
#39432=CARTESIAN_POINT('Ctrl Pts',(-0.000108931236351646,-0.0267405165991346,
-0.0153185960805941));
#39433=CARTESIAN_POINT('Ctrl Pts',(-0.00268853049064535,-0.0265828810501566,
-0.0138075158677251));
#39434=CARTESIAN_POINT('Ctrl Pts',(-0.00283835341055753,-0.0264252455011785,
-0.0108223904065071));
#39435=CARTESIAN_POINT('Ctrl Pts',(-0.000424596681505571,-0.0262676099522004,
-0.00905997311409863));
#39436=CARTESIAN_POINT('Ctrl Pts',(0.00237300567107693,-0.0261099744032224,
-0.010112364929601));
#39437=CARTESIAN_POINT('Ctrl Pts',(0.00302674342060714,-0.0259523388542444,
-0.0130288727691199));
#39438=CARTESIAN_POINT('Ctrl Pts',(0.000946260424987647,-0.0257947033052664,
-0.0151747785334045));
#39439=CARTESIAN_POINT('Ctrl Pts',(-0.00198909229421707,-0.0256370677562883,
-0.0146115212654435));
#39440=CARTESIAN_POINT('Ctrl Pts',(-0.00312752193478945,-0.0254794322073103,
-0.0118479333346609));
#39441=CARTESIAN_POINT('Ctrl Pts',(-0.00144062606541516,-0.0253217966583322,
-0.00938058159280683));
#39442=CARTESIAN_POINT('Ctrl Pts',(0.0015477057287291,-0.0251641611093541,
-0.00943841784387892));
#39443=CARTESIAN_POINT('Ctrl Pts',(0.0031378707302764,-0.0250065255603761,
-0.0119691943606062));
#39444=CARTESIAN_POINT('Ctrl Pts',(0.00189335241735305,-0.0248488900113981,
-0.0146866620434152));
#39445=CARTESIAN_POINT('Ctrl Pts',(-0.00106158040890607,-0.02469125446242,
-0.0151359192510257));
#39446=CARTESIAN_POINT('Ctrl Pts',(-0.00305750398630663,-0.024533618913442,
-0.012911116665859));
#39447=CARTESIAN_POINT('Ctrl Pts',(-0.00229134458105431,-0.024375983364464,
-0.0100220930021377));
#39448=CARTESIAN_POINT('Ctrl Pts',(0.000544766227629503,-0.0242183478154859,
-0.00907872994435708));
#39449=CARTESIAN_POINT('Ctrl Pts',(0.00288874691528906,-0.0240607122665079,
-0.0109332413475189));
#39450=CARTESIAN_POINT('Ctrl Pts',(0.00262309594450553,-0.0239030767175298,
-0.0139103015869071));
#39451=CARTESIAN_POINT('Ctrl Pts',(-1.22033682237757E-5,-0.0237454411685518,
-0.0153204986238699));
#39452=CARTESIAN_POINT('Ctrl Pts',(-0.00263647841344439,-0.0235878056195737,
-0.0138898908557028));
#39453=CARTESIAN_POINT('Ctrl Pts',(-0.00287901570169447,-0.0234301700705957,
-0.0109108584992703));
#39454=CARTESIAN_POINT('Ctrl Pts',(-0.000520712269325407,-0.0232725345216176,
-0.00907459516259491));
#39455=CARTESIAN_POINT('Ctrl Pts',(0.00230799140045058,-0.0231148989726396,
-0.0100399415576206));
#39456=CARTESIAN_POINT('Ctrl Pts',(0.00305170539575071,-0.0229572634236615,
-0.0129348245621481));
#39457=CARTESIAN_POINT('Ctrl Pts',(0.00103857452549612,-0.0227996278746835,
-0.0151440692783674));
#39458=CARTESIAN_POINT('Ctrl Pts',(-0.0019127821811494,-0.0226419923257055,
-0.014671891656961));
#39459=CARTESIAN_POINT('Ctrl Pts',(-0.00313617270155084,-0.0224843567767274,
-0.0119448467818114));
#39460=CARTESIAN_POINT('Ctrl Pts',(-0.00152641241355761,-0.0223267212277494,
-0.00942648820297463));
#39461=CARTESIAN_POINT('Ctrl Pts',(0.00146227594213839,-0.0221690856787713,
-0.00939184676928282));
#39462=CARTESIAN_POINT('Ctrl Pts',(0.0031299757357239,-0.0220114501297933,
-0.011872216805177));
#39463=CARTESIAN_POINT('Ctrl Pts',(0.0019701229263208,-0.0218538145808152,
-0.0146268854924312));
#39464=CARTESIAN_POINT('Ctrl Pts',(-0.000969496462509344,-0.0216961790318372,
-0.0151673445248549));
#39465=CARTESIAN_POINT('Ctrl Pts',(-0.00303329364753954,-0.0215385434828592,
-0.0130053548635084));
#39466=CARTESIAN_POINT('Ctrl Pts',(-0.00235687874403178,-0.0213809079338811,
-0.0100940113605692));
#39467=CARTESIAN_POINT('Ctrl Pts',(0.000448689607390529,-0.0212232723849031,
-0.00906335897191456));
#39468=CARTESIAN_POINT('Ctrl Pts',(0.00284892143926579,-0.021065636835925,
-0.0108444668490842));
#39469=CARTESIAN_POINT('Ctrl Pts',(0.00267549906275975,-0.020908001286947,
-0.0138283205282439));
#39470=CARTESIAN_POINT('Ctrl Pts',(8.50885075578431E-5,-0.0207503657379689,
-0.0153193709318953));
#39471=CARTESIAN_POINT('Ctrl Pts',(-0.00258218916268753,-0.0205927301889909,
-0.0139706352509576));
#39472=CARTESIAN_POINT('Ctrl Pts',(-0.00291677282672843,-0.0204350946400128,
-0.0110005322594209));
#39473=CARTESIAN_POINT('Ctrl Pts',(-0.000616406768606,-0.0202774590910348,
-0.00909218890023294));
#39474=CARTESIAN_POINT('Ctrl Pts',(0.00224080781627953,-0.0201198235420567,
-0.00996956155749723));
#39475=CARTESIAN_POINT('Ctrl Pts',(0.00307372504198695,-0.0199621879930787,
-0.0128400504296073));
#39476=CARTESIAN_POINT('Ctrl Pts',(0.00112990510879018,-0.0198045524441007,
-0.0151105182478334));
#39477=CARTESIAN_POINT('Ctrl Pts',(-0.00183464631769248,-0.0196469168951226,
-0.0147298723782209));
#39478=CARTESIAN_POINT('Ctrl Pts',(-0.00314181862706683,-0.0194892813461446,
-0.012041981929678));
#39479=CARTESIAN_POINT('Ctrl Pts',(-0.0016107381528704,-0.0193316457971665,
-0.00947502565319674));
#39480=CARTESIAN_POINT('Ctrl Pts',(0.00137544542665535,-0.0191740102481885,
-0.00934794331172965));
#39481=CARTESIAN_POINT('Ctrl Pts',(0.00311908706698777,-0.0190163746992104,
-0.0117755252625193));
#39482=CARTESIAN_POINT('Ctrl Pts',(0.00204500151668136,-0.0188587391502324,
-0.0145647714988127));
#39483=CARTESIAN_POINT('Ctrl Pts',(-0.000876472807886479,-0.0187011036012544,
-0.015195888615632));
#39484=CARTESIAN_POINT('Ctrl Pts',(-0.00300620188922807,-0.0185434680522763,
-0.0130988323304493));
#39485=CARTESIAN_POINT('Ctrl Pts',(-0.00242011332209363,-0.0183858325032983,
-0.0101678584909233));
#39486=CARTESIAN_POINT('Ctrl Pts',(0.000352100115072687,-0.0182281969543202,
-0.00905109131804506));
#39487=CARTESIAN_POINT('Ctrl Pts',(0.00280652901071745,-0.0180705614053422,
-0.010756728947428));
#39488=CARTESIAN_POINT('Ctrl Pts',(0.00272503200558233,-0.0179129258563641,
-0.0137452158489603));
#39489=CARTESIAN_POINT('Ctrl Pts',(0.000182894425582328,-0.0177552903073861,
-0.0153143486825729));
#39490=CARTESIAN_POINT('Ctrl Pts',(-0.00252658439587369,-0.017597654758408,
-0.0140513938555416));
#39491=CARTESIAN_POINT('Ctrl Pts',(-0.00294943707301346,-0.0174400106886692,
-0.0110875672067319));
#39492=CARTESIAN_POINT('Ctrl Pts',(-0.00146084604590834,-0.0173349118019229,
-0.0097770700517648));
#39493=CARTESIAN_POINT('Ctrl Pts',(-0.000603006314142103,-0.0172823580981696,
-0.00957796470297678));
#39494=CARTESIAN_POINT('Ctrl Pts',(-0.00200665217470697,-0.0272727695474359,
-0.010170024992384));
#39495=CARTESIAN_POINT('Ctrl Pts',(-0.00134429667692924,-0.0272202134713949,
-0.00950737632482718));
#39496=CARTESIAN_POINT('Ctrl Pts',(0.000676479527031423,-0.0271151122123614,
-0.00890039869449788));
#39497=CARTESIAN_POINT('Ctrl Pts',(0.00311484944689349,-0.0269574657703352,
-0.0109495332962628));
#39498=CARTESIAN_POINT('Ctrl Pts',(0.00273103886730998,-0.0267998302213571,
-0.0141065442048648));
#39499=CARTESIAN_POINT('Ctrl Pts',(-0.000115887050574685,-0.026642194672379,
-0.0155192762138441));
#39500=CARTESIAN_POINT('Ctrl Pts',(-0.00286020685504059,-0.026484559123401,
-0.0139117058335183));
#39501=CARTESIAN_POINT('Ctrl Pts',(-0.00301959673143072,-0.026326923574423,
-0.0107359649084888));
#39502=CARTESIAN_POINT('Ctrl Pts',(-0.000451709342071937,-0.026169288025445,
-0.00886100829604641));
#39503=CARTESIAN_POINT('Ctrl Pts',(0.00252453416878869,-0.0260116524764669,
-0.00998060068875387));
#39504=CARTESIAN_POINT('Ctrl Pts',(0.00322001640308403,-0.0258540169274889,
-0.0130833424074723));
#39505=CARTESIAN_POINT('Ctrl Pts',(0.00100668397238585,-0.0256963813785108,
-0.01536627518381));
#39506=CARTESIAN_POINT('Ctrl Pts',(-0.00211610596756238,-0.0255387458295328,
-0.0147670510706451));
#39507=CARTESIAN_POINT('Ctrl Pts',(-0.00332723013865741,-0.0253811102805547,
-0.0118269939756503));
#39508=CARTESIAN_POINT('Ctrl Pts',(-0.00153261737673712,-0.0252234747315767,
-0.00920208925896502));
#39509=CARTESIAN_POINT('Ctrl Pts',(0.00164653462190566,-0.0250658391825986,
-0.00926361864922554));
#39510=CARTESIAN_POINT('Ctrl Pts',(0.00333823975744216,-0.0249082036336206,
-0.0119559981356793));
#39511=CARTESIAN_POINT('Ctrl Pts',(0.00201425261196165,-0.0247505680846425,
-0.0148469899699792));
#39512=CARTESIAN_POINT('Ctrl Pts',(-0.00112936772459704,-0.0245929325356645,
-0.0153249345383428));
#39513=CARTESIAN_POINT('Ctrl Pts',(-0.00325274118756563,-0.0244352969866865,
-0.0129580669772913));
#39514=CARTESIAN_POINT('Ctrl Pts',(-0.00243765860227181,-0.0242776614377084,
-0.00988456443897111));
#39515=CARTESIAN_POINT('Ctrl Pts',(0.000579552325734072,-0.0241200258887304,
-0.00888096284544458));
#39516=CARTESIAN_POINT('Ctrl Pts',(0.00307320811809126,-0.0239623903397523,
-0.0108538942466433));
#39517=CARTESIAN_POINT('Ctrl Pts',(0.00279059397987449,-0.0238047547907743,
-0.0140210549443533));
#39518=CARTESIAN_POINT('Ctrl Pts',(-1.29826154360689E-5,-0.0236471192417962,
-0.0155213002441977));
#39519=CARTESIAN_POINT('Ctrl Pts',(-0.00280483098761143,-0.0234894836928182,
-0.0139993408840106));
#39520=CARTESIAN_POINT('Ctrl Pts',(-0.00306285551694802,-0.0233318481438402,
-0.0108300821395392));
#39521=CARTESIAN_POINT('Ctrl Pts',(-0.000553962399686529,-0.0231742125948621,
-0.00887656403680862));
#39522=CARTESIAN_POINT('Ctrl Pts',(0.00245536840586803,-0.0230165770458841,
-0.0099035527156234));
#39523=CARTESIAN_POINT('Ctrl Pts',(0.00324657232747075,-0.022858941496906,
-0.0129832887435019));
#39524=CARTESIAN_POINT('Ctrl Pts',(0.00110489279836343,-0.022701305947928,
-0.0153336049864378));
#39525=CARTESIAN_POINT('Ctrl Pts',(-0.0020349230651313,-0.0225436703989499,
-0.0148312764191248));
#39526=CARTESIAN_POINT('Ctrl Pts',(-0.00333643330093449,-0.0223860348499719,
-0.0119300958399773));
#39527=CARTESIAN_POINT('Ctrl Pts',(-0.00162388162011455,-0.0222283993009938,
-0.00925092723999238));
#39528=CARTESIAN_POINT('Ctrl Pts',(0.00155564970835097,-0.0220707637520158,
-0.00921407377433204));
#39529=CARTESIAN_POINT('Ctrl Pts',(0.00332984062727863,-0.0219131282030377,
-0.0118528280694337));
#39530=CARTESIAN_POINT('Ctrl Pts',(0.0020959253089158,-0.0217554926540597,
-0.0147833963817754));
#39531=CARTESIAN_POINT('Ctrl Pts',(-0.0010314037492434,-0.0215978571050817,
-0.0153583664759535));
#39532=CARTESIAN_POINT('Ctrl Pts',(-0.00322698489536608,-0.0214402215561036,
-0.0130583227638117));
#39533=CARTESIAN_POINT('Ctrl Pts',(-0.002507377455318,-0.0212825860071256,
-0.00996107515086551));
#39534=CARTESIAN_POINT('Ctrl Pts',(0.000477340723978841,-0.0211249504581475,
-0.00886461035812792));
#39535=CARTESIAN_POINT('Ctrl Pts',(0.0030308395825945,-0.0209673149091695,
-0.0107594510443588));
#39536=CARTESIAN_POINT('Ctrl Pts',(0.00284634330411602,-0.0208096793601914,
-0.0139338389775685));
#39537=CARTESIAN_POINT('Ctrl Pts',(9.0521842117449E-5,-0.0206520438112134,
-0.0155201005433471));
#39538=CARTESIAN_POINT('Ctrl Pts',(-0.00274707509170096,-0.0204944082622354,
-0.0140852412201302));
#39539=CARTESIAN_POINT('Ctrl Pts',(-0.00310302362671076,-0.0203367727132573,
-0.0109254820259798));
#39540=CARTESIAN_POINT('Ctrl Pts',(-0.000655767480114067,-0.0201791371642793,
-0.00889528122419899));
#39541=CARTESIAN_POINT('Ctrl Pts',(0.00238389480768462,-0.0200215016153012,
-0.00982867859404995));
#39542=CARTESIAN_POINT('Ctrl Pts',(0.00326999804026427,-0.0198638660663232,
-0.0128824627999178));
#39543=CARTESIAN_POINT('Ctrl Pts',(0.00120205530454347,-0.0197062305173451,
-0.0152979115517304));
#39544=CARTESIAN_POINT('Ctrl Pts',(-0.00195179782885014,-0.0195485949683671,
-0.0148929595047305));
#39545=CARTESIAN_POINT('Ctrl Pts',(-0.00334243974754914,-0.019390959419389,
-0.0120334335617402));
#39546=CARTESIAN_POINT('Ctrl Pts',(-0.00171359198734975,-0.019233323870411,
-0.00930256405361027));
#39547=CARTESIAN_POINT('Ctrl Pts',(0.00146327462223035,-0.0190756883214329,
-0.00916736685741573));
#39548=CARTESIAN_POINT('Ctrl Pts',(0.00331825666158819,-0.0189180527724549,
-0.0117499622793314));
#39549=CARTESIAN_POINT('Ctrl Pts',(0.00217558527862425,-0.0187604172234769,
-0.0147173160933204));
#39550=CARTESIAN_POINT('Ctrl Pts',(-0.000932440060507479,-0.0186027816744988,
-0.0153887332523004));
#39551=CARTESIAN_POINT('Ctrl Pts',(-0.00319816319030928,-0.0184451461255208,
-0.0131577692430934));
#39552=CARTESIAN_POINT('Ctrl Pts',(-0.00257464988324002,-0.0182875105765427,
-0.0100396377965929));
#39553=CARTESIAN_POINT('Ctrl Pts',(0.000374583500650467,-0.0181298750275647,
-0.00885155935208023));
#39554=CARTESIAN_POINT('Ctrl Pts',(0.00298574018158057,-0.0179722394785867,
-0.0106661106308367));
#39555=CARTESIAN_POINT('Ctrl Pts',(0.00289903917760691,-0.0178146039296086,
-0.0138454276412644));
#39556=CARTESIAN_POINT('Ctrl Pts',(0.000194573166129036,-0.0176569683806306,
-0.0155147575978273));
#39557=CARTESIAN_POINT('Ctrl Pts',(-0.00268791967733341,-0.0174993328316525,
-0.0141711566729167));
#39558=CARTESIAN_POINT('Ctrl Pts',(-0.00313777365147868,-0.0173416887619137,
-0.0110180745979418));
#39559=CARTESIAN_POINT('Ctrl Pts',(-0.00155412850596426,-0.0172365898751676,
-0.00962389552532573));
#39560=CARTESIAN_POINT('Ctrl Pts',(-0.000641511338384723,-0.0171840361714141,
-0.00941207628598281));
#39561=CARTESIAN_POINT('Ctrl Pts',(-0.0021270961731375,-0.0271744476206803,
-0.010049630445207));
#39562=CARTESIAN_POINT('Ctrl Pts',(-0.00142498453548643,-0.0271218915446394,
-0.00934720804103501));
#39563=CARTESIAN_POINT('Ctrl Pts',(0.000717083424467678,-0.0270167902856059,
-0.00870379818110647));
#39564=CARTESIAN_POINT('Ctrl Pts',(0.00330181006050744,-0.0268591438435796,
-0.0108759266768156));
#39565=CARTESIAN_POINT('Ctrl Pts',(0.00289496226429633,-0.0267015082946015,
-0.0142224288294477));
#39566=CARTESIAN_POINT('Ctrl Pts',(-0.000122842864797722,-0.0265438727456235,
-0.0157199563470941));
#39567=CARTESIAN_POINT('Ctrl Pts',(-0.00303188321943583,-0.0263862371966456,
-0.0140158957993116));
#39568=CARTESIAN_POINT('Ctrl Pts',(-0.00320084005230392,-0.0262286016476674,
-0.0106495394104707));
#39569=CARTESIAN_POINT('Ctrl Pts',(-0.000478822002638301,-0.0260709660986895,
-0.0086620434779942));
#39570=CARTESIAN_POINT('Ctrl Pts',(0.00267606266650046,-0.0259133305497115,
-0.0098488364479067));
#39571=CARTESIAN_POINT('Ctrl Pts',(0.00341328938556092,-0.0257556950007333,
-0.0131378120458245));
#39572=CARTESIAN_POINT('Ctrl Pts',(0.00106710751978404,-0.0255980594517554,
-0.0155577718342156));
#39573=CARTESIAN_POINT('Ctrl Pts',(-0.0022431196409077,-0.0254404239027772,
-0.0149225808758469));
#39574=CARTESIAN_POINT('Ctrl Pts',(-0.00352693834252537,-0.0252827883537992,
-0.0118060546166399));
#39575=CARTESIAN_POINT('Ctrl Pts',(-0.00162460868805907,-0.0251251528048211,
-0.00902359692512321));
#39576=CARTESIAN_POINT('Ctrl Pts',(0.0017453635150822,-0.0249675172558432,
-0.00908881945457216));
#39577=CARTESIAN_POINT('Ctrl Pts',(0.00353860878460794,-0.024809881706865,
-0.0119428019107525));
#39578=CARTESIAN_POINT('Ctrl Pts',(0.00213515280657024,-0.024652246157887,
-0.015007317896543));
#39579=CARTESIAN_POINT('Ctrl Pts',(-0.00119715504028801,-0.0244946106089089,
-0.0155139498256597));
#39580=CARTESIAN_POINT('Ctrl Pts',(-0.00344797838882464,-0.0243369750599309,
-0.0130050172887238));
#39581=CARTESIAN_POINT('Ctrl Pts',(-0.00258397262348931,-0.0241793395109529,
-0.00974703587580447));
#39582=CARTESIAN_POINT('Ctrl Pts',(0.000614338423838643,-0.0240217039619748,
-0.00868319574653206));
#39583=CARTESIAN_POINT('Ctrl Pts',(0.00325766932089345,-0.0238640684129969,
-0.0107745471457676));
#39584=CARTESIAN_POINT('Ctrl Pts',(0.00295809201524345,-0.0237064328640187,
-0.0141318083017995));
#39585=CARTESIAN_POINT('Ctrl Pts',(-1.37618626483643E-5,-0.0235487973150408,
-0.0157221018645255));
#39586=CARTESIAN_POINT('Ctrl Pts',(-0.00297318356177844,-0.0233911617660626,
-0.0141087909123184));
#39587=CARTESIAN_POINT('Ctrl Pts',(-0.00324669533220156,-0.0232335262170846,
-0.010749305779808));
#39588=CARTESIAN_POINT('Ctrl Pts',(-0.000587212530047655,-0.0230758906681066,
-0.00867853291102234));
#39589=CARTESIAN_POINT('Ctrl Pts',(0.00260274541128548,-0.0229182551191285,
-0.00976716387362624));
#39590=CARTESIAN_POINT('Ctrl Pts',(0.0034414392591908,-0.0227606195701505,
-0.0130317529248556));
#39591=CARTESIAN_POINT('Ctrl Pts',(0.00117121107123076,-0.0226029840211724,
-0.0155231406945085));
#39592=CARTESIAN_POINT('Ctrl Pts',(-0.0021570639491132,-0.0224453484721945,
-0.0149906611812887));
#39593=CARTESIAN_POINT('Ctrl Pts',(-0.00353669390031815,-0.0222877129232163,
-0.0119153448981433));
#39594=CARTESIAN_POINT('Ctrl Pts',(-0.0017213508266715,-0.0221300773742383,
-0.00907536627701014));
#39595=CARTESIAN_POINT('Ctrl Pts',(0.00164902347456355,-0.0219724418252602,
-0.00903630077938126));
#39596=CARTESIAN_POINT('Ctrl Pts',(0.00352970551883337,-0.0218148062762822,
-0.0118334393336902));
#39597=CARTESIAN_POINT('Ctrl Pts',(0.00222172769151081,-0.0216571707273041,
-0.0149399072711196));
#39598=CARTESIAN_POINT('Ctrl Pts',(-0.00109331103597745,-0.0214995351783261,
-0.015549388427052));
#39599=CARTESIAN_POINT('Ctrl Pts',(-0.00342067614319262,-0.0213418996293481,
-0.013111290664115));
#39600=CARTESIAN_POINT('Ctrl Pts',(-0.00265787616660422,-0.02118426408037,
-0.00982813894116177));
#39601=CARTESIAN_POINT('Ctrl Pts',(0.000505991840567147,-0.021026628531392,
-0.00866586174434128));
#39602=CARTESIAN_POINT('Ctrl Pts',(0.00321275772592322,-0.020868992982414,
-0.0106744352396337));
#39603=CARTESIAN_POINT('Ctrl Pts',(0.00301718754547228,-0.020711357433436,
-0.0140393574268932));
#39604=CARTESIAN_POINT('Ctrl Pts',(9.59551766770587E-5,-0.0205537218844579,
-0.0157208301547992));
#39605=CARTESIAN_POINT('Ctrl Pts',(-0.00291196102071441,-0.0203960863354798,
-0.0141998471893027));
#39606=CARTESIAN_POINT('Ctrl Pts',(-0.00328927442669309,-0.0202384507865018,
-0.010850431792539));
#39607=CARTESIAN_POINT('Ctrl Pts',(-0.000695128191622135,-0.0200808152375237,
-0.00869837354816502));
#39608=CARTESIAN_POINT('Ctrl Pts',(0.00252698179908972,-0.0199231796885458,
-0.00968779563060266));
#39609=CARTESIAN_POINT('Ctrl Pts',(0.00346627103854158,-0.0197655441395676,
-0.0129248751702283));
#39610=CARTESIAN_POINT('Ctrl Pts',(0.00127420550029675,-0.0196079085905897,
-0.0154853048556274));
#39611=CARTESIAN_POINT('Ctrl Pts',(-0.0020689493400078,-0.0194502730416115,
-0.0150560466312401));
#39612=CARTESIAN_POINT('Ctrl Pts',(-0.00354306086803145,-0.0192926374926335,
-0.0120248851938025));
#39613=CARTESIAN_POINT('Ctrl Pts',(-0.00181644582182911,-0.0191350019436555,
-0.00913010245402381));
#39614=CARTESIAN_POINT('Ctrl Pts',(0.00155110381780535,-0.0189773663946774,
-0.0089867904031018));
#39615=CARTESIAN_POINT('Ctrl Pts',(0.0035174262561886,-0.0188197308456995,
-0.0117243992961435));
#39616=CARTESIAN_POINT('Ctrl Pts',(0.00230616904056715,-0.0186620952967213,
-0.0148698606878284));
#39617=CARTESIAN_POINT('Ctrl Pts',(-0.000988407313128485,-0.0185044597477434,
-0.0155815778889689));
#39618=CARTESIAN_POINT('Ctrl Pts',(-0.0033901244913905,-0.0183468241987653,
-0.0132167061557375));
#39619=CARTESIAN_POINT('Ctrl Pts',(-0.00272918644438642,-0.0181891886497872,
-0.00991141710226236));
#39620=CARTESIAN_POINT('Ctrl Pts',(0.000397066886228245,-0.0180315531008093,
-0.0086520273861154));
#39621=CARTESIAN_POINT('Ctrl Pts',(0.00316495135244369,-0.0178739175518311,
-0.0105754923142454));
#39622=CARTESIAN_POINT('Ctrl Pts',(0.00307304634963151,-0.0177162820028532,
-0.0139456394335682));
#39623=CARTESIAN_POINT('Ctrl Pts',(0.000206251906675747,-0.0175586464538751,
-0.0157151665130819));
#39624=CARTESIAN_POINT('Ctrl Pts',(-0.00284925495879315,-0.017401010904897,
-0.014290919490292));
#39625=CARTESIAN_POINT('Ctrl Pts',(-0.00332611022994388,-0.0172433668351582,
-0.0109485819891518));
#39626=CARTESIAN_POINT('Ctrl Pts',(-0.00164741096602017,-0.0171382679484121,
-0.00947072099888669));
#39627=CARTESIAN_POINT('Ctrl Pts',(-0.000680016362627343,-0.0170857142446586,
-0.00924618786898885));
#39628=CARTESIAN_POINT('Ctrl Pts',(-0.00267260870462009,-0.0173794995011935,
-0.0135402263681242));
#39629=CARTESIAN_POINT('Ctrl Pts',(-0.00267396311369304,-0.0173793789565635,
-0.0135373081584126));
#39630=CARTESIAN_POINT('Ctrl Pts',(-0.00267531279930547,-0.0173792583760944,
-0.0135343877591632));
#39631=CARTESIAN_POINT('Ctrl Pts',(-0.00267800804240615,-0.0173790166708016,
-0.0135285310334481));
#39632=CARTESIAN_POINT('Ctrl Pts',(-0.00267935356128369,-0.0173788955458108,
-0.0135255946920731));
#39633=CARTESIAN_POINT('Ctrl Pts',(-0.00268069430973449,-0.0173787743898751,
-0.0135226561740565));
#39634=CARTESIAN_POINT('Ctrl Pts',(0.00214364697154644,-0.027178774389864,
-0.0108862500897033));
#39635=CARTESIAN_POINT('Ctrl Pts',(0.00200718019753922,-0.0271787743898637,
-0.0105977254813795));
#39636=CARTESIAN_POINT('Ctrl Pts',(0.00181515016014682,-0.0271787743898637,
-0.0103370893624455));
#39637=CARTESIAN_POINT('Ctrl Pts',(0.0015825829649816,-0.0271787743898636,
-0.0101151998101994));
#39638=CARTESIAN_POINT('Ctrl Pts',(0.00156807204491965,-0.0271787743898636,
-0.0101013551166134));
#39639=CARTESIAN_POINT('Ctrl Pts',(0.00155339606635249,-0.0271787743898636,
-0.0100876582609352));
#39640=CARTESIAN_POINT('Ctrl Pts',(0.00153858322606208,-0.0271787743898636,
-0.0100741352287478));
#39641=CARTESIAN_POINT('Ctrl Pts',(0.00130703486088774,-0.0271787743898636,
-0.00986274862538259));
#39642=CARTESIAN_POINT('Ctrl Pts',(0.00104161596381899,-0.0271787743898638,
-0.00969262022738725));
#39643=CARTESIAN_POINT('Ctrl Pts',(0.000754106682302279,-0.0271787743898641,
-0.00957416699352214));
#39644=CARTESIAN_POINT('Ctrl Pts',(0.000721077701908584,-0.0271787743898641,
-0.00956055912139272));
#39645=CARTESIAN_POINT('Ctrl Pts',(0.00068773017489579,-0.0271787743898642,
-0.00954763097757543));
#39646=CARTESIAN_POINT('Ctrl Pts',(0.000654172404124864,-0.0271787743898642,
-0.00953543584602603));
#39647=CARTESIAN_POINT('Ctrl Pts',(0.000621454371281899,-0.0271787743898643,
-0.00952354588118656));
#39648=CARTESIAN_POINT('Ctrl Pts',(0.000588531611466588,-0.0271787743898643,
-0.00951234954431439));
#39649=CARTESIAN_POINT('Ctrl Pts',(0.000555420931463722,-0.0271787743898643,
-0.00950185931133918));
#39650=CARTESIAN_POINT('Ctrl Pts',(0.00038258051039096,-0.0271787743898646,
-0.00944709944882868));
#39651=CARTESIAN_POINT('Ctrl Pts',(0.000204654649537397,-0.0271787743898647,
-0.00941152019527573));
#39652=CARTESIAN_POINT('Ctrl Pts',(2.43336311719498E-5,-0.0271787743898655,
-0.00939382593790338));
#39653=CARTESIAN_POINT('Ctrl Pts',(-7.0449357939566E-5,-0.0271787743898659,
-0.00938452522177465));
#39654=CARTESIAN_POINT('Ctrl Pts',(-0.000165901707066126,-0.0271787743898656,
-0.00938017829844935));
#39655=CARTESIAN_POINT('Ctrl Pts',(-0.000261664269848712,-0.0271787743898654,
-0.00938067795709841));
#39656=CARTESIAN_POINT('Ctrl Pts',(-0.000283370180679184,-0.0271787743898654,
-0.00938079121164974));
#39657=CARTESIAN_POINT('Ctrl Pts',(-0.000305092069150565,-0.0271787743898653,
-0.00938115369090413));
#39658=CARTESIAN_POINT('Ctrl Pts',(-0.000326825803069745,-0.0271787743898653,
-0.00938176453997136));
#39659=CARTESIAN_POINT('Ctrl Pts',(-0.000345831109748606,-0.0271787743898653,
-0.00938229870376947));
#39660=CARTESIAN_POINT('Ctrl Pts',(-0.000364849161917403,-0.0271787743898653,
-0.00938302307415796));
#39661=CARTESIAN_POINT('Ctrl Pts',(-0.000383850544190616,-0.0271787743898652,
-0.00938393558023816));
#39662=CARTESIAN_POINT('Ctrl Pts',(-0.0006742994320196,-0.0271787743898648,
-0.00939788384843884));
#39663=CARTESIAN_POINT('Ctrl Pts',(-0.000961964432259771,-0.0271787743898645,
-0.00945545867279974));
#39664=CARTESIAN_POINT('Ctrl Pts',(-0.00123688275642929,-0.0271787743898642,
-0.00955336079145493));
#39665=CARTESIAN_POINT('Ctrl Pts',(-0.00125242205520696,-0.0271787743898642,
-0.00955889454507919));
#39666=CARTESIAN_POINT('Ctrl Pts',(-0.00126792259952857,-0.0271787743898642,
-0.00956455895934887));
#39667=CARTESIAN_POINT('Ctrl Pts',(-0.00128337643900455,-0.0271787743898642,
-0.00957035152521633));
#39668=CARTESIAN_POINT('Ctrl Pts',(-0.00156303926269199,-0.0271787743898639,
-0.00967517759963037));
#39669=CARTESIAN_POINT('Ctrl Pts',(-0.00182522482013095,-0.0271787743898638,
-0.00982078890803008));
#39670=CARTESIAN_POINT('Ctrl Pts',(-0.0020595896027101,-0.0271787743898637,
-0.0100046652555036));
#39671=CARTESIAN_POINT('Ctrl Pts',(-0.00208038902733874,-0.0271787743898637,
-0.010020983928421));
#39672=CARTESIAN_POINT('Ctrl Pts',(-0.00210096855971851,-0.0271787743898637,
-0.0100376065791357));
#39673=CARTESIAN_POINT('Ctrl Pts',(-0.00212132034355959,-0.0271787743898723,
-0.0100545329429984));
#39674=CARTESIAN_POINT('Ctrl Pts',(0.000734447700009759,-0.027496347211233,
-0.0151361043823298));
#39675=CARTESIAN_POINT('Ctrl Pts',(-0.000243069169262639,-0.0274437919704715,
-0.0153786446838308));
#39676=CARTESIAN_POINT('Ctrl Pts',(-0.0024403684665538,-0.0273386915467173,
-0.0148161659350916));
#39677=CARTESIAN_POINT('Ctrl Pts',(-0.00354831004413418,-0.0271810459399706,
-0.0115765056537264));
#39678=CARTESIAN_POINT('Ctrl Pts',(-0.00144312695496411,-0.0270234103909925,
-0.00888283623912904));
#39679=CARTESIAN_POINT('Ctrl Pts',(0.00196194337287167,-0.0268657748420145,
-0.00916187994792398));
#39680=CARTESIAN_POINT('Ctrl Pts',(0.00359659766777445,-0.0267081392930364,
-0.0121647738576856));
#39681=CARTESIAN_POINT('Ctrl Pts',(0.00198114537143259,-0.0265505037440584,
-0.0151771107943776));
#39682=CARTESIAN_POINT('Ctrl Pts',(-0.00142350210994787,-0.0263928681950803,
-0.0154784703644144));
#39683=CARTESIAN_POINT('Ctrl Pts',(-0.00354246332004805,-0.0262352326461021,
-0.0127961640919714));
#39684=CARTESIAN_POINT('Ctrl Pts',(-0.00246109668429956,-0.0260775970971242,
-0.00955356181364477));
#39685=CARTESIAN_POINT('Ctrl Pts',(0.000843497391267268,-0.025919961548146,
-0.00867983985000952));
#39686=CARTESIAN_POINT('Ctrl Pts',(0.00338613269875458,-0.0257623259991681,
-0.0109643625076157));
#39687=CARTESIAN_POINT('Ctrl Pts',(0.00286978866718684,-0.0256046904501901,
-0.0143433086683626));
#39688=CARTESIAN_POINT('Ctrl Pts',(-0.000239050153610035,-0.025447054901212,
-0.0157642281583879));
#39689=CARTESIAN_POINT('Ctrl Pts',(-0.00313194163772321,-0.025289419352234,
-0.0139434841362084));
#39690=CARTESIAN_POINT('Ctrl Pts',(-0.00319550174896822,-0.025131783803256,
-0.0105259020768301));
#39691=CARTESIAN_POINT('Ctrl Pts',(-0.000372315933265614,-0.0249741482542779,
-0.00859884955669905));
#39692=CARTESIAN_POINT('Ctrl Pts',(0.00278721283092204,-0.0248165127052998,
-0.00990318551528194));
#39693=CARTESIAN_POINT('Ctrl Pts',(0.00342883321548304,-0.0246588771563218,
-0.0132606003240156));
#39694=CARTESIAN_POINT('Ctrl Pts',(0.00097291979816731,-0.0245012416073438,
-0.0156380781585438));
#39695=CARTESIAN_POINT('Ctrl Pts',(-0.00236190849724789,-0.0243436060583657,
-0.0148878566236573));
#39696=CARTESIAN_POINT('Ctrl Pts',(-0.00356303951920687,-0.0241859705093877,
-0.0116876697707944));
#39697=CARTESIAN_POINT('Ctrl Pts',(-0.00154539748107324,-0.0240283349604096,
-0.00892849736567574));
#39698=CARTESIAN_POINT('Ctrl Pts',(0.00186832334048244,-0.0238706994114316,
-0.00910291630068922));
#39699=CARTESIAN_POINT('Ctrl Pts',(0.003594241126128,-0.0237130638624535,
-0.0120533602574297));
#39700=CARTESIAN_POINT('Ctrl Pts',(0.00207319896783111,-0.0235554283134755,
-0.0151144617782086));
#39701=CARTESIAN_POINT('Ctrl Pts',(-0.00132072644568367,-0.0233977927644975,
-0.0155208877375533));
#39702=CARTESIAN_POINT('Ctrl Pts',(-0.00352153605955123,-0.0232401572155194,
-0.0129054816873811));
#39703=CARTESIAN_POINT('Ctrl Pts',(-0.00254106591574783,-0.0230825216665414,
-0.0096309450690597));
#39704=CARTESIAN_POINT('Ctrl Pts',(0.000734948395842858,-0.0229248861175633,
-0.00865542367096509));
#39705=CARTESIAN_POINT('Ctrl Pts',(0.00334702617063905,-0.0227672505685853,
-0.0108601824934037));
#39706=CARTESIAN_POINT('Ctrl Pts',(0.00293547265879514,-0.0226096150196073,
-0.0142534899469383));
#39707=CARTESIAN_POINT('Ctrl Pts',(-0.000127923569543504,-0.0224519794706292,
-0.0157699052315523));
#39708=CARTESIAN_POINT('Ctrl Pts',(-0.00307575640295856,-0.0222943439216512,
-0.014039531470352));
#39709=CARTESIAN_POINT('Ctrl Pts',(-0.00324501720966393,-0.0221367083726731,
-0.0106255510154228));
#39710=CARTESIAN_POINT('Ctrl Pts',(-0.000482799425948263,-0.0219790728236951,
-0.0086120802105612));
#39711=CARTESIAN_POINT('Ctrl Pts',(0.00271556895104147,-0.021821437274717,
-0.00981804517396586));
#39712=CARTESIAN_POINT('Ctrl Pts',(0.00346075088011901,-0.021663801725739,
-0.0131540031563442));
#39713=CARTESIAN_POINT('Ctrl Pts',(0.00107956507222703,-0.0215061661767609,
-0.0156063216332275));
#39714=CARTESIAN_POINT('Ctrl Pts',(-0.00227687654957576,-0.0213485306277829,
-0.014959628960963));
#39715=CARTESIAN_POINT('Ctrl Pts',(-0.00357643697965559,-0.0211908950788049,
-0.0117981333566007));
#39716=CARTESIAN_POINT('Ctrl Pts',(-0.00164512134804076,-0.0210332595298268,
-0.00897786179596077));
#39717=CARTESIAN_POINT('Ctrl Pts',(0.0017723614516327,-0.0208756239808488,
-0.00904658680123543));
#39718=CARTESIAN_POINT('Ctrl Pts',(0.00358873110925933,-0.0207179884318707,
-0.011942223695265));
#39719=CARTESIAN_POINT('Ctrl Pts',(0.00216311847927169,-0.0205603528828927,
-0.0150489165114876));
#39720=CARTESIAN_POINT('Ctrl Pts',(-0.0012166088095401,-0.0204027173339146,
-0.0155601459752024));
#39721=CARTESIAN_POINT('Ctrl Pts',(-0.003497277816922,-0.0202450817849366,
-0.0130140783316013));
#39722=CARTESIAN_POINT('Ctrl Pts',(-0.00261858165263156,-0.0200874462359586,
-0.0097107763522708));
#39723=CARTESIAN_POINT('Ctrl Pts',(0.000625685134828339,-0.0199298106869805,
-0.00863437154163214));
#39724=CARTESIAN_POINT('Ctrl Pts',(0.00330472067115259,-0.0197721751380025,
-0.0107572653591462));
#39725=CARTESIAN_POINT('Ctrl Pts',(0.00299834431493395,-0.0196145395890244,
-0.014161680220569));
#39726=CARTESIAN_POINT('Ctrl Pts',(-1.6674577032454E-5,-0.0194569040400464,
-0.0157721432019016));
#39727=CARTESIAN_POINT('Ctrl Pts',(-0.00301662439656255,-0.0192992684910683,
-0.0141337927842166));
#39728=CARTESIAN_POINT('Ctrl Pts',(-0.00329143158006377,-0.0191416329420903,
-0.0107266870729041));
#39729=CARTESIAN_POINT('Ctrl Pts',(-0.00059280963165573,-0.0189839973931122,
-0.00862871718285146));
#39730=CARTESIAN_POINT('Ctrl Pts',(0.00264130373978803,-0.0188263618441342,
-0.00973517223149046));
#39731=CARTESIAN_POINT('Ctrl Pts',(0.00348939724868163,-0.0186687262951562,
-0.013046450041716));
#39732=CARTESIAN_POINT('Ctrl Pts',(0.00118509637283412,-0.0185110907461781,
-0.0155713185576321));
#39733=CARTESIAN_POINT('Ctrl Pts',(-0.00218951000492656,-0.0183534551972001,
-0.0150286641021081));
#39734=CARTESIAN_POINT('Ctrl Pts',(-0.00358670864122049,-0.018195819648222,
-0.0119090974795379));
#39735=CARTESIAN_POINT('Ctrl Pts',(-0.00174269656258942,-0.018038184099244,
-0.00903002020530739));
#39736=CARTESIAN_POINT('Ctrl Pts',(0.00167359605724419,-0.0178805485502659,
-0.00899377017639597));
#39737=CARTESIAN_POINT('Ctrl Pts',(0.00358194225358649,-0.0177229130012879,
-0.0118302936733849));
#39738=CARTESIAN_POINT('Ctrl Pts',(0.0022464705553738,-0.0175652666528983,
-0.0149830002760419));
#39739=CARTESIAN_POINT('Ctrl Pts',(1.47162903616745E-5,-0.0174601654875016,
-0.0153878269104618));
#39740=CARTESIAN_POINT('Ctrl Pts',(-0.000943092295784545,-0.0174076095050974,
-0.0150763837366195));
#39741=CARTESIAN_POINT('Ctrl Pts',(0.000690033766136825,-0.0273898599693712,
-0.0149570904152181));
#39742=CARTESIAN_POINT('Ctrl Pts',(-0.000228370153920869,-0.0273373047286097,
-0.0151849636833654));
#39743=CARTESIAN_POINT('Ctrl Pts',(-0.00229279313382739,-0.0272322043048555,
-0.0146564994654789));
#39744=CARTESIAN_POINT('Ctrl Pts',(-0.00333373464596939,-0.0270745586981087,
-0.0116127497404478));
#39745=CARTESIAN_POINT('Ctrl Pts',(-0.00135585737110244,-0.0269169231491307,
-0.00908197341579252));
#39746=CARTESIAN_POINT('Ctrl Pts',(0.00184329963115394,-0.0267592876001526,
-0.00934414263668327));
#39747=CARTESIAN_POINT('Ctrl Pts',(0.00337910219330849,-0.0266016520511746,
-0.0121654438591319));
#39748=CARTESIAN_POINT('Ctrl Pts',(0.00186134043567162,-0.0264440165021965,
-0.0149956170644823));
#39749=CARTESIAN_POINT('Ctrl Pts',(-0.00133741929073781,-0.0262863809532184,
-0.0152787526493183));
#39750=CARTESIAN_POINT('Ctrl Pts',(-0.00332824148826644,-0.0261287454042405,
-0.0127586523085022));
#39751=CARTESIAN_POINT('Ctrl Pts',(-0.00231226786314605,-0.0259711098552624,
-0.00971213849660252));
#39752=CARTESIAN_POINT('Ctrl Pts',(0.000792488943208649,-0.0258134743062844,
-0.00889125273834406));
#39753=CARTESIAN_POINT('Ctrl Pts',(0.00318136458011873,-0.0256558387573063,
-0.011037624458525));
#39754=CARTESIAN_POINT('Ctrl Pts',(0.00269624519487149,-0.0254982032083283,
-0.0142122370889994));
#39755=CARTESIAN_POINT('Ctrl Pts',(-0.00022459417844039,-0.0253405676593502,
-0.0155472299374572));
#39756=CARTESIAN_POINT('Ctrl Pts',(-0.00294254510371564,-0.0251829321103721,
-0.0138365909705451));
#39757=CARTESIAN_POINT('Ctrl Pts',(-0.00300226157221008,-0.0250252965613941,
-0.0106256788532042));
#39758=CARTESIAN_POINT('Ctrl Pts',(-0.000349801035009846,-0.024867661012416,
-0.00881516013554496));
#39759=CARTESIAN_POINT('Ctrl Pts',(0.00261866293096226,-0.024710025463438,
-0.0100406195573617));
#39760=CARTESIAN_POINT('Ctrl Pts',(0.00322148288721361,-0.02455238991446,
-0.0131950028918365));
#39761=CARTESIAN_POINT('Ctrl Pts',(0.000914084845618756,-0.024394754365482,
-0.0154287085512653));
#39762=CARTESIAN_POINT('Ctrl Pts',(-0.00221907783985831,-0.0242371188165039,
-0.0147238548344551));
#39763=CARTESIAN_POINT('Ctrl Pts',(-0.00334757339195157,-0.0240794832675258,
-0.0117171914785847));
#39764=CARTESIAN_POINT('Ctrl Pts',(-0.00145194333650873,-0.0239218477185478,
-0.00912487329704566));
#39765=CARTESIAN_POINT('Ctrl Pts',(0.00175534104195211,-0.0237642121695698,
-0.00928874467224547));
#39766=CARTESIAN_POINT('Ctrl Pts',(0.00337688815777223,-0.0236065766205917,
-0.0120607677246945));
#39767=CARTESIAN_POINT('Ctrl Pts',(0.00194782731527988,-0.0234489410716137,
-0.0149367565948105));
#39768=CARTESIAN_POINT('Ctrl Pts',(-0.00124085873417469,-0.0232913055226356,
-0.0153186049352418));
#39769=CARTESIAN_POINT('Ctrl Pts',(-0.00330857975282177,-0.0231336699736576,
-0.0128613591888756));
#39770=CARTESIAN_POINT('Ctrl Pts',(-0.00238740115030942,-0.0229760344246795,
-0.00978484218832786));
#39771=CARTESIAN_POINT('Ctrl Pts',(0.00069050418361027,-0.0228183988757015,
-0.00886831306819399));
#39772=CARTESIAN_POINT('Ctrl Pts',(0.00314462292393853,-0.0226607633267235,
-0.0109397444766531));
#39773=CARTESIAN_POINT('Ctrl Pts',(0.00275795710724289,-0.0225031277777454,
-0.0141278499357506));
#39774=CARTESIAN_POINT('Ctrl Pts',(-0.000120187703588163,-0.0223454922287674,
-0.0155525637034643));
#39775=CARTESIAN_POINT('Ctrl Pts',(-0.00288975753402832,-0.0221878566797893,
-0.0139268300763462));
#39776=CARTESIAN_POINT('Ctrl Pts',(-0.00304878270615251,-0.0220302211308113,
-0.0107193017652071));
#39777=CARTESIAN_POINT('Ctrl Pts',(-0.0004536033078616,-0.0218725855818332,
-0.00882759069787478));
#39778=CARTESIAN_POINT('Ctrl Pts',(0.00255135154003003,-0.0217149500328552,
-0.00996062787059126));
#39779=CARTESIAN_POINT('Ctrl Pts',(0.00325147040890474,-0.0215573144838771,
-0.0130948519279668));
#39780=CARTESIAN_POINT('Ctrl Pts',(0.00101428100676018,-0.0213996789348991,
-0.0153988724243863));
#39781=CARTESIAN_POINT('Ctrl Pts',(-0.00213918799189042,-0.0212420433859211,
-0.0147912869146629));
#39782=CARTESIAN_POINT('Ctrl Pts',(-0.00336016067364632,-0.021084407836943,
-0.01182097504838));
#39783=CARTESIAN_POINT('Ctrl Pts',(-0.00154563664577557,-0.020926772287965,
-0.00917125253377325));
#39784=CARTESIAN_POINT('Ctrl Pts',(0.00166518221434912,-0.0207691367389869,
-0.00923582156192436));
#39785=CARTESIAN_POINT('Ctrl Pts',(0.00337171134573875,-0.0206115011900089,
-0.0119563518751454));
#39786=CARTESIAN_POINT('Ctrl Pts',(0.00203230916351456,-0.0204538656410308,
-0.014875175018277));
#39787=CARTESIAN_POINT('Ctrl Pts',(-0.00114303735820951,-0.0202962300920528,
-0.0153554891266914));
#39788=CARTESIAN_POINT('Ctrl Pts',(-0.00328578846826729,-0.0201385945430748,
-0.0129633887158252));
#39789=CARTESIAN_POINT('Ctrl Pts',(-0.00246022931200976,-0.0199809589940967,
-0.00985984586933738));
#39790=CARTESIAN_POINT('Ctrl Pts',(0.000587848351891767,-0.0198233234451187,
-0.00884853401505157));
#39791=CARTESIAN_POINT('Ctrl Pts',(0.0031048757463811,-0.0196656878961406,
-0.0108430510051495));
#39792=CARTESIAN_POINT('Ctrl Pts',(0.00281702675327508,-0.0195080523471626,
-0.014041592178726));
#39793=CARTESIAN_POINT('Ctrl Pts',(-1.56662226436196E-5,-0.0193504167981845,
-0.0155546663380134));
#39794=CARTESIAN_POINT('Ctrl Pts',(-0.00283420139153906,-0.0191927812492065,
-0.0140153911670897));
#39795=CARTESIAN_POINT('Ctrl Pts',(-0.0030923902806734,-0.0190351457002284,
-0.0108143218662095));
#39796=CARTESIAN_POINT('Ctrl Pts',(-0.000556960914614001,-0.0188775101512504,
-0.00884322158983128));
#39797=CARTESIAN_POINT('Ctrl Pts',(0.00248157733634815,-0.0187198746022724,
-0.0098827664672451));
#39798=CARTESIAN_POINT('Ctrl Pts',(0.00327838445817626,-0.0185622390532943,
-0.0129938028257018));
#39799=CARTESIAN_POINT('Ctrl Pts',(0.00111343055927733,-0.0184046035043163,
-0.0153659860744406));
#39800=CARTESIAN_POINT('Ctrl Pts',(-0.00205710472600525,-0.0182469679553382,
-0.0148561473239737));
#39801=CARTESIAN_POINT('Ctrl Pts',(-0.00336981118152323,-0.0180893324063602,
-0.0119252288865435));
#39802=CARTESIAN_POINT('Ctrl Pts',(-0.00163731123713958,-0.0179316968573822,
-0.00922025679049115));
#39803=CARTESIAN_POINT('Ctrl Pts',(0.0015723894163691,-0.0177740613084041,
-0.00918619889369064));
#39804=CARTESIAN_POINT('Ctrl Pts',(0.00336533302955961,-0.017616425759426,
-0.0118511905484224));
#39805=CARTESIAN_POINT('Ctrl Pts',(0.00211062072604963,-0.0174587794110365,
-0.0148132449064481));
#39806=CARTESIAN_POINT('Ctrl Pts',(1.38263585844006E-5,-0.0173536782456397,
-0.01519359063723));
#39807=CARTESIAN_POINT('Ctrl Pts',(-0.000886061088714966,-0.0173011222632356,
-0.0149009812299417));
#39808=CARTESIAN_POINT('Ctrl Pts',(0.000645619832263892,-0.0272833727275095,
-0.0147780764481064));
#39809=CARTESIAN_POINT('Ctrl Pts',(-0.0002136711385791,-0.0272308174867479,
-0.0149912826829002));
#39810=CARTESIAN_POINT('Ctrl Pts',(-0.002145217801101,-0.0271257170629937,
-0.014496832995866));
#39811=CARTESIAN_POINT('Ctrl Pts',(-0.0031191592478046,-0.026968071456247,
-0.0116489938271691));
#39812=CARTESIAN_POINT('Ctrl Pts',(-0.00126858778724075,-0.0268104359072689,
-0.00928111059245599));
#39813=CARTESIAN_POINT('Ctrl Pts',(0.00172465588943622,-0.0266528003582908,
-0.00952640532544256));
#39814=CARTESIAN_POINT('Ctrl Pts',(0.00316160671884255,-0.0264951648093128,
-0.0121661138605784));
#39815=CARTESIAN_POINT('Ctrl Pts',(0.00174153549991065,-0.0263375292603347,
-0.0148141233345868));
#39816=CARTESIAN_POINT('Ctrl Pts',(-0.00125133647152775,-0.0261798937113568,
-0.0150790349342222));
#39817=CARTESIAN_POINT('Ctrl Pts',(-0.00311401965648484,-0.0260222581623787,
-0.0127211405250328));
#39818=CARTESIAN_POINT('Ctrl Pts',(-0.00216343904199254,-0.0258646226134007,
-0.00987071517956028));
#39819=CARTESIAN_POINT('Ctrl Pts',(0.00074148049515003,-0.0257069870644226,
-0.0091026656266786));
#39820=CARTESIAN_POINT('Ctrl Pts',(0.00297659646148286,-0.0255493515154446,
-0.0111108864094343));
#39821=CARTESIAN_POINT('Ctrl Pts',(0.00252270172255615,-0.0253917159664665,
-0.0140811655096361));
#39822=CARTESIAN_POINT('Ctrl Pts',(-0.000210138203270753,-0.0252340804174884,
-0.0153302317165266));
#39823=CARTESIAN_POINT('Ctrl Pts',(-0.00275314856970804,-0.0250764448685105,
-0.0137296978048819));
#39824=CARTESIAN_POINT('Ctrl Pts',(-0.00280902139545195,-0.0249188093195324,
-0.0107254556295784));
#39825=CARTESIAN_POINT('Ctrl Pts',(-0.000327286136754079,-0.0247611737705544,
-0.00903147071439088));
#39826=CARTESIAN_POINT('Ctrl Pts',(0.0024501130310025,-0.0246035382215763,
-0.0101780535994417));
#39827=CARTESIAN_POINT('Ctrl Pts',(0.00301413255894418,-0.0244459026725983,
-0.0131294054596574));
#39828=CARTESIAN_POINT('Ctrl Pts',(0.000855249893070201,-0.0242882671236202,
-0.0152193389439868));
#39829=CARTESIAN_POINT('Ctrl Pts',(-0.00207624718246873,-0.0241306315746422,
-0.0145598530452527));
#39830=CARTESIAN_POINT('Ctrl Pts',(-0.00313210726469626,-0.0239729960256641,
-0.011746713186375));
#39831=CARTESIAN_POINT('Ctrl Pts',(-0.00135848919194423,-0.0238153604766861,
-0.00932124922841558));
#39832=CARTESIAN_POINT('Ctrl Pts',(0.00164235874342176,-0.0236577249277079,
-0.00947457304380171));
#39833=CARTESIAN_POINT('Ctrl Pts',(0.00315953518941646,-0.02350008937873,
-0.0120681751919595));
#39834=CARTESIAN_POINT('Ctrl Pts',(0.00182245566272866,-0.0233424538297518,
-0.0147590514114124));
#39835=CARTESIAN_POINT('Ctrl Pts',(-0.00116099102266572,-0.0231848182807739,
-0.0151163221329304));
#39836=CARTESIAN_POINT('Ctrl Pts',(-0.0030956234460923,-0.0230271827317957,
-0.0128172366903702));
#39837=CARTESIAN_POINT('Ctrl Pts',(-0.00223373638487103,-0.0228695471828178,
-0.00993873930759601));
#39838=CARTESIAN_POINT('Ctrl Pts',(0.000646059971377684,-0.0227119116338398,
-0.00908120246542289));
#39839=CARTESIAN_POINT('Ctrl Pts',(0.00294221967723799,-0.0225542760848617,
-0.0110193064599024));
#39840=CARTESIAN_POINT('Ctrl Pts',(0.00258044155569065,-0.0223966405358837,
-0.0140022099245627));
#39841=CARTESIAN_POINT('Ctrl Pts',(-0.000112451837632818,-0.0222390049869056,
-0.0153352221753762));
#39842=CARTESIAN_POINT('Ctrl Pts',(-0.0027037586650981,-0.0220813694379276,
-0.0138141286823404));
#39843=CARTESIAN_POINT('Ctrl Pts',(-0.00285254820264108,-0.0219237338889494,
-0.0108130525149913));
#39844=CARTESIAN_POINT('Ctrl Pts',(-0.000424407189774945,-0.0217660983399715,
-0.00904310118518834));
#39845=CARTESIAN_POINT('Ctrl Pts',(0.00238713412901858,-0.0216084627909933,
-0.0101032105672167));
#39846=CARTESIAN_POINT('Ctrl Pts',(0.00304218993769049,-0.0214508272420154,
-0.0130357006995895));
#39847=CARTESIAN_POINT('Ctrl Pts',(0.000948996941293319,-0.0212931916930374,
-0.0151914232155454));
#39848=CARTESIAN_POINT('Ctrl Pts',(-0.00200149943420506,-0.0211355561440593,
-0.0146229448683627));
#39849=CARTESIAN_POINT('Ctrl Pts',(-0.00314388436763707,-0.0209779205950813,
-0.0118438167401592));
#39850=CARTESIAN_POINT('Ctrl Pts',(-0.00144615194351038,-0.0208202850461031,
-0.00936464327158571));
#39851=CARTESIAN_POINT('Ctrl Pts',(0.00155800297706554,-0.0206626494971252,
-0.0094250563226133));
#39852=CARTESIAN_POINT('Ctrl Pts',(0.00315469158221817,-0.020505013948147,
-0.0119704800550257));
#39853=CARTESIAN_POINT('Ctrl Pts',(0.00190149984775741,-0.0203473783991691,
-0.0147014335250665));
#39854=CARTESIAN_POINT('Ctrl Pts',(-0.00106946590687894,-0.020189742850191,
-0.0151508322781805));
#39855=CARTESIAN_POINT('Ctrl Pts',(-0.00307429911961257,-0.020032107301213,
-0.0129126991000491));
#39856=CARTESIAN_POINT('Ctrl Pts',(-0.00230187697138798,-0.019874471752235,
-0.0100089153864039));
#39857=CARTESIAN_POINT('Ctrl Pts',(0.000550011568955204,-0.0197168362032569,
-0.00906269648847102));
#39858=CARTESIAN_POINT('Ctrl Pts',(0.00290503082160958,-0.0195592006542789,
-0.0109288366511528));
#39859=CARTESIAN_POINT('Ctrl Pts',(0.0026357091916162,-0.0194015651053008,
-0.0139215041368831));
#39860=CARTESIAN_POINT('Ctrl Pts',(-1.46578682547907E-5,-0.0192439295563228,
-0.0153371894741254));
#39861=CARTESIAN_POINT('Ctrl Pts',(-0.00265177838651556,-0.0190862940073448,
-0.0138969895499631));
#39862=CARTESIAN_POINT('Ctrl Pts',(-0.00289334898128302,-0.0189286584583667,
-0.0109019566595151));
#39863=CARTESIAN_POINT('Ctrl Pts',(-0.000521112197572276,-0.0187710229093887,
-0.00905772599681111));
#39864=CARTESIAN_POINT('Ctrl Pts',(0.00232185093290827,-0.0186133873604106,
-0.0100303607029996));
#39865=CARTESIAN_POINT('Ctrl Pts',(0.00306737166767089,-0.0184557518114326,
-0.0129411556096876));
#39866=CARTESIAN_POINT('Ctrl Pts',(0.00104176474572055,-0.0182981162624545,
-0.0151606535912491));
#39867=CARTESIAN_POINT('Ctrl Pts',(-0.00192469944708394,-0.0181404807134765,
-0.0146836305458396));
#39868=CARTESIAN_POINT('Ctrl Pts',(-0.00315291372182597,-0.0179828451644985,
-0.0119413602935491));
#39869=CARTESIAN_POINT('Ctrl Pts',(-0.00153192591168972,-0.0178252096155204,
-0.0094104933756749));
#39870=CARTESIAN_POINT('Ctrl Pts',(0.001471182775494,-0.0176675740665424,
-0.00937862761098531));
#39871=CARTESIAN_POINT('Ctrl Pts',(0.00314872380553277,-0.0175099385175643,
-0.0118720874234598));
#39872=CARTESIAN_POINT('Ctrl Pts',(0.00197477089672548,-0.0173522921691749,
-0.0146434895368542));
#39873=CARTESIAN_POINT('Ctrl Pts',(1.29364268071242E-5,-0.017247191003778,
-0.014999354363998));
#39874=CARTESIAN_POINT('Ctrl Pts',(-0.000829029881645386,-0.0171946350213738,
-0.0147255787232639));
#39875=CARTESIAN_POINT('Ctrl Pts',(0.000601205898390958,-0.0271768854856476,
-0.0145990624809945));
#39876=CARTESIAN_POINT('Ctrl Pts',(-0.000198972123237332,-0.0271243302448861,
-0.0147976016824351));
#39877=CARTESIAN_POINT('Ctrl Pts',(-0.00199764246837458,-0.027019229821132,
-0.0143371665262532));
#39878=CARTESIAN_POINT('Ctrl Pts',(-0.00290458384963981,-0.0268615842143851,
-0.0116852379138905));
#39879=CARTESIAN_POINT('Ctrl Pts',(-0.00118131820337908,-0.026703948665407,
-0.00948024776911945));
#39880=CARTESIAN_POINT('Ctrl Pts',(0.00160601214771848,-0.026546313116429,
-0.00970866801420186));
#39881=CARTESIAN_POINT('Ctrl Pts',(0.0029441112443766,-0.026388677567451,
-0.0121667838620248));
#39882=CARTESIAN_POINT('Ctrl Pts',(0.00162173056414967,-0.0262310420184729,
-0.0146326296046914));
#39883=CARTESIAN_POINT('Ctrl Pts',(-0.00116525365231769,-0.0260734064694949,
-0.0148793172191262));
#39884=CARTESIAN_POINT('Ctrl Pts',(-0.00289979782470325,-0.0259157709205169,
-0.0126836287415636));
#39885=CARTESIAN_POINT('Ctrl Pts',(-0.00201461022083903,-0.0257581353715388,
-0.010029291862518));
#39886=CARTESIAN_POINT('Ctrl Pts',(0.000690472047091409,-0.0256004998225608,
-0.00931407851501315));
#39887=CARTESIAN_POINT('Ctrl Pts',(0.00277182834284702,-0.0254428642735827,
-0.0111841483603438));
#39888=CARTESIAN_POINT('Ctrl Pts',(0.00234915825024082,-0.0252852287246047,
-0.013950093930273));
#39889=CARTESIAN_POINT('Ctrl Pts',(-0.000195682228101112,-0.0251275931756266,
-0.015113233495596));
#39890=CARTESIAN_POINT('Ctrl Pts',(-0.00256375203570046,-0.0249699576266486,
-0.0136228046392186));
#39891=CARTESIAN_POINT('Ctrl Pts',(-0.00261578121869382,-0.0248123220776705,
-0.0108252324059526));
#39892=CARTESIAN_POINT('Ctrl Pts',(-0.000304771238498309,-0.0246546865286925,
-0.00924778129323679));
#39893=CARTESIAN_POINT('Ctrl Pts',(0.00228156313104271,-0.0244970509797144,
-0.0103154876415214));
#39894=CARTESIAN_POINT('Ctrl Pts',(0.00280678223067475,-0.0243394154307364,
-0.0130638080274784));
#39895=CARTESIAN_POINT('Ctrl Pts',(0.000796414940521645,-0.0241817798817584,
-0.0150099693367085));
#39896=CARTESIAN_POINT('Ctrl Pts',(-0.00193341652507914,-0.0240241443327803,
-0.0143958512560506));
#39897=CARTESIAN_POINT('Ctrl Pts',(-0.00291664113744096,-0.0238665087838023,
-0.0117762348941654));
#39898=CARTESIAN_POINT('Ctrl Pts',(-0.00126503504737973,-0.0237088732348243,
-0.0095176251597855));
#39899=CARTESIAN_POINT('Ctrl Pts',(0.00152937644489143,-0.0235512376858462,
-0.00966040141535797));
#39900=CARTESIAN_POINT('Ctrl Pts',(0.00294218222106068,-0.0233936021368682,
-0.0120755826592244));
#39901=CARTESIAN_POINT('Ctrl Pts',(0.00169708401017743,-0.0232359665878901,
-0.0145813462280142));
#39902=CARTESIAN_POINT('Ctrl Pts',(-0.00108112331115675,-0.0230783310389121,
-0.0149140393306191));
#39903=CARTESIAN_POINT('Ctrl Pts',(-0.00288266713936284,-0.022920695489934,
-0.0127731141918649));
#39904=CARTESIAN_POINT('Ctrl Pts',(-0.00208007161943263,-0.022763059940956,
-0.0100926364268643));
#39905=CARTESIAN_POINT('Ctrl Pts',(0.000601615759145098,-0.0226054243919779,
-0.00929409186265181));
#39906=CARTESIAN_POINT('Ctrl Pts',(0.00273981643053748,-0.0224477888429999,
-0.0110988684431518));
#39907=CARTESIAN_POINT('Ctrl Pts',(0.00240292600413841,-0.0222901532940218,
-0.0138765699133749));
#39908=CARTESIAN_POINT('Ctrl Pts',(-0.000104715971677476,-0.0221325177450438,
-0.0151178806472884));
#39909=CARTESIAN_POINT('Ctrl Pts',(-0.00251775979616787,-0.0219748821960658,
-0.0137014272883347));
#39910=CARTESIAN_POINT('Ctrl Pts',(-0.00265631369912967,-0.0218172466470877,
-0.0109068032647757));
#39911=CARTESIAN_POINT('Ctrl Pts',(-0.000395211071688283,-0.0216596110981097,
-0.0092586116725019));
#39912=CARTESIAN_POINT('Ctrl Pts',(0.00222291671800713,-0.0215019755491316,
-0.0102457932638421));
#39913=CARTESIAN_POINT('Ctrl Pts',(0.00283290946647623,-0.0213443400001536,
-0.0129765494712121));
#39914=CARTESIAN_POINT('Ctrl Pts',(0.000883712875826465,-0.0211867044511755,
-0.0149839740067044));
#39915=CARTESIAN_POINT('Ctrl Pts',(-0.00186381087651972,-0.0210290689021975,
-0.0144546028220626));
#39916=CARTESIAN_POINT('Ctrl Pts',(-0.00292760806162782,-0.0208714333532195,
-0.0118666584319385));
#39917=CARTESIAN_POINT('Ctrl Pts',(-0.00134666724124519,-0.0207137978042414,
-0.00955803400939818));
#39918=CARTESIAN_POINT('Ctrl Pts',(0.00145082373978195,-0.0205561622552634,
-0.00961429108330222));
#39919=CARTESIAN_POINT('Ctrl Pts',(0.00293767181869759,-0.0203985267062853,
-0.0119846082349061));
#39920=CARTESIAN_POINT('Ctrl Pts',(0.00177069053200028,-0.0202408911573073,
-0.0145276920318559));
#39921=CARTESIAN_POINT('Ctrl Pts',(-0.000995894455548362,-0.0200832556083292,
-0.0149461754296697));
#39922=CARTESIAN_POINT('Ctrl Pts',(-0.00286280977095785,-0.0199256200593512,
-0.0128620094842728));
#39923=CARTESIAN_POINT('Ctrl Pts',(-0.00214352463076619,-0.0197679845103731,
-0.0101579849034705));
#39924=CARTESIAN_POINT('Ctrl Pts',(0.000512174786018637,-0.0196103489613951,
-0.00927685896189047));
#39925=CARTESIAN_POINT('Ctrl Pts',(0.00270518589683808,-0.019452713412417,
-0.0110146222971561));
#39926=CARTESIAN_POINT('Ctrl Pts',(0.00245439162995732,-0.019295077863439,
-0.0138014160950401));
#39927=CARTESIAN_POINT('Ctrl Pts',(-1.3649513865962E-5,-0.019137442314461,
-0.0151197126102372));
#39928=CARTESIAN_POINT('Ctrl Pts',(-0.00246935538149206,-0.0189798067654829,
-0.0137785879328362));
#39929=CARTESIAN_POINT('Ctrl Pts',(-0.00269430768189265,-0.0188221712165049,
-0.0109895914528207));
#39930=CARTESIAN_POINT('Ctrl Pts',(-0.000485263480530543,-0.0186645356675268,
-0.00927223040379092));
#39931=CARTESIAN_POINT('Ctrl Pts',(0.0021621245294684,-0.0185069001185488,
-0.0101779549387543));
#39932=CARTESIAN_POINT('Ctrl Pts',(0.00285635887716552,-0.0183492645695708,
-0.0128885083936734));
#39933=CARTESIAN_POINT('Ctrl Pts',(0.000970098932163777,-0.0181916290205927,
-0.0149553211080576));
#39934=CARTESIAN_POINT('Ctrl Pts',(-0.00179229416816263,-0.0180339934716147,
-0.0145111137677053));
#39935=CARTESIAN_POINT('Ctrl Pts',(-0.0029360162621287,-0.0178763579226366,
-0.0119574917005547));
#39936=CARTESIAN_POINT('Ctrl Pts',(-0.00142654058623987,-0.0177187223736586,
-0.00960072996085867));
#39937=CARTESIAN_POINT('Ctrl Pts',(0.00136997613461892,-0.0175610868246805,
-0.00957105632827997));
#39938=CARTESIAN_POINT('Ctrl Pts',(0.00293211458150592,-0.0174034512757025,
-0.0118929842984973));
#39939=CARTESIAN_POINT('Ctrl Pts',(0.0018389210674013,-0.017245804927313,
-0.0144737341672604));
#39940=CARTESIAN_POINT('Ctrl Pts',(1.20464950298498E-5,-0.0171407037619162,
-0.0148051180907662));
#39941=CARTESIAN_POINT('Ctrl Pts',(-0.000771998674575806,-0.017088147779512,
-0.0145501762165862));
#39942=CARTESIAN_POINT('Ctrl Pts',(-0.00300179803210124,-0.0271787743899901,
-0.0121753188445143));
#39943=CARTESIAN_POINT('Ctrl Pts',(-0.00299170500774972,-0.0271787744029572,
-0.012274001554098));
#39944=CARTESIAN_POINT('Ctrl Pts',(-0.00297664702496829,-0.0271787743898748,
-0.0123720503346277));
#39945=CARTESIAN_POINT('Ctrl Pts',(-0.00295682936558202,-0.0271787743898749,
-0.0124691137840994));
#39946=CARTESIAN_POINT('Ctrl Pts',(-0.00290457240419616,-0.0271787743898752,
-0.0127250592937154));
#39947=CARTESIAN_POINT('Ctrl Pts',(-0.00281935579375609,-0.0271787743898754,
-0.012974265349726));
#39948=CARTESIAN_POINT('Ctrl Pts',(-0.00270343235514401,-0.0271787743898756,
-0.0132095505979502));
#39949=CARTESIAN_POINT('Ctrl Pts',(-0.00269512702070926,-0.0271787743898756,
-0.0132264076089004));
#39950=CARTESIAN_POINT('Ctrl Pts',(-0.00268666329850635,-0.0271787743898756,
-0.0132431924273196));
#39951=CARTESIAN_POINT('Ctrl Pts',(-0.00267804168256273,-0.0271787743898756,
-0.0132599020323125));
#39952=CARTESIAN_POINT('Ctrl Pts',(-0.00267151568645102,-0.0271787743898757,
-0.0132725501040805));
#39953=CARTESIAN_POINT('Ctrl Pts',(-0.00266490146409413,-0.0271787743898756,
-0.0132851506618195));
#39954=CARTESIAN_POINT('Ctrl Pts',(-0.00265820309333032,-0.0271787743898756,
-0.0132976957827427));
#39955=CARTESIAN_POINT('Ctrl Pts',(-0.00249348720410649,-0.0271787743898759,
-0.0136061858351965));
#39956=CARTESIAN_POINT('Ctrl Pts',(-0.00227771368615723,-0.0271787743898759,
-0.0138830139207218));
#39957=CARTESIAN_POINT('Ctrl Pts',(-0.00201563806114113,-0.0271787743898759,
-0.0141093884962233));
#39958=CARTESIAN_POINT('Ctrl Pts',(-0.00200231890338116,-0.0271787743898759,
-0.014120893262009));
#39959=CARTESIAN_POINT('Ctrl Pts',(-0.00198887690751847,-0.0271787743898759,
-0.0141322675641596));
#39960=CARTESIAN_POINT('Ctrl Pts',(-0.00197533127033276,-0.0271787743898759,
-0.0141434930754665));
#39961=CARTESIAN_POINT('Ctrl Pts',(-0.00194648600772747,-0.0271787743898759,
-0.0141673976594359));
#39962=CARTESIAN_POINT('Ctrl Pts',(-0.0019171536737065,-0.0271787743898759,
-0.014190642780961));
#39963=CARTESIAN_POINT('Ctrl Pts',(-0.00188734151124788,-0.0271787743898759,
-0.0142132063515489));
#39964=CARTESIAN_POINT('Ctrl Pts',(-0.00166838124506507,-0.0271787743898758,
-0.0143789281581709));
#39965=CARTESIAN_POINT('Ctrl Pts',(-0.00142362040013632,-0.0271787743898756,
-0.014508195233492));
#39966=CARTESIAN_POINT('Ctrl Pts',(-0.00116282079016005,-0.0271787743898753,
-0.0145991360864556));
#39967=CARTESIAN_POINT('Ctrl Pts',(-0.00114190913175246,-0.0271787743898753,
-0.0146064279840648));
#39968=CARTESIAN_POINT('Ctrl Pts',(-0.00112089415409831,-0.0271787743898753,
-0.0146134714313065));
#39969=CARTESIAN_POINT('Ctrl Pts',(-0.00109978090207821,-0.0271787743898752,
-0.0146202643895321));
#39970=CARTESIAN_POINT('Ctrl Pts',(-0.00108278352153522,-0.0271787743898752,
-0.014625733111066));
#39971=CARTESIAN_POINT('Ctrl Pts',(-0.00106571994357321,-0.0271787743898752,
-0.0146310401292033));
#39972=CARTESIAN_POINT('Ctrl Pts',(-0.00104861536807709,-0.0271787743898752,
-0.0146361778513352));
#39973=CARTESIAN_POINT('Ctrl Pts',(-0.000873308221192212,-0.0271787743898749,
-0.0146888350721259));
#39974=CARTESIAN_POINT('Ctrl Pts',(-0.000693203211584065,-0.0271787743898748,
-0.0147239408709482));
#39975=CARTESIAN_POINT('Ctrl Pts',(-0.000511222013638069,-0.0271787743898745,
-0.0147408433458497));
#39976=CARTESIAN_POINT('Ctrl Pts',(-0.000462148710303348,-0.0271787743898744,
-0.0147454012907765));
#39977=CARTESIAN_POINT('Ctrl Pts',(-0.000412939374657768,-0.0271787743898743,
-0.0147486309176275));
#39978=CARTESIAN_POINT('Ctrl Pts',(-0.000363653449390059,-0.0271787743898743,
-0.0147505091750227));
#39979=CARTESIAN_POINT('Ctrl Pts',(-0.000335973747865316,-0.0271787743898743,
-0.0147515640320393));
#39980=CARTESIAN_POINT('Ctrl Pts',(-0.000308269918835363,-0.0271787743898742,
-0.0147521925733346));
#39981=CARTESIAN_POINT('Ctrl Pts',(-0.000280552769976453,-0.0271787743898741,
-0.0147523901087495));
#39982=CARTESIAN_POINT('Ctrl Pts',(-0.000263915086500017,-0.0271787743898741,
-0.0147525086826953));
#39983=CARTESIAN_POINT('Ctrl Pts',(-0.000247272607789491,-0.0271787743898741,
-0.0147524719481251));
#39984=CARTESIAN_POINT('Ctrl Pts',(-0.000230627712965026,-0.027178774389874,
-0.0147522788149046));
#39985=CARTESIAN_POINT('Ctrl Pts',(-0.000216079303444679,-0.027178774389874,
-0.0147521100075187));
#39986=CARTESIAN_POINT('Ctrl Pts',(-0.000201531292573118,-0.027178774389874,
-0.0147518216826401));
#39987=CARTESIAN_POINT('Ctrl Pts',(-0.000186996318757126,-0.027178774389874,
-0.0147514136797492));
#39988=CARTESIAN_POINT('Ctrl Pts',(-9.88498753030835E-5,-0.0271787743898738,
-0.0147489393716279));
#39989=CARTESIAN_POINT('Ctrl Pts',(-1.10664436843476E-5,-0.0271787743898736,
-0.0147420666416071));
#39990=CARTESIAN_POINT('Ctrl Pts',(7.60196322764222E-5,-0.0271787743898741,
-0.014730708327085));
#39991=CARTESIAN_POINT('Ctrl Pts',(0.000165600962475197,-0.0271787743898746,
-0.0147190245657892));
#39992=CARTESIAN_POINT('Ctrl Pts',(0.00025444545205105,-0.0271787743898749,
-0.0147025947256612));
#39993=CARTESIAN_POINT('Ctrl Pts',(0.000342167409581488,-0.027178774389875,
-0.0146812694278629));
#39994=CARTESIAN_POINT('Ctrl Pts',(0.000423588645699061,-0.0271787743898751,
-0.0146614758418989));
#39995=CARTESIAN_POINT('Ctrl Pts',(0.000504043196429721,-0.0271787743898753,
-0.0146374642252552));
#39996=CARTESIAN_POINT('Ctrl Pts',(0.000583194675706476,-0.0271787743898754,
-0.0146090727027793));
#39997=CARTESIAN_POINT('Ctrl Pts',(0.000589319753685136,-0.0271787743898754,
-0.0146068756460636));
#39998=CARTESIAN_POINT('Ctrl Pts',(0.000595437012035837,-0.0271787743898754,
-0.0146046523408536));
#39999=CARTESIAN_POINT('Ctrl Pts',(0.000601546286299641,-0.0271787743898749,
-0.0146024027019753));
#40000=CARTESIAN_POINT('Origin',(0.,-0.0172787743898723,-0.0121758532865581));
#40001=CARTESIAN_POINT('',(0.0028,-0.0171787743898723,-0.0121758532865581));
#40002=CARTESIAN_POINT('',(0.0029,-0.0172787743898723,-0.0121758532865581));
#40003=CARTESIAN_POINT('Origin',(0.,-0.0171787743898623,-0.0121758532865581));
#40004=CARTESIAN_POINT('Origin',(0.,-0.0171787743898723,-0.0121758532865581));
#40005=CARTESIAN_POINT('Ctrl Pts',(0.00176574804943854,-0.0343694510790993,
-0.0139408222827216));
#40006=CARTESIAN_POINT('Ctrl Pts',(0.00117779798543426,-0.0343164323406156,
-0.0145290523617757));
#40007=CARTESIAN_POINT('Ctrl Pts',(-0.000621947546423068,-0.0342104065694797,
-0.0150611744231589));
#40008=CARTESIAN_POINT('Ctrl Pts',(-0.00276742883656761,-0.034051373765692,
-0.0132101082372629));
#40009=CARTESIAN_POINT('Ctrl Pts',(-0.00236482154393933,-0.0338923526677358,
-0.0104096023683696));
#40010=CARTESIAN_POINT('Ctrl Pts',(0.000204910886527884,-0.0337333315697798,
-0.00923059166728955));
#40011=CARTESIAN_POINT('Ctrl Pts',(0.00258846653129079,-0.0335743104718236,
-0.0107552119605033));
#40012=CARTESIAN_POINT('Ctrl Pts',(0.00259485856040026,-0.0334152893738676,
-0.0135839857225452));
#40013=CARTESIAN_POINT('Ctrl Pts',(0.000219742753097404,-0.0332562682759115,
-0.0151201044584147));
#40014=CARTESIAN_POINT('Ctrl Pts',(-0.00235736426033115,-0.0330972471779554,
-0.0139534669866695));
#40015=CARTESIAN_POINT('Ctrl Pts',(-0.00277031546347644,-0.0329382260799993,
-0.0111550102704199));
#40016=CARTESIAN_POINT('Ctrl Pts',(-0.000640244886201917,-0.0327792049820433,
-0.00929366988804862));
#40017=CARTESIAN_POINT('Ctrl Pts',(0.00207759635746219,-0.0326201838840872,
-0.010078116312487));
#40018=CARTESIAN_POINT('Ctrl Pts',(0.00288822476733986,-0.0324611627861311,
-0.0127882449165322));
#40019=CARTESIAN_POINT('Ctrl Pts',(0.00104752965503765,-0.032302141688175,
-0.0149362096781171));
#40020=CARTESIAN_POINT('Ctrl Pts',(-0.00175478257452117,-0.0321431205902189,
-0.0145502212948222));
#40021=CARTESIAN_POINT('Ctrl Pts',(-0.00294623597977783,-0.0319840994922628,
-0.0119846095548743));
#40022=CARTESIAN_POINT('Ctrl Pts',(-0.00143310357258225,-0.0318250783943067,
-0.00959455553988092));
#40023=CARTESIAN_POINT('Ctrl Pts',(0.00139559025190196,-0.0316660572963506,
-0.00957408303108934));
#40024=CARTESIAN_POINT('Ctrl Pts',(0.00294315991374164,-0.0315070361983945,
-0.0119419835692896));
#40025=CARTESIAN_POINT('Ctrl Pts',(0.00178896491918136,-0.0313480151004384,
-0.0145245742798952));
#40026=CARTESIAN_POINT('Ctrl Pts',(-0.00100746200682521,-0.0311889940024823,
-0.0149510805060739));
#40027=CARTESIAN_POINT('Ctrl Pts',(-0.0028790642322956,-0.0310299729045262,
-0.0128299910268252));
#40028=CARTESIAN_POINT('Ctrl Pts',(-0.00210773065532187,-0.0308709518065702,
-0.0101083992625063));
#40029=CARTESIAN_POINT('Ctrl Pts',(0.000598437139890697,-0.0307119307086141,
-0.00928472180902646));
#40030=CARTESIAN_POINT('Ctrl Pts',(0.002755292326791,-0.030552909610658,
-0.0111149852850437));
#40031=CARTESIAN_POINT('Ctrl Pts',(0.0023827642768738,-0.0303938885127019,
-0.0139192225077422));
#40032=CARTESIAN_POINT('Ctrl Pts',(-0.000176943674720605,-0.0302348674147459,
-0.0151228549563469));
#40033=CARTESIAN_POINT('Ctrl Pts',(-0.00257451101079573,-0.0300758463167898,
-0.0136216312142491));
#40034=CARTESIAN_POINT('Ctrl Pts',(-0.00260817017370304,-0.0299168252188337,
-0.0107923783780903));
#40035=CARTESIAN_POINT('Ctrl Pts',(-0.000248651555250166,-0.0297578041208776,
-0.00923473179216972));
#40036=CARTESIAN_POINT('Ctrl Pts',(0.00234119373410808,-0.0295987830229215,
-0.0103738661700957));
#40037=CARTESIAN_POINT('Ctrl Pts',(0.00277780667786063,-0.0294397535098039,
-0.0131736113086904));
#40038=CARTESIAN_POINT('Ctrl Pts',(0.0013745903082445,-0.0293337310293383,
-0.0144197667809647));
#40039=CARTESIAN_POINT('Ctrl Pts',(0.000564492329997462,-0.0292807155815248,
-0.0146077928730744));
#40040=CARTESIAN_POINT('Ctrl Pts',(0.00188614792707067,-0.0342711666745561,
-0.0140611690395707));
#40041=CARTESIAN_POINT('Ctrl Pts',(0.00125810770649936,-0.0342181479360723,
-0.0146895083683901));
#40042=CARTESIAN_POINT('Ctrl Pts',(-0.000664355866515366,-0.0341121221649365,
-0.01525791387978));
#40043=CARTESIAN_POINT('Ctrl Pts',(-0.00295612965001848,-0.0339530893611486,
-0.0132806302857199));
#40044=CARTESIAN_POINT('Ctrl Pts',(-0.00252607004403119,-0.0337940682631925,
-0.0102891682019633));
#40045=CARTESIAN_POINT('Ctrl Pts',(0.000218883007675803,-0.0336350471652364,
-0.00902976508919009));
#40046=CARTESIAN_POINT('Ctrl Pts',(0.00276496456209497,-0.0334760260672803,
-0.0106583436434915));
#40047=CARTESIAN_POINT('Ctrl Pts',(0.00277179244020502,-0.0333170049693242,
-0.0136800011042621));
#40048=CARTESIAN_POINT('Ctrl Pts',(0.000234726204780603,-0.0331579838713681,
-0.0153208621378145));
#40049=CARTESIAN_POINT('Ctrl Pts',(-0.00251810427562861,-0.032998962773412,
-0.0140746759394636));
#40050=CARTESIAN_POINT('Ctrl Pts',(-0.00295921310541975,-0.032839941675456,
-0.0110854027325473));
#40051=CARTESIAN_POINT('Ctrl Pts',(-0.000683900834726285,-0.0326809205774999,
-0.00909714438226979));
#40052=CARTESIAN_POINT('Ctrl Pts',(0.00221926002645898,-0.0325218994795438,
-0.00993507932877742));
#40053=CARTESIAN_POINT('Ctrl Pts',(0.00308516221188206,-0.0323628783815877,
-0.0128300016537604));
#40054=CARTESIAN_POINT('Ctrl Pts',(0.00111895685685313,-0.0322038572836316,
-0.0151244282475049));
#40055=CARTESIAN_POINT('Ctrl Pts',(-0.00187443475667168,-0.0320448361856755,
-0.0147121207332723));
#40056=CARTESIAN_POINT('Ctrl Pts',(-0.00314712899594364,-0.0318858150877194,
-0.0119715693468445));
#40057=CARTESIAN_POINT('Ctrl Pts',(-0.00153082164443737,-0.0317267939897633,
-0.00941854632218373));
#40058=CARTESIAN_POINT('Ctrl Pts',(0.001490750428127,-0.0315677728918073,
-0.0093966778681699));
#40059=CARTESIAN_POINT('Ctrl Pts',(0.00314384318425632,-0.0314087517938512,
-0.0119260368517781));
#40060=CARTESIAN_POINT('Ctrl Pts',(0.00191094786993477,-0.0312497306958951,
-0.0146847249425447));
#40061=CARTESIAN_POINT('Ctrl Pts',(-0.00107615714279284,-0.031090709597939,
-0.015140313062631));
#40062=CARTESIAN_POINT('Ctrl Pts',(-0.0030753770535804,-0.030931688499983,
-0.0128745942780693));
#40063=CARTESIAN_POINT('Ctrl Pts',(-0.00225144907147014,-0.0307726674020269,
-0.00996742716199346));
#40064=CARTESIAN_POINT('Ctrl Pts',(0.000639242371665568,-0.0306136463040708,
-0.0090875861665865));
#40065=CARTESIAN_POINT('Ctrl Pts',(0.00294316559619194,-0.0304546252061146,
-0.0110426485903456));
#40066=CARTESIAN_POINT('Ctrl Pts',(0.00254523622605875,-0.0302956041081586,
-0.0140380964552258));
#40067=CARTESIAN_POINT('Ctrl Pts',(-0.000189008814359819,-0.0301365830102025,
-0.0153238001821038));
#40068=CARTESIAN_POINT('Ctrl Pts',(-0.0027500574658865,-0.0299775619122464,
-0.013720213503853));
#40069=CARTESIAN_POINT('Ctrl Pts',(-0.00278601172355351,-0.0298185408142903,
-0.0106980443026601));
#40070=CARTESIAN_POINT('Ctrl Pts',(-0.000265606192031256,-0.0296595197163342,
-0.00903418751398792));
#40071=CARTESIAN_POINT('Ctrl Pts',(0.00250083114058254,-0.0295004986183781,
-0.0102509952835128));
#40072=CARTESIAN_POINT('Ctrl Pts',(0.00296721511821342,-0.0293414691052605,
-0.013241644765564));
#40073=CARTESIAN_POINT('Ctrl Pts',(0.00146831857539992,-0.029235446624795,
-0.0145727710049986));
#40074=CARTESIAN_POINT('Ctrl Pts',(0.00060298298979322,-0.0291824311769814,
-0.0147736179061069));
#40075=CARTESIAN_POINT('Ctrl Pts',(0.00200654780470278,-0.0341728822700128,
-0.0141815157964198));
#40076=CARTESIAN_POINT('Ctrl Pts',(0.00133841742756444,-0.034119863531529,
-0.0148499643750045));
#40077=CARTESIAN_POINT('Ctrl Pts',(-0.000706764186607663,-0.0340138377603931,
-0.0154546533364009));
#40078=CARTESIAN_POINT('Ctrl Pts',(-0.00314483046346935,-0.0338548049566054,
-0.0133511523341767));
#40079=CARTESIAN_POINT('Ctrl Pts',(-0.00268731854412305,-0.0336957838586492,
-0.0101687340355571));
#40080=CARTESIAN_POINT('Ctrl Pts',(0.000232855128823719,-0.0335367627606931,
-0.00882893851109065));
#40081=CARTESIAN_POINT('Ctrl Pts',(0.00294146259289918,-0.033377741662737,
-0.0105614753264796));
#40082=CARTESIAN_POINT('Ctrl Pts',(0.00294872632000978,-0.0332187205647809,
-0.0137760164859788));
#40083=CARTESIAN_POINT('Ctrl Pts',(0.000249709656463804,-0.0330596994668248,
-0.0155216198172141));
#40084=CARTESIAN_POINT('Ctrl Pts',(-0.00267884429092607,-0.0329006783688689,
-0.0141958848922576));
#40085=CARTESIAN_POINT('Ctrl Pts',(-0.00314811074736304,-0.0327416572709126,
-0.0110157951946748));
#40086=CARTESIAN_POINT('Ctrl Pts',(-0.000727556783250659,-0.0325826361729567,
-0.00890061887649098));
#40087=CARTESIAN_POINT('Ctrl Pts',(0.00236092369545578,-0.0324236150750004,
-0.00979204234506796));
#40088=CARTESIAN_POINT('Ctrl Pts',(0.00328209965642423,-0.0322645939770444,
-0.0128717583909887));
#40089=CARTESIAN_POINT('Ctrl Pts',(0.00119038405866861,-0.0321055728790883,
-0.0153126468168928));
#40090=CARTESIAN_POINT('Ctrl Pts',(-0.00199408693882221,-0.0319465517811322,
-0.0148740201717226));
#40091=CARTESIAN_POINT('Ctrl Pts',(-0.00334802201210944,-0.0317875306831761,
-0.011958529138815));
#40092=CARTESIAN_POINT('Ctrl Pts',(-0.00162853971629248,-0.0316285095852202,
-0.00924253710448655));
#40093=CARTESIAN_POINT('Ctrl Pts',(0.00158591060435204,-0.0314694884872639,
-0.00921927270525046));
#40094=CARTESIAN_POINT('Ctrl Pts',(0.00334452645477101,-0.031310467389308,
-0.0119100901342666));
#40095=CARTESIAN_POINT('Ctrl Pts',(0.00203293082068818,-0.0311514462913518,
-0.0148448756051943));
#40096=CARTESIAN_POINT('Ctrl Pts',(-0.00114485227876049,-0.0309924251933957,
-0.0153295456191882));
#40097=CARTESIAN_POINT('Ctrl Pts',(-0.00327168987486519,-0.0308334040954397,
-0.0129191975293132));
#40098=CARTESIAN_POINT('Ctrl Pts',(-0.00239516748761842,-0.0306743829974836,
-0.00982645506148058));
#40099=CARTESIAN_POINT('Ctrl Pts',(0.000680047603440434,-0.0305153618995274,
-0.00889045052414654));
#40100=CARTESIAN_POINT('Ctrl Pts',(0.0031310388655929,-0.0303563408015715,
-0.0109703118956475));
#40101=CARTESIAN_POINT('Ctrl Pts',(0.00270770817524368,-0.0301973197036154,
-0.0141569704027094));
#40102=CARTESIAN_POINT('Ctrl Pts',(-0.000201073953999031,-0.0300382986056592,
-0.0155247454078606));
#40103=CARTESIAN_POINT('Ctrl Pts',(-0.00292560392097725,-0.0298792775077031,
-0.0138187957934569));
#40104=CARTESIAN_POINT('Ctrl Pts',(-0.00296385327340397,-0.029720256409747,
-0.0106037102272297));
#40105=CARTESIAN_POINT('Ctrl Pts',(-0.000282560828812347,-0.0295612353117909,
-0.00883364323580613));
#40106=CARTESIAN_POINT('Ctrl Pts',(0.002660468547057,-0.0294022142138348,
-0.0101281243969297));
#40107=CARTESIAN_POINT('Ctrl Pts',(0.00315662355856618,-0.0292431847007172,
-0.0133096782224377));
#40108=CARTESIAN_POINT('Ctrl Pts',(0.00156204684255533,-0.0291371622202517,
-0.0147257752290324));
#40109=CARTESIAN_POINT('Ctrl Pts',(0.000641473649588978,-0.0290841467724382,
-0.0149394429391394));
#40110=CARTESIAN_POINT('Ctrl Pts',(0.0021269476823349,-0.0340745978654695,
-0.0143018625532689));
#40111=CARTESIAN_POINT('Ctrl Pts',(0.00141872714862954,-0.0340215791269856,
-0.0150104203816191));
#40112=CARTESIAN_POINT('Ctrl Pts',(-0.000749172506699962,-0.0339155533558498,
-0.0156513927930219));
#40113=CARTESIAN_POINT('Ctrl Pts',(-0.00333353127692023,-0.033756520552062,
-0.0134216743826337));
#40114=CARTESIAN_POINT('Ctrl Pts',(-0.00284856704421491,-0.0335974994541059,
-0.0100482998691509));
#40115=CARTESIAN_POINT('Ctrl Pts',(0.000246827249971632,-0.0334384783561498,
-0.0086281119329912));
#40116=CARTESIAN_POINT('Ctrl Pts',(0.00311796062370337,-0.0332794572581937,
-0.0104646070094678));
#40117=CARTESIAN_POINT('Ctrl Pts',(0.00312566019981454,-0.0331204361602375,
-0.0138720318676957));
#40118=CARTESIAN_POINT('Ctrl Pts',(0.000264693108147008,-0.0329614150622815,
-0.0157223774966138));
#40119=CARTESIAN_POINT('Ctrl Pts',(-0.00283958430622353,-0.0328023939643254,
-0.0143170938450517));
#40120=CARTESIAN_POINT('Ctrl Pts',(-0.00333700838930635,-0.0326433728663693,
-0.0109461876568023));
#40121=CARTESIAN_POINT('Ctrl Pts',(-0.000771212731775031,-0.0324843517684132,
-0.00870409337071217));
#40122=CARTESIAN_POINT('Ctrl Pts',(0.00250258736445257,-0.0323253306704572,
-0.00964900536135851));
#40123=CARTESIAN_POINT('Ctrl Pts',(0.00347903710096643,-0.0321663095725011,
-0.0129135151282171));
#40124=CARTESIAN_POINT('Ctrl Pts',(0.0012618112604841,-0.032007288474545,
-0.0155008653862805));
#40125=CARTESIAN_POINT('Ctrl Pts',(-0.0021137391209727,-0.0318482673765889,
-0.0150359196101727));
#40126=CARTESIAN_POINT('Ctrl Pts',(-0.00354891502827525,-0.0316892462786328,
-0.0119454889307853));
#40127=CARTESIAN_POINT('Ctrl Pts',(-0.00172625778814758,-0.0315302251806767,
-0.00906652788678938));
#40128=CARTESIAN_POINT('Ctrl Pts',(0.00168107078057706,-0.0313712040827206,
-0.00904186754233102));
#40129=CARTESIAN_POINT('Ctrl Pts',(0.0035452097252857,-0.0312121829847645,
-0.0118941434167551));
#40130=CARTESIAN_POINT('Ctrl Pts',(0.00215491377144159,-0.0310531618868085,
-0.0150050262678438));
#40131=CARTESIAN_POINT('Ctrl Pts',(-0.00121354741472812,-0.0308941407888524,
-0.0155187781757453));
#40132=CARTESIAN_POINT('Ctrl Pts',(-0.00346800269614999,-0.0307351196908962,
-0.0129638007805572));
#40133=CARTESIAN_POINT('Ctrl Pts',(-0.0025388859037667,-0.0305760985929401,
-0.00968548296096771));
#40134=CARTESIAN_POINT('Ctrl Pts',(0.000720852835215301,-0.030417077494984,
-0.00869331488170658));
#40135=CARTESIAN_POINT('Ctrl Pts',(0.00331891213499383,-0.030258056397028,
-0.0108979752009492));
#40136=CARTESIAN_POINT('Ctrl Pts',(0.00287018012442863,-0.0300990352990719,
-0.014275844350193));
#40137=CARTESIAN_POINT('Ctrl Pts',(-0.000213139093638245,-0.0299400142011158,
-0.0157256906336175));
#40138=CARTESIAN_POINT('Ctrl Pts',(-0.00310115037606801,-0.0297809931031597,
-0.0139173780830608));
#40139=CARTESIAN_POINT('Ctrl Pts',(-0.00314169482325445,-0.0296219720052037,
-0.0105093761517993));
#40140=CARTESIAN_POINT('Ctrl Pts',(-0.000299515465593438,-0.0294629509072476,
-0.00863309895762433));
#40141=CARTESIAN_POINT('Ctrl Pts',(0.00282010595353146,-0.0293039298092915,
-0.0100052535103467));
#40142=CARTESIAN_POINT('Ctrl Pts',(0.00334603199891895,-0.0291449002961739,
-0.0133777116793113));
#40143=CARTESIAN_POINT('Ctrl Pts',(0.00165577510971075,-0.0290388778157083,
-0.0148787794530662));
#40144=CARTESIAN_POINT('Ctrl Pts',(0.000679964309384735,-0.0289858623678948,
-0.015105267972172));
#40145=CARTESIAN_POINT('Ctrl Pts',(0.00267357255235765,-0.0292787743898725,
-0.0108117659595362));
#40146=CARTESIAN_POINT('Ctrl Pts',(0.00270942158183447,-0.0292787743769101,
-0.0109044263882472));
#40147=CARTESIAN_POINT('Ctrl Pts',(0.00274057340703459,-0.0292787743898644,
-0.0109987720071259));
#40148=CARTESIAN_POINT('Ctrl Pts',(0.00276704473487997,-0.0292787743898645,
-0.0110943957950434));
#40149=CARTESIAN_POINT('Ctrl Pts',(0.00284508802080715,-0.0292787743898647,
-0.0113763157147949));
#40150=CARTESIAN_POINT('Ctrl Pts',(0.0028827204075281,-0.0292787743898651,
-0.0116697038393258));
#40151=CARTESIAN_POINT('Ctrl Pts',(0.00287783547757714,-0.0292787743898655,
-0.011963215493794));
#40152=CARTESIAN_POINT('Ctrl Pts',(0.00287617507520755,-0.0292787743898657,
-0.0120629809871526));
#40153=CARTESIAN_POINT('Ctrl Pts',(0.00286958813063577,-0.029278774389866,
-0.0121623132322861));
#40154=CARTESIAN_POINT('Ctrl Pts',(0.00285803849087999,-0.0292787743898655,
-0.0122608040104835));
#40155=CARTESIAN_POINT('Ctrl Pts',(0.00282980275969606,-0.0292787743898642,
-0.0125015872033864));
#40156=CARTESIAN_POINT('Ctrl Pts',(0.00277204190124365,-0.0292787743898644,
-0.0127374351857662));
#40157=CARTESIAN_POINT('Ctrl Pts',(0.00268282981823786,-0.0292787743898641,
-0.0129617552268038));
#40158=CARTESIAN_POINT('Ctrl Pts',(0.00267753866184219,-0.0292787743898641,
-0.0129750596176421));
#40159=CARTESIAN_POINT('Ctrl Pts',(0.00267213630271764,-0.0292787743898641,
-0.012988323028573));
#40160=CARTESIAN_POINT('Ctrl Pts',(0.00266662212529158,-0.0292787743898641,
-0.013001543904261));
#40161=CARTESIAN_POINT('Ctrl Pts',(0.00266099360072982,-0.0292787743898641,
-0.0130150389403812));
#40162=CARTESIAN_POINT('Ctrl Pts',(0.00265525166642689,-0.0292787743898641,
-0.0130284821681761));
#40163=CARTESIAN_POINT('Ctrl Pts',(0.0026493980102342,-0.0292787743898641,
-0.0130418677383362));
#40164=CARTESIAN_POINT('Ctrl Pts',(0.00263902493206007,-0.0292787743898641,
-0.0130655878819704));
#40165=CARTESIAN_POINT('Ctrl Pts',(0.0026282991561088,-0.029278774389864,
-0.013089131499636));
#40166=CARTESIAN_POINT('Ctrl Pts',(0.00261721939710271,-0.029278774389864,
-0.0131124910242309));
#40167=CARTESIAN_POINT('Ctrl Pts',(0.00248779252520929,-0.0292787743898638,
-0.0133853625005478));
#40168=CARTESIAN_POINT('Ctrl Pts',(0.00231037877727216,-0.0292787743898636,
-0.0136334676728105));
#40169=CARTESIAN_POINT('Ctrl Pts',(0.00209532275943825,-0.0292787743898636,
-0.0138485399734916));
#40170=CARTESIAN_POINT('Ctrl Pts',(0.00208085851571133,-0.0292787743898636,
-0.0138630053123707));
#40171=CARTESIAN_POINT('Ctrl Pts',(0.00206621895014382,-0.0292787743898636,
-0.0138773230384675));
#40172=CARTESIAN_POINT('Ctrl Pts',(0.0020514297876405,-0.0292787743898636,
-0.0138914683166346));
#40173=CARTESIAN_POINT('Ctrl Pts',(0.00188347219527991,-0.0292787743898637,
-0.0140521134419883));
#40174=CARTESIAN_POINT('Ctrl Pts',(0.00169583105268622,-0.0292787743898637,
-0.0141911607834212));
#40175=CARTESIAN_POINT('Ctrl Pts',(0.00149313379990858,-0.0292787743898639,
-0.0143044621723636));
#40176=CARTESIAN_POINT('Ctrl Pts',(0.00146908053839098,-0.0292787743898639,
-0.0143179071890138));
#40177=CARTESIAN_POINT('Ctrl Pts',(0.00144481456590165,-0.0292787743898639,
-0.0143309872340784));
#40178=CARTESIAN_POINT('Ctrl Pts',(0.00142034322819153,-0.029278774389864,
-0.0143436933191354));
#40179=CARTESIAN_POINT('Ctrl Pts',(0.00140470331950154,-0.029278774389864,
-0.0143518139217952));
#40180=CARTESIAN_POINT('Ctrl Pts',(0.00138897952649762,-0.029278774389864,
-0.0143597817659317));
#40181=CARTESIAN_POINT('Ctrl Pts',(0.00137317376994739,-0.029278774389864,
-0.0143675944004388));
#40182=CARTESIAN_POINT('Ctrl Pts',(0.00136117393413807,-0.029278774389864,
-0.0143735258046728));
#40183=CARTESIAN_POINT('Ctrl Pts',(0.0013491292146614,-0.029278774389864,
-0.0143793665313414));
#40184=CARTESIAN_POINT('Ctrl Pts',(0.00133704814932165,-0.029278774389864,
-0.0143851120911698));
#40185=CARTESIAN_POINT('Ctrl Pts',(0.00109928812760478,-0.0292787743898642,
-0.0144981869228298));
#40186=CARTESIAN_POINT('Ctrl Pts',(0.000846613469422695,-0.0292787743898645,
-0.0145751840384429));
#40187=CARTESIAN_POINT('Ctrl Pts',(0.000585792948533347,-0.029278774389865,
-0.0146085347508578));
#40188=CARTESIAN_POINT('Ctrl Pts',(0.000579083537205416,-0.029278774389865,
-0.0146093926727993));
#40189=CARTESIAN_POINT('Ctrl Pts',(0.000572368752880877,-0.029278774389865,
-0.0146102214611691));
#40190=CARTESIAN_POINT('Ctrl Pts',(0.000565648716062883,-0.029278774389865,
-0.0146110209461011));
#40191=CARTESIAN_POINT('Ctrl Pts',(-0.00214342189834001,-0.034078774389864,
-0.0134651256783301));
#40192=CARTESIAN_POINT('Ctrl Pts',(-0.00203881996138949,-0.0340787743898638,
-0.0136859499145821));
#40193=CARTESIAN_POINT('Ctrl Pts',(-0.00190154780260284,-0.0340787743898637,
-0.0138907123562036));
#40194=CARTESIAN_POINT('Ctrl Pts',(-0.00173853782088977,-0.0340787743898637,
-0.014074484164648));
#40195=CARTESIAN_POINT('Ctrl Pts',(-0.00172188027006473,-0.0340787743898637,
-0.014093263310607));
#40196=CARTESIAN_POINT('Ctrl Pts',(-0.00170495136862563,-0.0340787743898636,
-0.0141118225411361));
#40197=CARTESIAN_POINT('Ctrl Pts',(-0.00168775685180314,-0.0340787743898637,
-0.0141301559522264));
#40198=CARTESIAN_POINT('Ctrl Pts',(-0.00167336442387989,-0.0340787743898637,
-0.0141455016755421));
#40199=CARTESIAN_POINT('Ctrl Pts',(-0.00165878196066412,-0.0340787743898637,
-0.0141606930102152));
#40200=CARTESIAN_POINT('Ctrl Pts',(-0.00164403551346177,-0.0340787743898637,
-0.014175703674688));
#40201=CARTESIAN_POINT('Ctrl Pts',(-0.00144997531169396,-0.0340787743898636,
-0.0143732409212044));
#40202=CARTESIAN_POINT('Ctrl Pts',(-0.00122722417391643,-0.0340787743898636,
-0.0145403352498076));
#40203=CARTESIAN_POINT('Ctrl Pts',(-0.000984003088329723,-0.0340787743898639,
-0.0146696633580869));
#40204=CARTESIAN_POINT('Ctrl Pts',(-0.000971343819170138,-0.034078774389864,
-0.0146763946796278));
#40205=CARTESIAN_POINT('Ctrl Pts',(-0.000958629164297646,-0.034078774389864,
-0.0146830225748522));
#40206=CARTESIAN_POINT('Ctrl Pts',(-0.000945871640704679,-0.034078774389864,
-0.0146895401571214));
#40207=CARTESIAN_POINT('Ctrl Pts',(-0.000862042915607934,-0.034078774389864,
-0.014732366698523));
#40208=CARTESIAN_POINT('Ctrl Pts',(-0.000776237932625443,-0.0340787743898641,
-0.0147705018511941));
#40209=CARTESIAN_POINT('Ctrl Pts',(-0.00068878756990034,-0.0340787743898642,
-0.0148036883024632));
#40210=CARTESIAN_POINT('Ctrl Pts',(-0.000652192714614692,-0.0340787743898642,
-0.0148175756477388));
#40211=CARTESIAN_POINT('Ctrl Pts',(-0.000615309219919732,-0.0340787743898643,
-0.0148305960499244));
#40212=CARTESIAN_POINT('Ctrl Pts',(-0.000578159304347232,-0.0340787743898643,
-0.0148427288545622));
#40213=CARTESIAN_POINT('Ctrl Pts',(-0.000405102583540647,-0.0340787743898646,
-0.014899247512881));
#40214=CARTESIAN_POINT('Ctrl Pts',(-0.000226292457930033,-0.0340787743898648,
-0.0149365677617328));
#40215=CARTESIAN_POINT('Ctrl Pts',(-4.4359070532995E-5,-0.034078774389865,
-0.0149557093126185));
#40216=CARTESIAN_POINT('Ctrl Pts',(-2.60444274983421E-5,-0.034078774389865,
-0.0149576362303581));
#40217=CARTESIAN_POINT('Ctrl Pts',(-7.69789496846054E-6,-0.0340787743898651,
-0.0149593782812497));
#40218=CARTESIAN_POINT('Ctrl Pts',(1.06779760546631E-5,-0.0340787743898655,
-0.0149609360713358));
#40219=CARTESIAN_POINT('Ctrl Pts',(2.82810386610846E-5,-0.0340787743898659,
-0.0149624283476137));
#40220=CARTESIAN_POINT('Ctrl Pts',(4.59139311838308E-5,-0.0340787743898658,
-0.0149637516227164));
#40221=CARTESIAN_POINT('Ctrl Pts',(6.35497484007623E-5,-0.0340787743898657,
-0.0149649050553157));
#40222=CARTESIAN_POINT('Ctrl Pts',(0.000405656097217325,-0.0340787743898652,
-0.0149872797834223));
#40223=CARTESIAN_POINT('Ctrl Pts',(0.000750534762719912,-0.0340787743898648,
-0.0149466263762361));
#40224=CARTESIAN_POINT('Ctrl Pts',(0.00108150703137315,-0.0340787743898644,
-0.0148487557072035));
#40225=CARTESIAN_POINT('Ctrl Pts',(0.00109597282815472,-0.0340787743898644,
-0.0148444780762864));
#40226=CARTESIAN_POINT('Ctrl Pts',(0.00111041391370224,-0.0340787743898644,
-0.0148400892861284));
#40227=CARTESIAN_POINT('Ctrl Pts',(0.00112482350330411,-0.0340787743898644,
-0.0148355911496298));
#40228=CARTESIAN_POINT('Ctrl Pts',(0.00140950929982585,-0.034078774389864,
-0.0147467228607084));
#40229=CARTESIAN_POINT('Ctrl Pts',(0.00167901061227646,-0.0340787743898638,
-0.0146164309612491));
#40230=CARTESIAN_POINT('Ctrl Pts',(0.00192310254496218,-0.0340787743898638,
-0.0144476154136012));
#40231=CARTESIAN_POINT('Ctrl Pts',(0.0019912392349424,-0.0340787743898637,
-0.0144004916413922));
#40232=CARTESIAN_POINT('Ctrl Pts',(0.0020573924532646,-0.0340787743898637,
-0.0143503417818491));
#40233=CARTESIAN_POINT('Ctrl Pts',(0.00212132034355962,-0.0340787743898724,
-0.0142971736301177));
#40234=CARTESIAN_POINT('Origin',(3.47714923605922E-19,-0.0340787743898723,
-0.0121758532865581));
#40235=CARTESIAN_POINT('',(-0.00300000000001,-0.0340787743898623,-0.0121758532865581));
#40236=CARTESIAN_POINT('Origin',(0.,-0.0340787743898623,-0.0121758532865581));
#40237=CARTESIAN_POINT('Ctrl Pts',(0.00299997408502258,-0.0340787743898722,
-0.0121633837535663));
#40238=CARTESIAN_POINT('Ctrl Pts',(0.00298983422017737,-0.0340787745628727,
-0.0120688605133317));
#40239=CARTESIAN_POINT('Ctrl Pts',(0.00297516577473772,-0.0340787743898748,
-0.0119748920917585));
#40240=CARTESIAN_POINT('Ctrl Pts',(0.00295613328802263,-0.0340787743898749,
-0.0118817936805995));
#40241=CARTESIAN_POINT('Ctrl Pts',(0.00291449826526791,-0.0340787743898751,
-0.011678133773985));
#40242=CARTESIAN_POINT('Ctrl Pts',(0.00285202694145493,-0.0340787743898755,
-0.0114785958149418));
#40243=CARTESIAN_POINT('Ctrl Pts',(0.00276980767921813,-0.0340787743898755,
-0.0112867975378626));
#40244=CARTESIAN_POINT('Ctrl Pts',(0.00276313869579095,-0.0340787743898755,
-0.011271240361887));
#40245=CARTESIAN_POINT('Ctrl Pts',(0.00275633938651183,-0.0340787743898755,
-0.0112557344634974));
#40246=CARTESIAN_POINT('Ctrl Pts',(0.00274941013017219,-0.0340787743898755,
-0.0112402819807807));
#40247=CARTESIAN_POINT('Ctrl Pts',(0.00274257548204977,-0.0340787743898755,
-0.01122504047768));
#40248=CARTESIAN_POINT('Ctrl Pts',(0.00273561765327543,-0.0340787743898756,
-0.0112098582491205));
#40249=CARTESIAN_POINT('Ctrl Pts',(0.00272853986062164,-0.0340787743898756,
-0.0111947423811783));
#40250=CARTESIAN_POINT('Ctrl Pts',(0.00261926295131071,-0.0340787743898758,
-0.0109613623697716));
#40251=CARTESIAN_POINT('Ctrl Pts',(0.0024813567361139,-0.0340787743898759,
-0.0107432447506426));
#40252=CARTESIAN_POINT('Ctrl Pts',(0.00231681416997636,-0.0340787743898759,
-0.0105475950993701));
#40253=CARTESIAN_POINT('Ctrl Pts',(0.00229331961457605,-0.0340787743898759,
-0.0105196588535781));
#40254=CARTESIAN_POINT('Ctrl Pts',(0.00226927930088061,-0.0340787743898759,
-0.0104921842003603));
#40255=CARTESIAN_POINT('Ctrl Pts',(0.00224469656570801,-0.0340787743898759,
-0.0104651960118044));
#40256=CARTESIAN_POINT('Ctrl Pts',(0.00214084894393267,-0.0340787743898759,
-0.0103511867619029));
#40257=CARTESIAN_POINT('Ctrl Pts',(0.00202796472163855,-0.0340787743898759,
-0.0102465484986737));
#40258=CARTESIAN_POINT('Ctrl Pts',(0.00190673318272766,-0.0340787743898759,
-0.0101531055610276));
#40259=CARTESIAN_POINT('Ctrl Pts',(0.00175487922115659,-0.0340787743898758,
-0.0100360594491834));
#40260=CARTESIAN_POINT('Ctrl Pts',(0.00158979661873312,-0.0340787743898757,
-0.00993641896279302));
#40261=CARTESIAN_POINT('Ctrl Pts',(0.00141474219894874,-0.0340787743898755,
-0.0098549840709787));
#40262=CARTESIAN_POINT('Ctrl Pts',(0.00140014729757205,-0.0340787743898755,
-0.00984819455823109));
#40263=CARTESIAN_POINT('Ctrl Pts',(0.00138548304086077,-0.0340787743898755,
-0.00984153210814379));
#40264=CARTESIAN_POINT('Ctrl Pts',(0.00137075131632936,-0.0340787743898755,
-0.00983499746591276));
#40265=CARTESIAN_POINT('Ctrl Pts',(0.00135722807646553,-0.0340787743898755,
-0.00982899887870553));
#40266=CARTESIAN_POINT('Ctrl Pts',(0.00134365490868854,-0.0340787743898755,
-0.00982311109996221));
#40267=CARTESIAN_POINT('Ctrl Pts',(0.00133003924889329,-0.0340787743898755,
-0.0098173367535274));
#40268=CARTESIAN_POINT('Ctrl Pts',(0.00105134533856905,-0.0340787743898752,
-0.00969914378956656));
#40269=CARTESIAN_POINT('Ctrl Pts',(0.000754090522326119,-0.0340787743898749,
-0.00962763092554494));
#40270=CARTESIAN_POINT('Ctrl Pts',(0.000451492268503984,-0.0340787743898744,
-0.00960616484366454));
#40271=CARTESIAN_POINT('Ctrl Pts',(0.000428385096958881,-0.0340787743898744,
-0.00960452563910818));
#40272=CARTESIAN_POINT('Ctrl Pts',(0.000405247230892682,-0.0340787743898743,
-0.00960318119938207));
#40273=CARTESIAN_POINT('Ctrl Pts',(0.000382084954837052,-0.0340787743898743,
-0.00960213448339256));
#40274=CARTESIAN_POINT('Ctrl Pts',(0.000279580069589831,-0.0340787743898742,
-0.00959750223127132));
#40275=CARTESIAN_POINT('Ctrl Pts',(0.000177094560444756,-0.0340787743898738,
-0.00959872195292196));
#40276=CARTESIAN_POINT('Ctrl Pts',(7.52901806218787E-5,-0.0340787743898741,
-0.00960590461313921));
#40277=CARTESIAN_POINT('Ctrl Pts',(-9.57122147715958E-5,-0.0340787743898747,
-0.00961796943888233));
#40278=CARTESIAN_POINT('Ctrl Pts',(-0.000264954695593333,-0.0340787743898749,
-0.00964681365331277));
#40279=CARTESIAN_POINT('Ctrl Pts',(-0.00042980566833564,-0.0340787743898751,
-0.00969349766606961));
#40280=CARTESIAN_POINT('Ctrl Pts',(-0.000487639239516593,-0.0340787743898752,
-0.00970987550800693));
#40281=CARTESIAN_POINT('Ctrl Pts',(-0.000544928777483045,-0.0340787743898753,
-0.00972845541296338));
#40282=CARTESIAN_POINT('Ctrl Pts',(-0.000601546286299631,-0.0340787743898749,
-0.00974930387114081));
#40283=CARTESIAN_POINT('Origin',(0.,-0.0340787743898623,-0.0121758532865581));
#40284=CARTESIAN_POINT('Ctrl Pts',(-0.000724274042549492,-0.0343719489147863,
-0.00925661861704697));
#40285=CARTESIAN_POINT('Ctrl Pts',(0.000248170763243804,-0.034318931779031,
-0.00901533557115846));
#40286=CARTESIAN_POINT('Ctrl Pts',(0.00243605023693017,-0.0342129076106235,
-0.00958549404345891));
#40287=CARTESIAN_POINT('Ctrl Pts',(0.00349868472071628,-0.0340538764095642,
-0.0128296735919113));
#40288=CARTESIAN_POINT('Ctrl Pts',(0.00134170352018559,-0.033894855311608,
-0.0154689316834747));
#40289=CARTESIAN_POINT('Ctrl Pts',(-0.0020430070581503,-0.033735834213652,
-0.0150874279970315));
#40290=CARTESIAN_POINT('Ctrl Pts',(-0.0035543079777708,-0.0335768131156959,
-0.0120320136823328));
#40291=CARTESIAN_POINT('Ctrl Pts',(-0.00180176699430847,-0.0334177920177398,
-0.00910923480492393));
#40292=CARTESIAN_POINT('Ctrl Pts',(0.00160421041412461,-0.0332587709197837,
-0.00900124265134754));
#40293=CARTESIAN_POINT('Ctrl Pts',(0.00353784086413984,-0.0330997498218276,
-0.0118076421117317));
#40294=CARTESIAN_POINT('Ctrl Pts',(0.00222365303830162,-0.0329407287238715,
-0.0149519682884868));
#40295=CARTESIAN_POINT('Ctrl Pts',(-0.00113172692687037,-0.0327817076259155,
-0.0155479188897315));
#40296=CARTESIAN_POINT('Ctrl Pts',(-0.00344824427242963,-0.0326226865279594,
-0.0130483563484526));
#40297=CARTESIAN_POINT('Ctrl Pts',(-0.00259931962519099,-0.0324636654300033,
-0.00974786494194555));
#40298=CARTESIAN_POINT('Ctrl Pts',(0.000635718683001802,-0.0323046443320472,
-0.0086762131723468));
#40299=CARTESIAN_POINT('Ctrl Pts',(0.00328718528952945,-0.0321456232340911,
-0.0108171659297137));
#40300=CARTESIAN_POINT('Ctrl Pts',(0.00292107726441006,-0.031986602136135,
-0.0142053653426598));
#40301=CARTESIAN_POINT('Ctrl Pts',(-0.000126521491820488,-0.0318275810381789,
-0.0157305134276381));
#40302=CARTESIAN_POINT('Ctrl Pts',(-0.0030579759603136,-0.0316685599402228,
-0.013992552104926));
#40303=CARTESIAN_POINT('Ctrl Pts',(-0.00318226944401077,-0.0315095388422667,
-0.0105868977657637));
#40304=CARTESIAN_POINT('Ctrl Pts',(-0.000385298871985522,-0.0313505177443106,
-0.00863987195853032));
#40305=CARTESIAN_POINT('Ctrl Pts',(0.00276536268907811,-0.0311914966463545,
-0.0099388107940399));
#40306=CARTESIAN_POINT('Ctrl Pts',(0.00337748671553294,-0.0310324755483984,
-0.013291305500576));
#40307=CARTESIAN_POINT('Ctrl Pts',(0.000889122011464058,-0.0308734544504424,
-0.0156198472351357));
#40308=CARTESIAN_POINT('Ctrl Pts',(-0.00241539722144602,-0.0307144333524863,
-0.0147868499547505));
#40309=CARTESIAN_POINT('Ctrl Pts',(-0.00350270981497701,-0.0305554122545302,
-0.0115570468537307));
#40310=CARTESIAN_POINT('Ctrl Pts',(-0.00137444815928839,-0.0303963911565741,
-0.00889522286003844));
#40311=CARTESIAN_POINT('Ctrl Pts',(0.00201523246796173,-0.0302373700586181,
-0.00924509377514259));
#40312=CARTESIAN_POINT('Ctrl Pts',(0.00355554012085794,-0.030078348960662,
-0.0122850754526157));
#40313=CARTESIAN_POINT('Ctrl Pts',(0.00183083526626607,-0.0299193278627059,
-0.015225310182813));
#40314=CARTESIAN_POINT('Ctrl Pts',(-0.00157243363987404,-0.0297603067647498,
-0.0153652084114242));
#40315=CARTESIAN_POINT('Ctrl Pts',(-0.00353631530869309,-0.0296012856667937,
-0.0125792758989247));
#40316=CARTESIAN_POINT('Ctrl Pts',(-0.00224571395583235,-0.0294422535936614,
-0.00941883780444782));
#40317=CARTESIAN_POINT('Ctrl Pts',(-2.28054016345844E-5,-0.0293362285531812,
-0.00900568258223235));
#40318=CARTESIAN_POINT('Ctrl Pts',(0.000930034741678471,-0.0292832105453529,
-0.00931551426486963));
#40319=CARTESIAN_POINT('Ctrl Pts',(-0.000683227961914626,-0.0342735368066846,
-0.00942205757329488));
#40320=CARTESIAN_POINT('Ctrl Pts',(0.000234106422178279,-0.0342205196709293,
-0.00919444852754381));
#40321=CARTESIAN_POINT('Ctrl Pts',(0.00229799432358602,-0.0341144955025218,
-0.00973229496150817));
#40322=CARTESIAN_POINT('Ctrl Pts',(0.00330040715348911,-0.0339554643014624,
-0.0127926202676201));
#40323=CARTESIAN_POINT('Ctrl Pts',(0.00126566645735814,-0.0337964432035063,
-0.0152823062441023));
#40324=CARTESIAN_POINT('Ctrl Pts',(-0.00192722569982459,-0.0336374221055502,
-0.0149224231462159));
#40325=CARTESIAN_POINT('Ctrl Pts',(-0.00335287812762294,-0.0334784010075941,
-0.0120401653647717));
#40326=CARTESIAN_POINT('Ctrl Pts',(-0.00169965720024032,-0.033319379909638,
-0.00928302630106875));
#40327=CARTESIAN_POINT('Ctrl Pts',(0.00151329655259554,-0.0331603588116819,
-0.00918115428211436));
#40328=CARTESIAN_POINT('Ctrl Pts',(0.00333734423875804,-0.0330013377137258,
-0.0118285093866645));
#40329=CARTESIAN_POINT('Ctrl Pts',(0.00209763410547778,-0.0328423166157698,
-0.0147946402144062));
#40330=CARTESIAN_POINT('Ctrl Pts',(-0.00106758966394507,-0.0326832955178137,
-0.0153568170849966));
#40331=CARTESIAN_POINT('Ctrl Pts',(-0.00325282526782655,-0.0325242744198576,
-0.0129989098283113));
#40332=CARTESIAN_POINT('Ctrl Pts',(-0.00245201090409445,-0.0323652533219015,
-0.00988546397148232));
#40333=CARTESIAN_POINT('Ctrl Pts',(0.000599691214404787,-0.0322062322239454,
-0.00887454488366325));
#40334=CARTESIAN_POINT('Ctrl Pts',(0.00310089382451873,-0.0320472111259893,
-0.0108941655010505));
#40335=CARTESIAN_POINT('Ctrl Pts',(0.00275553388456782,-0.0318881900280332,
-0.0140903487735019));
#40336=CARTESIAN_POINT('Ctrl Pts',(-0.000119351261976234,-0.0317291689300771,
-0.0155290636196804));
#40337=CARTESIAN_POINT('Ctrl Pts',(-0.00288467425340072,-0.0315701478321211,
-0.0138895960940694));
#40338=CARTESIAN_POINT('Ctrl Pts',(-0.00300192377299798,-0.031411126734165,
-0.0106769471015127));
#40339=CARTESIAN_POINT('Ctrl Pts',(-0.000363463202558005,-0.0312521056362089,
-0.00884026320022485));
#40340=CARTESIAN_POINT('Ctrl Pts',(0.00260864397039946,-0.0310930845382528,
-0.0100655885344216));
#40341=CARTESIAN_POINT('Ctrl Pts',(0.00318607768535292,-0.0309340634402968,
-0.013228090558674));
#40342=CARTESIAN_POINT('Ctrl Pts',(0.000838733661705831,-0.0307750423423407,
-0.0154246691050157));
#40343=CARTESIAN_POINT('Ctrl Pts',(-0.00227851175642546,-0.0306160212443846,
-0.0146388794719168));
#40344=CARTESIAN_POINT('Ctrl Pts',(-0.0033042041374851,-0.0304570001464284,
-0.01159211587077));
#40345=CARTESIAN_POINT('Ctrl Pts',(-0.00129655539127476,-0.0302979790484724,
-0.00908114284765269));
#40346=CARTESIAN_POINT('Ctrl Pts',(0.00190102515205851,-0.0301389579505163,
-0.0094111858675825));
#40347=CARTESIAN_POINT('Ctrl Pts',(0.00335404044265945,-0.0299799368525602,
-0.0122788856106888));
#40348=CARTESIAN_POINT('Ctrl Pts',(0.00172707811420276,-0.0298209157546041,
-0.0150524912685583));
#40349=CARTESIAN_POINT('Ctrl Pts',(-0.00148332063266471,-0.029661894656648,
-0.0151844611804898));
#40350=CARTESIAN_POINT('Ctrl Pts',(-0.0033359051396361,-0.0295028735586919,
-0.0125564131203294));
#40351=CARTESIAN_POINT('Ctrl Pts',(-0.00211844478601719,-0.0293438414855596,
-0.00957508346995853));
#40352=CARTESIAN_POINT('Ctrl Pts',(-2.15129732174238E-5,-0.0292378164450794,
-0.00918534259310061));
#40353=CARTESIAN_POINT('Ctrl Pts',(0.000877327784425402,-0.0291847984372511,
-0.00947761548516741));
#40354=CARTESIAN_POINT('Ctrl Pts',(-0.00064218188127976,-0.0341751246985829,
-0.00958749652954282));
#40355=CARTESIAN_POINT('Ctrl Pts',(0.000220042081112754,-0.0341221075628275,
-0.00937356148392917));
#40356=CARTESIAN_POINT('Ctrl Pts',(0.00215993841024188,-0.03401608339442,
-0.00987909587955745));
#40357=CARTESIAN_POINT('Ctrl Pts',(0.00310212958626195,-0.0338570521933608,
-0.0127555669433291));
#40358=CARTESIAN_POINT('Ctrl Pts',(0.00118962939453071,-0.0336980310954046,
-0.0150956808047299));
#40359=CARTESIAN_POINT('Ctrl Pts',(-0.00181144434149887,-0.0335390099974485,
-0.0147574182954002));
#40360=CARTESIAN_POINT('Ctrl Pts',(-0.00315144827747508,-0.0333799888994924,
-0.0120483170472104));
#40361=CARTESIAN_POINT('Ctrl Pts',(-0.00159754740617219,-0.0332209678015363,
-0.00945681779721357));
#40362=CARTESIAN_POINT('Ctrl Pts',(0.00142238269106645,-0.0330619467035802,
-0.00936106591288119));
#40363=CARTESIAN_POINT('Ctrl Pts',(0.00313684761337623,-0.0329029256056242,
-0.0118493766615973));
#40364=CARTESIAN_POINT('Ctrl Pts',(0.00197161517265394,-0.032743904507668,
-0.0146373121403257));
#40365=CARTESIAN_POINT('Ctrl Pts',(-0.00100345240101975,-0.032584883409712,
-0.0151657152802616));
#40366=CARTESIAN_POINT('Ctrl Pts',(-0.00305740626322348,-0.0324258623117559,
-0.0129494633081701));
#40367=CARTESIAN_POINT('Ctrl Pts',(-0.00230470218299792,-0.0322668412137998,
-0.0100230630010191));
#40368=CARTESIAN_POINT('Ctrl Pts',(0.000563663745807771,-0.0321078201158437,
-0.00907287659497971));
#40369=CARTESIAN_POINT('Ctrl Pts',(0.00291460235950802,-0.0319487990178876,
-0.0109711650723872));
#40370=CARTESIAN_POINT('Ctrl Pts',(0.00258999050472557,-0.0317897779199315,
-0.0139753322043438));
#40371=CARTESIAN_POINT('Ctrl Pts',(-0.000112181032131976,-0.0316307568219755,
-0.0153276138117228));
#40372=CARTESIAN_POINT('Ctrl Pts',(-0.00271137254648784,-0.0314717357240193,
-0.0137866400832125));
#40373=CARTESIAN_POINT('Ctrl Pts',(-0.00282157810198519,-0.0313127146260633,
-0.0107669964372615));
#40374=CARTESIAN_POINT('Ctrl Pts',(-0.000341627533130492,-0.0311536935281072,
-0.00904065444191939));
#40375=CARTESIAN_POINT('Ctrl Pts',(0.00245192525172084,-0.0309946724301511,
-0.0101923662748032));
#40376=CARTESIAN_POINT('Ctrl Pts',(0.00299466865517291,-0.030835651332195,
-0.0131648756167719));
#40377=CARTESIAN_POINT('Ctrl Pts',(0.000788345311947609,-0.0306766302342389,
-0.0152294909748955));
#40378=CARTESIAN_POINT('Ctrl Pts',(-0.0021416262914049,-0.0305176091362828,
-0.014490908989083));
#40379=CARTESIAN_POINT('Ctrl Pts',(-0.0031056984599932,-0.0303585880383268,
-0.0116271848878091));
#40380=CARTESIAN_POINT('Ctrl Pts',(-0.00121866262326115,-0.0301995669403707,
-0.00926706283526693));
#40381=CARTESIAN_POINT('Ctrl Pts',(0.00178681783615527,-0.0300405458424146,
-0.00957727796002242));
#40382=CARTESIAN_POINT('Ctrl Pts',(0.00315254076446096,-0.0298815247444585,
-0.012272695768762));
#40383=CARTESIAN_POINT('Ctrl Pts',(0.00162332096213945,-0.0297225036465024,
-0.0148796723543037));
#40384=CARTESIAN_POINT('Ctrl Pts',(-0.00139420762545537,-0.0295634825485463,
-0.0150037139495554));
#40385=CARTESIAN_POINT('Ctrl Pts',(-0.00313549497057911,-0.0294044614505902,
-0.012533550341734));
#40386=CARTESIAN_POINT('Ctrl Pts',(-0.00199117561620204,-0.0292454293774579,
-0.00973132913546924));
#40387=CARTESIAN_POINT('Ctrl Pts',(-2.02205448002642E-5,-0.0291394043369777,
-0.00936500260396888));
#40388=CARTESIAN_POINT('Ctrl Pts',(0.000824620827172333,-0.0290863863291494,
-0.00963971670546519));
#40389=CARTESIAN_POINT('Ctrl Pts',(-0.000601135800644895,-0.0340767125904812,
-0.00975293548579074));
#40390=CARTESIAN_POINT('Ctrl Pts',(0.000205977740047228,-0.0340236954547259,
-0.00955267444031453));
#40391=CARTESIAN_POINT('Ctrl Pts',(0.00202188249689775,-0.0339176712863184,
-0.0100258967976067));
#40392=CARTESIAN_POINT('Ctrl Pts',(0.00290385201903478,-0.033758640085259,
-0.012718513619038));
#40393=CARTESIAN_POINT('Ctrl Pts',(0.00111359233170327,-0.033599618987303,
-0.0149090553653577));
#40394=CARTESIAN_POINT('Ctrl Pts',(-0.00169566298317314,-0.0334405978893469,
-0.0145924134445845));
#40395=CARTESIAN_POINT('Ctrl Pts',(-0.00295001842732721,-0.0332815767913908,
-0.0120564687296492));
#40396=CARTESIAN_POINT('Ctrl Pts',(-0.00149543761210405,-0.0331225556934346,
-0.00963060929335837));
#40397=CARTESIAN_POINT('Ctrl Pts',(0.00133146882953737,-0.0329635345954786,
-0.009540977543648));
#40398=CARTESIAN_POINT('Ctrl Pts',(0.00293635098799442,-0.0328045134975225,
-0.0118702439365301));
#40399=CARTESIAN_POINT('Ctrl Pts',(0.0018455962398301,-0.0326454923995664,
-0.0144799840662451));
#40400=CARTESIAN_POINT('Ctrl Pts',(-0.000939315138094445,-0.0324864713016103,
-0.0149746134755266));
#40401=CARTESIAN_POINT('Ctrl Pts',(-0.0028619872586204,-0.0323274502036543,
-0.0129000167880288));
#40402=CARTESIAN_POINT('Ctrl Pts',(-0.00215739346190139,-0.0321684291056982,
-0.0101606620305559));
#40403=CARTESIAN_POINT('Ctrl Pts',(0.000527636277210757,-0.0320094080077421,
-0.00927120830629617));
#40404=CARTESIAN_POINT('Ctrl Pts',(0.00272831089449731,-0.031850386909786,
-0.0110481646437239));
#40405=CARTESIAN_POINT('Ctrl Pts',(0.00242444712488331,-0.0316913658118299,
-0.013860315635186));
#40406=CARTESIAN_POINT('Ctrl Pts',(-0.000105010802287719,-0.0315323447138738,
-0.0151261640037651));
#40407=CARTESIAN_POINT('Ctrl Pts',(-0.00253807083957495,-0.0313733236159177,
-0.0136836840723558));
#40408=CARTESIAN_POINT('Ctrl Pts',(-0.00264123243097238,-0.0312143025179616,
-0.0108570457730104));
#40409=CARTESIAN_POINT('Ctrl Pts',(-0.000319791863702978,-0.0310552814200056,
-0.00924104568361391));
#40410=CARTESIAN_POINT('Ctrl Pts',(0.00229520653304219,-0.0308962603220495,
-0.0103191440151849));
#40411=CARTESIAN_POINT('Ctrl Pts',(0.00280325962499289,-0.0307372392240933,
-0.0131016606748699));
#40412=CARTESIAN_POINT('Ctrl Pts',(0.000737956962189381,-0.0305782181261372,
-0.0150343128447755));
#40413=CARTESIAN_POINT('Ctrl Pts',(-0.00200474082638433,-0.0304191970281811,
-0.0143429385062493));
#40414=CARTESIAN_POINT('Ctrl Pts',(-0.0029071927825013,-0.0302601759302251,
-0.0116622539048482));
#40415=CARTESIAN_POINT('Ctrl Pts',(-0.00114076985524752,-0.030101154832269,
-0.00945298282288118));
#40416=CARTESIAN_POINT('Ctrl Pts',(0.00167261052025204,-0.0299421337343129,
-0.00974337005246235));
#40417=CARTESIAN_POINT('Ctrl Pts',(0.00295104108626248,-0.0297831126363568,
-0.012266505926835));
#40418=CARTESIAN_POINT('Ctrl Pts',(0.00151956381007614,-0.0296240915384008,
-0.014706853440049));
#40419=CARTESIAN_POINT('Ctrl Pts',(-0.00130509461824602,-0.0294650704404447,
-0.014822966718621));
#40420=CARTESIAN_POINT('Ctrl Pts',(-0.00293508480152213,-0.0293060493424886,
-0.0125106875631388));
#40421=CARTESIAN_POINT('Ctrl Pts',(-0.00186390644638689,-0.0291470172693563,
-0.00988757480097995));
#40422=CARTESIAN_POINT('Ctrl Pts',(-1.89281163831043E-5,-0.029040992228876,
-0.00954466261483715));
#40423=CARTESIAN_POINT('Ctrl Pts',(0.000771913869919264,-0.0289879742210478,
-0.00980181792576297));
#40424=CARTESIAN_POINT('Ctrl Pts',(-0.00249512019792405,-0.029278774389874,
-0.0120001969329541));
#40425=CARTESIAN_POINT('Ctrl Pts',(-0.00250451942578934,-0.0292787743898746,
-0.0116746048596339));
#40426=CARTESIAN_POINT('Ctrl Pts',(-0.00244956820908934,-0.029278774389875,
-0.0113485528346615));
#40427=CARTESIAN_POINT('Ctrl Pts',(-0.00233887355507737,-0.0292787743898753,
-0.0110396898663454));
#40428=CARTESIAN_POINT('Ctrl Pts',(-0.0023342889065707,-0.0292787743898753,
-0.011026897666405));
#40429=CARTESIAN_POINT('Ctrl Pts',(-0.00232960758938224,-0.0292787743898754,
-0.0110141358510404));
#40430=CARTESIAN_POINT('Ctrl Pts',(-0.00232483460901268,-0.0292787743898754,
-0.0110014176248355));
#40431=CARTESIAN_POINT('Ctrl Pts',(-0.00222580382029312,-0.0292787743898756,
-0.0107375372241906));
#40432=CARTESIAN_POINT('Ctrl Pts',(-0.00208719432964695,-0.0292787743898758,
-0.0104910173381353));
#40433=CARTESIAN_POINT('Ctrl Pts',(-0.00191326911752999,-0.0292787743898759,
-0.0102724976348523));
#40434=CARTESIAN_POINT('Ctrl Pts',(-0.00189637749193036,-0.0292787743898759,
-0.0102512749899633));
#40435=CARTESIAN_POINT('Ctrl Pts',(-0.00187914941593776,-0.0292787743898759,
-0.0102303172981295));
#40436=CARTESIAN_POINT('Ctrl Pts',(-0.00186158669131192,-0.0292787743898759,
-0.0102096351284549));
#40437=CARTESIAN_POINT('Ctrl Pts',(-0.00184648594129761,-0.0292787743898759,
-0.01019185222286));
#40438=CARTESIAN_POINT('Ctrl Pts',(-0.00183113778395428,-0.0292787743898759,
-0.010174273010336));
#40439=CARTESIAN_POINT('Ctrl Pts',(-0.00181554315970928,-0.0292787743898759,
-0.0101569043754393));
#40440=CARTESIAN_POINT('Ctrl Pts',(-0.00180724793405888,-0.0292787743898759,
-0.0101476655028994));
#40441=CARTESIAN_POINT('Ctrl Pts',(-0.00179888407649718,-0.0292787743898759,
-0.0101384875200101));
#40442=CARTESIAN_POINT('Ctrl Pts',(-0.00179045824703803,-0.0292787743898759,
-0.0101293782351649));
#40443=CARTESIAN_POINT('Ctrl Pts',(-0.00176932982413912,-0.0292787743898759,
-0.0101065359947126));
#40444=CARTESIAN_POINT('Ctrl Pts',(-0.00174780084142207,-0.0292787743898759,
-0.0100841134776088));
#40445=CARTESIAN_POINT('Ctrl Pts',(-0.0017258778551185,-0.0292787743898759,
-0.0100621241575538));
#40446=CARTESIAN_POINT('Ctrl Pts',(-0.00129914862071067,-0.029278774389876,
-0.00963410374179902));
#40447=CARTESIAN_POINT('Ctrl Pts',(-0.00072150280878173,-0.0292787743898755,
-0.00936613739934554));
#40448=CARTESIAN_POINT('Ctrl Pts',(-0.000116750728983814,-0.0292787743898747,
-0.00928163047214553));
#40449=CARTESIAN_POINT('Ctrl Pts',(-9.8096741933677E-5,-0.0292787743898747,
-0.00927902379880236));
#40450=CARTESIAN_POINT('Ctrl Pts',(-7.94118191834939E-5,-0.0292787743898746,
-0.00927659177262819));
#40451=CARTESIAN_POINT('Ctrl Pts',(-6.06985211378466E-5,-0.0292787743898746,
-0.00927433533713099));
#40452=CARTESIAN_POINT('Ctrl Pts',(-4.47341024448895E-5,-0.0292787743898746,
-0.00927241035945239));
#40453=CARTESIAN_POINT('Ctrl Pts',(-2.87488940363722E-5,-0.0292787743898746,
-0.00927061324069165));
#40454=CARTESIAN_POINT('Ctrl Pts',(-1.27594804140441E-5,-0.0292787743898745,
-0.0092689459349433));
#40455=CARTESIAN_POINT('Ctrl Pts',(8.69557107774587E-5,-0.0292787743898736,
-0.00925854807324565));
#40456=CARTESIAN_POINT('Ctrl Pts',(0.000186975259284375,-0.029278774389874,
-0.00925317714695822));
#40457=CARTESIAN_POINT('Ctrl Pts',(0.000286891956576391,-0.0292787743898741,
-0.00925288394665933));
#40458=CARTESIAN_POINT('Ctrl Pts',(0.000484391186557055,-0.0292787743898744,
-0.00925230439554493));
#40459=CARTESIAN_POINT('Ctrl Pts',(0.000681486279184165,-0.0292787743898747,
-0.00927151228708075));
#40460=CARTESIAN_POINT('Ctrl Pts',(0.000875206702308309,-0.0292787743898749,
-0.0093114725913186));
#40461=CARTESIAN_POINT('Ctrl Pts',(0.000892515753144813,-0.0292787743898749,
-0.00931504307153096));
#40462=CARTESIAN_POINT('Ctrl Pts',(0.000909797888585897,-0.029278774389875,
-0.00931877977997034));
#40463=CARTESIAN_POINT('Ctrl Pts',(0.000927050983124846,-0.0292787743898723,
-0.00932268373767265));
#40464=CARTESIAN_POINT('Origin',(0.,-0.0292787743898723,-0.0121758532865581));
#40465=CARTESIAN_POINT('',(0.001475,-0.0292787743898623,-0.0121758532865581));
#40466=CARTESIAN_POINT('Origin',(0.,-0.0292787743898623,-0.0121758532865581));
#40467=CARTESIAN_POINT('Origin',(0.,-0.0341787743898723,-0.0121758532865581));
#40468=CARTESIAN_POINT('',(-0.0029,-0.0341787743898723,-0.0121758532865581));
#40469=CARTESIAN_POINT('Origin',(0.,-0.0271787743898723,-0.0121758532865581));
#40470=CARTESIAN_POINT('',(0.001475,-0.0271787743898623,-0.0121758532865581));
#40471=CARTESIAN_POINT('Origin',(0.,-0.0271787743898623,-0.0121758532865581));
#40472=CARTESIAN_POINT('Origin',(0.,-0.0292787743898723,-0.0121758532865581));
#40473=CARTESIAN_POINT('',(0.001475,-0.0292787743898723,-0.0121758532865581));
#50050=UNCERTAINTY_MEASURE_WITH_UNIT(LENGTH_MEASURE(1.E-5),#50082,
'DISTANCE_ACCURACY_VALUE',
'Maximum model space distance between geometric entities at asserted c
onnectivities');
#50059=UNCERTAINTY_MEASURE_WITH_UNIT(LENGTH_MEASURE(1.E-5),#50082,
'DISTANCE_ACCURACY_VALUE',
'Maximum model space distance between geometric entities at asserted c
onnectivities');
#50072=(
GEOMETRIC_REPRESENTATION_CONTEXT(3)
GLOBAL_UNCERTAINTY_ASSIGNED_CONTEXT((#50050))
GLOBAL_UNIT_ASSIGNED_CONTEXT((#50082,#50083,#50084))
REPRESENTATION_CONTEXT('','3D')
);
#50081=(
GEOMETRIC_REPRESENTATION_CONTEXT(3)
GLOBAL_UNCERTAINTY_ASSIGNED_CONTEXT((#50059))
GLOBAL_UNIT_ASSIGNED_CONTEXT((#50082,#50083,#50084))
REPRESENTATION_CONTEXT('','3D')
);
#50082=(
LENGTH_UNIT()
NAMED_UNIT(*)
SI_UNIT($,.METRE.)
);
#50083=(
NAMED_UNIT(*)
PLANE_ANGLE_UNIT()
SI_UNIT($,.RADIAN.)
);
#50084=(
NAMED_UNIT(*)
SI_UNIT($,.STERADIAN.)
SOLID_ANGLE_UNIT()
);
#50097=SHAPE_DEFINITION_REPRESENTATION(#50118,#50159);
#50118=PRODUCT_DEFINITION_SHAPE('',$,#50181);
#50159=SHAPE_REPRESENTATION('',(#10620),#50072);
#50168=PRODUCT_DEFINITION_CONTEXT('part definition',#50233,'design');
#50181=PRODUCT_DEFINITION('Filament Thermal Heatbreak Throat',
'Filament Thermal Heatbreak Throat',#50202,#50168);
#50202=PRODUCT_DEFINITION_FORMATION('',$,#50247);
#50233=APPLICATION_CONTEXT('Managed model based 3d engineering');
#50234=PRODUCT_CONTEXT('part definition',#50233,'mechanical');
#50247=PRODUCT('Filament Thermal Heatbreak Throat',
'Filament Thermal Heatbreak Throat',
'LEGAL AND USAGE DISCLAIMER: this Data/Model is provided \X2\201C\X0\A
S IS\X2\201D\X0\ for informational and representational only. It is a 
geometric approximation and is NOT engineered, certified, or guarantee
d for dimensional accuracy, exact tolerances, or production-level prec
ision. Vendor disclaims all implied warranties including fitness for a
 particular purpose. DO NOT USE FOR DIRECT PHYSICAL MANUFACTURING, AUT
OMATED PRODUCTION, OR SAFETY-CRITICAL SYSTEMS without independent engi
neering verification and resolution of any design discrepancies.',(#50234));
#50261=PRESENTATION_STYLE_ASSIGNMENT((#50268));
#50268=SURFACE_STYLE_USAGE(.BOTH.,#50275);
#50275=SURFACE_SIDE_STYLE('',(#50282));
#50282=SURFACE_STYLE_FILL_AREA(#50289);
#50289=FILL_AREA_STYLE('Opaque(179,179,179)',(#50296));
#50296=FILL_AREA_STYLE_COLOUR('Opaque(179,179,179)',#50303);
#50303=COLOUR_RGB('Opaque(179,179,179)',0.701960784313725,0.701960784313725,
0.701960784313725);
ENDSEC;
END-ISO-10303-21;
